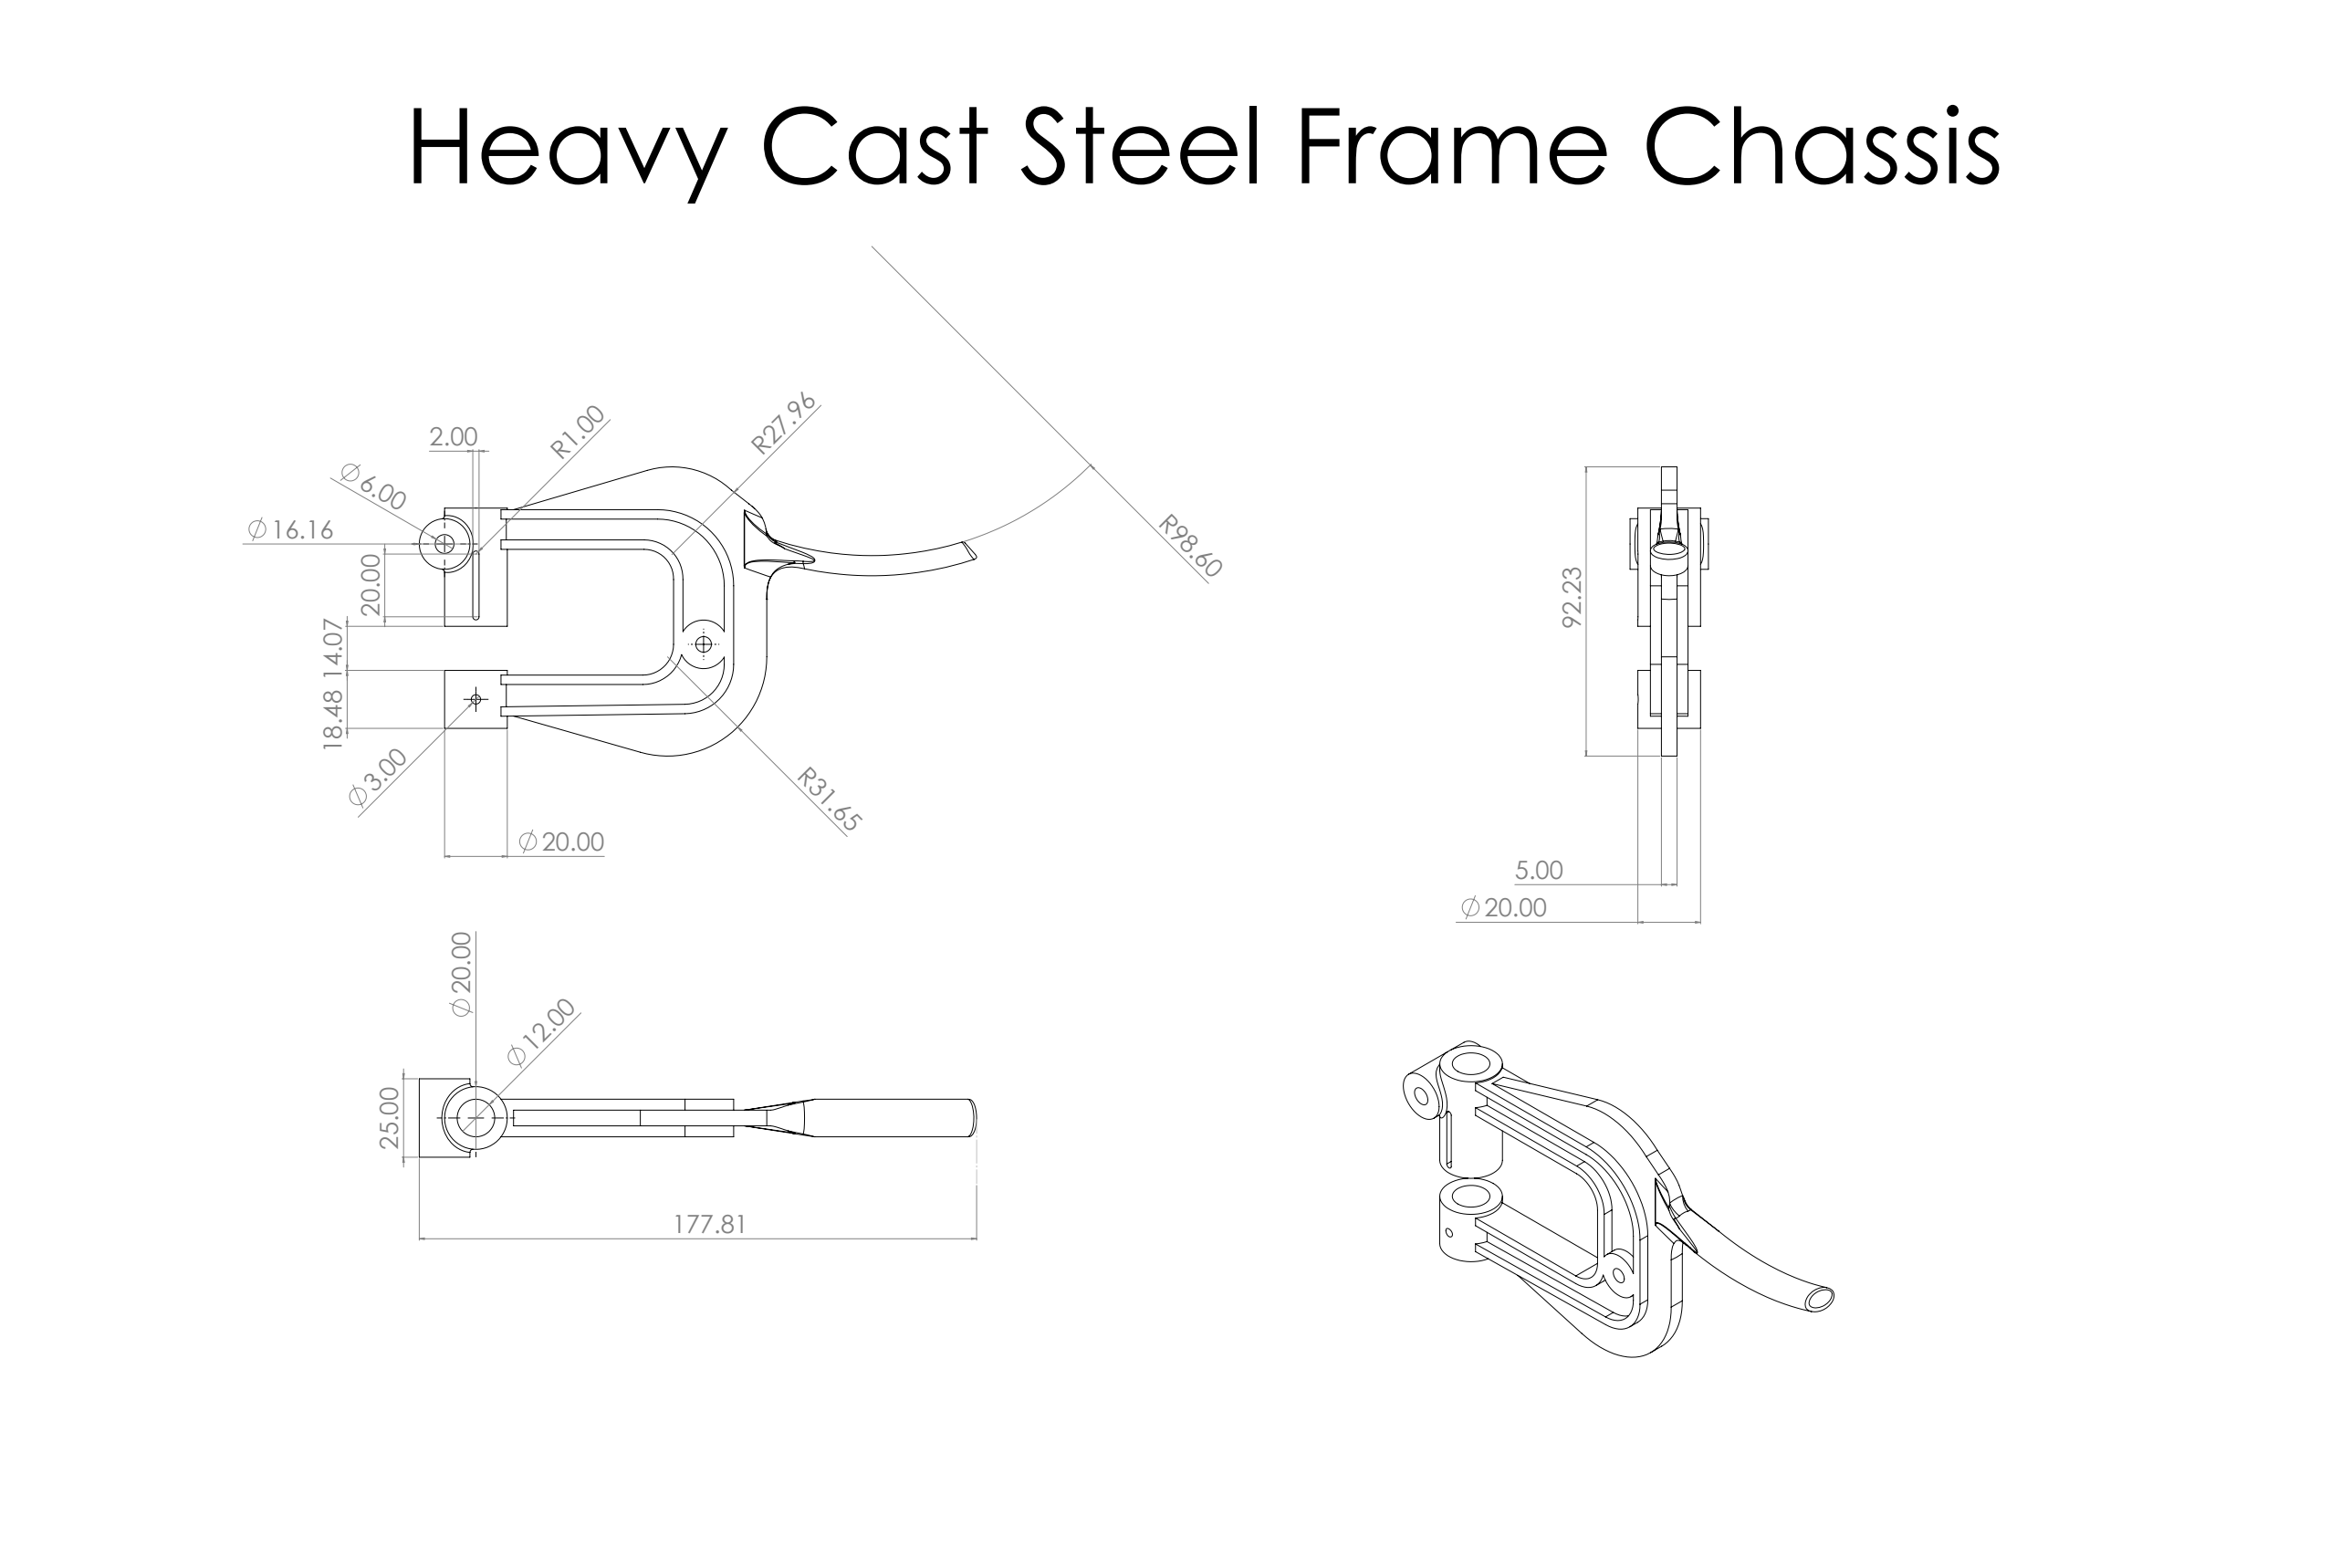
ISO-10303-21;
HEADER;
FILE_DESCRIPTION (('STEP AP214'),
    '1' );
FILE_NAME ('Heavy Cast Steel Frame Chassis.step',
    '2026-10-24T22:54:28',
    ( '' ),
    ( '' ),
    'SwSTEP 2.0',
    'SolidWorks 2025',
    '' );
FILE_SCHEMA (( 'AUTOMOTIVE_DESIGN' ));
ENDSEC;

DATA;
#3=CARTESIAN_POINT ( 'NONE',  ( 35.84136525188217348, -3.161327592290550825, 5.800309892887216989 ) ) ;
#5=CARTESIAN_POINT ( 'NONE',  ( 21.85645829928708039, 3.222455659797274663, 4.920547929353077166 ) ) ;
#7=VERTEX_POINT ( 'NONE', #10173 ) ;
#8=AXIS2_PLACEMENT_3D ( 'NONE', #5733, #22003, #2874 ) ;
#12=CARTESIAN_POINT ( 'NONE',  ( -71.92837670882107659, -20.78299143688747819, 38.00000000000000711 ) ) ;
#18=ORIENTED_EDGE ( 'NONE', *, *, #8070, .F. ) ;
#19=CARTESIAN_POINT ( 'NONE',  ( 21.85695786933250062, 3.618345527896555058, -4.619311229777957273 ) ) ;
#21=CARTESIAN_POINT ( 'NONE',  ( 21.85643539959774273, 10.54442680926682208, -0.8960936389291185300 ) ) ;
#28=CARTESIAN_POINT ( 'NONE',  ( 84.98726364908050357, 2.895996327189970021, 0.3032432708941606436 ) ) ;
#33=CARTESIAN_POINT ( 'NONE',  ( 15.61026443024166888, -3.737113800699907618, 2.632854455050967157 ) ) ;
#35=CARTESIAN_POINT ( 'NONE',  ( 34.13602976376383680, -3.136024335859604495, -5.534151046271431618 ) ) ;
#42=ORIENTED_EDGE ( 'NONE', *, *, #27798, .T. ) ;
#43=CARTESIAN_POINT ( 'NONE',  ( 37.00808470818950013, -3.245065655003315896, 5.947274188226997715 ) ) ;
#46=CARTESIAN_POINT ( 'NONE',  ( 87.70627581785944926, -2.246752060737267964, -2.595469083058261184 ) ) ;
#50=CARTESIAN_POINT ( 'NONE',  ( -70.92837670882107659, -23.80776546975053520, 0.000000000000000000 ) ) ;
#55=CARTESIAN_POINT ( 'NONE',  ( 24.04452188815935898, 3.332949059894338983, 3.268005727657652404 ) ) ;
#62=CARTESIAN_POINT ( 'NONE',  ( -71.02647992656017095, -45.61702805680359774, 6.000000000000006217 ) ) ;
#64=CARTESIAN_POINT ( 'NONE',  ( 17.44489164598297748, 8.923283497490654526, -2.906184072486747816 ) ) ;
#74=CARTESIAN_POINT ( 'NONE',  ( 27.93970670347097851, 2.313158937601060838, 2.612756796560576689 ) ) ;
#75=ADVANCED_FACE ( 'NONE', ( #21079, #21280 ), #17552, .T. ) ;
#78=CARTESIAN_POINT ( 'NONE',  ( 21.32819773538203734, -0.9284710762945487250, 4.803740791084685213 ) ) ;
#81=DIRECTION ( 'NONE',  ( -0.000000000000000000, -0.000000000000000000, -1.000000000000000000 ) ) ;
#86=CARTESIAN_POINT ( 'NONE',  ( 33.43749314767592296, -3.587398716883661631, -5.336340041065867901 ) ) ;
#90=CARTESIAN_POINT ( 'NONE',  ( 87.15505355144220800, 0.4610318193416703680, -5.246243280819175681 ) ) ;
#91=CARTESIAN_POINT ( 'NONE',  ( 23.06594672544511582, -8.086844732617873177, 2.500000000000001332 ) ) ;
#99=CARTESIAN_POINT ( 'NONE',  ( 8.290806648384990041, -33.63722727088462250, 6.000000000000001776 ) ) ;
#105=CARTESIAN_POINT ( 'NONE',  ( 24.41733686895641853, 3.169751135957838084, 3.243633740826553424 ) ) ;
#111=CARTESIAN_POINT ( 'NONE',  ( 23.09356329134889663, 0.3660385851480518205, 5.918987391801470821 ) ) ;
#117=EDGE_CURVE ( 'NONE', #23904, #23738, #12152, .T. ) ;
#120=CARTESIAN_POINT ( 'NONE',  ( 21.85643539959779602, 4.838159542671753854, -10.55000746994157979 ) ) ;
#122=CARTESIAN_POINT ( 'NONE',  ( -73.76321677170048474, 8.370041474172571938, 9.593160009199120708 ) ) ;
#123=CARTESIAN_POINT ( 'NONE',  ( 37.18496992949054913, -2.918767381260244154, 5.998331359843706245 ) ) ;
#127=CARTESIAN_POINT ( 'NONE',  ( -80.34626650618338317, 10.54088118240301775, -3.386839445737261034 ) ) ;
#128=CARTESIAN_POINT ( 'NONE',  ( 28.64320648638592104, -3.206774183960824587, -4.676863129512683237 ) ) ;
#129=CARTESIAN_POINT ( 'NONE',  ( 37.18689723876565978, -2.963747097358016003, -6.000011646107364705 ) ) ;
#130=CARTESIAN_POINT ( 'NONE',  ( -4.890026461918814071, -8.228598103685714525E-16, 6.000000000000000000 ) ) ;
#131=SHAPE_REPRESENTATION ( 'Heavy Cast Steel Frame Chassis', ( #30744 ), #7710 ) ;
#132=CARTESIAN_POINT ( 'NONE',  ( 21.48907598089328630, 5.617352746613489600, 3.514627525551620391 ) ) ;
#134=DIRECTION ( 'NONE',  ( 7.826543628040252284E-17, -1.000000000000000000, 0.000000000000000000 ) ) ;
#135=DIRECTION ( 'NONE',  ( 0.000000000000000000, 0.000000000000000000, -1.000000000000000000 ) ) ;
#137=CARTESIAN_POINT ( 'NONE',  ( 21.75356392267549310, 0.6818289899092313533, -8.045969637709488254 ) ) ;
#139=CARTESIAN_POINT ( 'NONE',  ( 32.63483486068848549, -3.790703822822770075, -4.926795467402606654 ) ) ;
#140=CARTESIAN_POINT ( 'NONE',  ( 25.39710067966193918, 2.282707499838438459, -4.082506721808119465 ) ) ;
#141=VERTEX_POINT ( 'NONE', #15910 ) ;
#144=CARTESIAN_POINT ( 'NONE',  ( 35.79015163951060430, -3.279169341215469213, 5.792316770070685017 ) ) ;
#146=CARTESIAN_POINT ( 'NONE',  ( 87.19696342060086636, -0.1553247823698818142, -5.755373573531420206 ) ) ;
#148=DIRECTION ( 'NONE',  ( 0.000000000000000000, 1.000000000000000000, 0.000000000000000000 ) ) ;
#150=CARTESIAN_POINT ( 'NONE',  ( 24.34527755301806451, 2.925195485058063927, 3.749207160500627634 ) ) ;
#163=CARTESIAN_POINT ( 'NONE',  ( -71.80187163192030653, -21.28714814314140469, 9.961904852117910991 ) ) ;
#165=CARTESIAN_POINT ( 'NONE',  ( 22.18865037645032601, 5.257466153314783064, -3.084642082178049360 ) ) ;
#173=CARTESIAN_POINT ( 'NONE',  ( -80.59724102483603758, -5.646254625739555166, -5.338710406051827562 ) ) ;
#176=CARTESIAN_POINT ( 'NONE',  ( 87.91343731185466481, -2.496140582104141359, -0.8634702502314072214 ) ) ;
#178=ORIENTED_EDGE ( 'NONE', *, *, #20772, .F. ) ;
#184=ORIENTED_EDGE ( 'NONE', *, *, #32019, .F. ) ;
#185=CARTESIAN_POINT ( 'NONE',  ( 35.86808974331964350, -2.088826501973227057, 5.804480896110276511 ) ) ;
#187=CARTESIAN_POINT ( 'NONE',  ( 87.73528170195316989, -0.1907079786014589107, -4.255344914058586170 ) ) ;
#191=DIRECTION ( 'NONE',  ( 1.000000000000000000, 0.000000000000000000, 0.000000000000000000 ) ) ;
#193=ORIENTED_EDGE ( 'NONE', *, *, #36678, .T. ) ;
#195=ORIENTED_EDGE ( 'NONE', *, *, #21675, .F. ) ;
#196=CARTESIAN_POINT ( 'NONE',  ( -72.40112826922974421, 5.951953399866846794, 9.891857903246553008 ) ) ;
#199=CARTESIAN_POINT ( 'NONE',  ( 21.94883752246645514, 5.596572238070317340, 3.078924485188955895 ) ) ;
#200=CARTESIAN_POINT ( 'NONE',  ( 25.44397797946202289, 1.878947632829091274, 4.230557655479292301 ) ) ;
#201=CARTESIAN_POINT ( 'NONE',  ( 27.23730700677205618, 2.045195204592743288, 3.801859922671973369 ) ) ;
#206=CARTESIAN_POINT ( 'NONE',  ( 85.45774792847294066, 2.367526054045318240, -2.907096912194419236 ) ) ;
#211=CARTESIAN_POINT ( 'NONE',  ( 23.22388547762907507, 3.341220446849921366, -3.796200845986580141 ) ) ;
#213=CARTESIAN_POINT ( 'NONE',  ( 21.85643539959774273, -10.14878426894149221, 9.991042268249278990 ) ) ;
#215=EDGE_CURVE ( 'NONE', #29684, #24175, #38700, .T. ) ;
#217=CARTESIAN_POINT ( 'NONE',  ( 88.07575545775937087, -0.5731442609823791390, 3.387043347726935050 ) ) ;
#218=VERTEX_POINT ( 'NONE', #31772 ) ;
#220=CARTESIAN_POINT ( 'NONE',  ( 14.77315594796442966, 13.19392823276588089, 2.499999999999996891 ) ) ;
#222=CARTESIAN_POINT ( 'NONE',  ( 26.28033317518049472, -2.868937434659071695, 4.308079602883402970 ) ) ;
#223=CARTESIAN_POINT ( 'NONE',  ( 33.68713372036676645, -3.101946962961664500, -5.464089962110080911 ) ) ;
#231=CARTESIAN_POINT ( 'NONE',  ( 31.99965334531182393, -3.138902966780172665, 5.200717837716557490 ) ) ;
#234=CARTESIAN_POINT ( 'NONE',  ( 20.91779494910925052, 4.579615739114438533, 2.660980063663031636 ) ) ;
#240=CARTESIAN_POINT ( 'NONE',  ( 87.52056228721085063, 0.05047505923521825727, -4.363535012332786955 ) ) ;
#248=CARTESIAN_POINT ( 'NONE',  ( 23.42285139394776650, 3.710806655037595547, 3.268438641518027765 ) ) ;
#250=EDGE_CURVE ( 'NONE', #11656, #22420, #37713, .T. ) ;
#255=CARTESIAN_POINT ( 'NONE',  ( -72.12756863348978698, -46.19478142241662511, 5.880635833492268816 ) ) ;
#257=CARTESIAN_POINT ( 'NONE',  ( 15.15950051851460145, 11.94258596470134215, -2.548869419651209611 ) ) ;
#262=VECTOR ( 'NONE', #5403, 1000.000000000000000 ) ;
#267=CARTESIAN_POINT ( 'NONE',  ( 17.02720445904918023, 12.19482440094239273, 2.500000000000000444 ) ) ;
#268=CARTESIAN_POINT ( 'NONE',  ( 31.47838864403340509, -3.170179483860372738, -5.357953045474171283 ) ) ;
#269=CARTESIAN_POINT ( 'NONE',  ( 0.000000000000000000, 0.000000000000000000, -2.500000000000000000 ) ) ;
#272=CIRCLE ( 'NONE', #25922, 10.00000000000000888 ) ;
#275=DIRECTION ( 'NONE',  ( -0.000000000000000000, -0.000000000000000000, 1.000000000000000000 ) ) ;
#277=CARTESIAN_POINT ( 'NONE',  ( 36.44537822125108306, -3.301946079842590365, -5.889618514196052423 ) ) ;
#280=CARTESIAN_POINT ( 'NONE',  ( 14.75904227071888108, -4.442295602227281037, -2.509903513768624972 ) ) ;
#286=CARTESIAN_POINT ( 'NONE',  ( 31.57897186779749887, -2.953369379551184171, 5.135060318927252787 ) ) ;
#290=B_SPLINE_CURVE_WITH_KNOTS ( 'NONE', 3,
 ( #31493, #201, #40324, #12739, #21411, #2492, #33986, #15014, #5760, #12117, #37245, #27977, #18300, #40525, #12334, #9037, #21615, #18711, #24908, #12538, #37442, #9240, #21817, #6170, #3114, #15632, #25110, #4461, #3513, #22239, #20275, #20084, #35749, #37849, #13504, #16983, #1375, #1769, #7523, #29956, #25318, #17182, #6583, #39002, #9654, #29158 ),
 .UNSPECIFIED., .F., .F.,
 ( 4, 2, 1, 1, 2, 2, 1, 1, 1, 2, 2, 2, 1, 1, 1, 2, 2, 1, 2, 2, 2, 2, 1, 1, 2, 2, 1, 2, 4 ),
 ( 0.1281237029900336166, 0.4747198910002122796, 0.4963821527508484044, 0.4990899354696787804, 0.4997668811493873875, 0.5004438268290958280, 0.5017977181885129312, 0.5072132836261800115, 0.5180444145015135060, 0.5613689380028479281, 0.6480179850055166613, 0.7346670320081853944, 0.7454981628835195551, 0.7482059456023534283, 0.7495598369617704204, 0.7498983098016249738, 0.7502367826414796381, 0.7509137283211883007, 0.7563292937588557141, 0.7779915555095239243, 0.7996538172601921346, 0.8104849481355265173, 0.8118388394949429543, 0.8121773123347969525, 0.8123465487547236741, 0.8125157851746505067, 0.8131927308543577260, 0.8159005135731869363, 0.8213160790108455789 ),
 .UNSPECIFIED. ) ;
#296=CARTESIAN_POINT ( 'NONE',  ( 23.06570227960076025, 3.126885040524279624, 4.061145912289076954 ) ) ;
#303=CARTESIAN_POINT ( 'NONE',  ( 23.43463349670878415, 3.790763441738238537, 3.110222249176512133 ) ) ;
#305=VECTOR ( 'NONE', #27454, 1000.000000000000000 ) ;
#311=CARTESIAN_POINT ( 'NONE',  ( 21.84880020533123002, 0.3448032378364013772, 8.036168467369821045 ) ) ;
#318=CARTESIAN_POINT ( 'NONE',  ( 22.67874324181232737, -4.030091496876125667, 7.802482278901700319 ) ) ;
#321=CARTESIAN_POINT ( 'NONE',  ( -75.51466614119452458, 10.05014096851642158, 8.892739820773797987 ) ) ;
#322=CARTESIAN_POINT ( 'NONE',  ( 21.96835285544658944, 0.2152711931543893065, -7.743667062754403752 ) ) ;
#323=ORIENTED_EDGE ( 'NONE', *, *, #28033, .F. ) ;
#327=FACE_OUTER_BOUND ( 'NONE', #20175, .T. ) ;
#328=CARTESIAN_POINT ( 'NONE',  ( 36.87196059928034941, -2.085890912122125407, -5.863601101037241747 ) ) ;
#338=CARTESIAN_POINT ( 'NONE',  ( 30.66378199172083896, -3.777849468416345502, -4.533872787636463286 ) ) ;
#343=DIRECTION ( 'NONE',  ( 0.7877517966954343809, -0.6159927814537400348, 0.000000000000000000 ) ) ;
#344=CARTESIAN_POINT ( 'NONE',  ( 88.38642666631945133, -2.374919807968325358, 0.2172961577596721761 ) ) ;
#348=CARTESIAN_POINT ( 'NONE',  ( 24.52494981597524770, 2.752700276650007716, 3.867455811991591386 ) ) ;
#364=ORIENTED_EDGE ( 'NONE', *, *, #24881, .F. ) ;
#370=CARTESIAN_POINT ( 'NONE',  ( 33.89815560913680059, -5.472034195326516581, 0.3552926572089393775 ) ) ;
#371=CARTESIAN_POINT ( 'NONE',  ( 22.19574982338894031, 5.228104102381771590, -3.102888934201143201 ) ) ;
#372=ORIENTED_EDGE ( 'NONE', *, *, #28540, .T. ) ;
#377=CARTESIAN_POINT ( 'NONE',  ( -81.11285676435983305, -5.649961960633484104, -4.124376956758348811 ) ) ;
#379=CARTESIAN_POINT ( 'NONE',  ( 29.20860690094596634, 2.240472738085125037, 1.050758983225395848 ) ) ;
#381=CARTESIAN_POINT ( 'NONE',  ( 87.68638643695580015, -2.222987235672965411, -2.753905389729575326 ) ) ;
#385=CARTESIAN_POINT ( 'NONE',  ( 24.97673583131591712, 3.396458356181121019, -1.647695864654638909 ) ) ;
#394=CARTESIAN_POINT ( 'NONE',  ( 21.25246165869702253, 3.318379160498120761, 3.523358653204108570 ) ) ;
#396=CARTESIAN_POINT ( 'NONE',  ( 86.26657670271889344, 1.459011185482768314, -4.895973709007312991 ) ) ;
#411=CARTESIAN_POINT ( 'NONE',  ( 23.70424450760806323, 1.818959193472196922, 4.681574839466135174 ) ) ;
#413=CIRCLE ( 'NONE', #30646, 12.38600677260393113 ) ;
#417=CARTESIAN_POINT ( 'NONE',  ( 85.87571968583984017, 1.898040338034475472, 4.108051227457266918 ) ) ;
#421=CARTESIAN_POINT ( 'NONE',  ( 22.18398091595247124, 4.302725770086238022, -3.814574538098304046 ) ) ;
#425=CARTESIAN_POINT ( 'NONE',  ( 21.85643539959775339, -6.841675198209371977, -12.88699694080538549 ) ) ;
#427=CARTESIAN_POINT ( 'NONE',  ( 53.63043182916395324, -5.819003020824450978, 6.000000000000000888 ) ) ;
#429=CARTESIAN_POINT ( 'NONE',  ( 85.06055580697953644, 2.762169973306998205, -2.784126402610546780 ) ) ;
#431=CARTESIAN_POINT ( 'NONE',  ( 14.69558838330753581, 12.33286846116140367, 2.499999999999996891 ) ) ;
#432=CARTESIAN_POINT ( 'NONE',  ( 14.98566736410303868, -6.090311521776418324, 2.529564007200721054 ) ) ;
#433=CARTESIAN_POINT ( 'NONE',  ( 33.62870426848748195, -1.228885055514358005, -5.454970633020429283 ) ) ;
#436=CARTESIAN_POINT ( 'NONE',  ( -74.18164544079856171, -2.036837289978346455, 10.73485733915913443 ) ) ;
#440=CARTESIAN_POINT ( 'NONE',  ( 33.46455574127770660, -3.089180930156425475, 5.429351285402141514 ) ) ;
#443=CARTESIAN_POINT ( 'NONE',  ( 36.13178710339454369, -1.532094116269871797, 5.644416983045655201 ) ) ;
#445=VECTOR ( 'NONE', #7320, 1000.000000000000000 ) ;
#448=VECTOR ( 'NONE', #1284, 1000.000000000000000 ) ;
#449=EDGE_CURVE ( 'NONE', #15211, #25138, #33471, .T. ) ;
#451=CARTESIAN_POINT ( 'NONE',  ( -80.82841455951717080, 11.46672392024627385, -1.471659699228122786 ) ) ;
#454=CARTESIAN_POINT ( 'NONE',  ( 8.290806648384990041, -10.90558813203967148, 6.000000000000000000 ) ) ;
#458=CARTESIAN_POINT ( 'NONE',  ( 22.03184786808944651, 5.415838924531075627, 3.191312399929147059 ) ) ;
#467=CARTESIAN_POINT ( 'NONE',  ( 19.96934150597399693, 6.745664378534328876, -3.285863046672279353 ) ) ;
#474=B_SPLINE_CURVE_WITH_KNOTS ( 'NONE', 3,
 ( #7514, #16768, #32255, #7119, #4054, #35545, #13493, #35147, #38993, #16570, #10598, #20074, #26464, #32851, #19480, #29350, #16376, #29150, #32651, #13092, #19682, #7315, #32054, #38600, #4451, #22979, #28950, #10792, #32446, #13285, #25857, #25653, #3860, #1170, #753, #1365 ),
 .UNSPECIFIED., .F., .F.,
 ( 4, 2, 2, 2, 2, 2, 2, 2, 2, 2, 2, 2, 2, 2, 2, 2, 2, 4 ),
 ( 0.07948797976893491601, 0.08078140541914788364, 0.08207483106936083739, 0.08336825671957380501, 0.08466168236978677264, 0.08595510801999974027, 0.08724853367021269401, 0.08854195932042566164, 0.08983538497063862927, 0.09112881062085158301, 0.09242223627106455064, 0.09371566192127751826, 0.09500908757149048589, 0.09630251322170343964, 0.09759593887191640726, 0.09888936452212937489, 0.09953607734723585176, 0.1001827901723423425 ),
 .UNSPECIFIED. ) ;
#478=CARTESIAN_POINT ( 'NONE',  ( 26.73479038929921359, 2.133517298515754668, 4.055905576634827092 ) ) ;
#490=CARTESIAN_POINT ( 'NONE',  ( 30.66842703005120185, 0.2949493320676357944, -4.962900476310909248 ) ) ;
#495=CARTESIAN_POINT ( 'NONE',  ( 22.49821043992852410, -9.358482552309803637, -2.500000000000000000 ) ) ;
#497=CARTESIAN_POINT ( 'NONE',  ( 21.89440445940014257, -12.98914838499760549, 2.499999999999999556 ) ) ;
#506=CARTESIAN_POINT ( 'NONE',  ( 30.31548945822549967, -3.037691172068890388, 4.938150023066174121 ) ) ;
#508=CARTESIAN_POINT ( 'NONE',  ( 21.85677098809243546, 3.668375465701176896, 4.582786065448858359 ) ) ;
#514=CARTESIAN_POINT ( 'NONE',  ( 24.40645114936911853, 3.164002126677583959, 3.269146773302918696 ) ) ;
#518=EDGE_LOOP ( 'NONE', ( #5397, #1910, #16353, #3651, #24693, #26966, #34035 ) ) ;
#520=CARTESIAN_POINT ( 'NONE',  ( 24.12512118317265930, 0.5285243960147255615, 5.092426130416875196 ) ) ;
#527=CARTESIAN_POINT ( 'NONE',  ( 24.99455384622441301, -2.608472216378299180, -6.027016329390949778 ) ) ;
#531=CARTESIAN_POINT ( 'NONE',  ( -72.64281072204887835, 6.529755665022496380, 9.854046603058758791 ) ) ;
#532=CARTESIAN_POINT ( 'NONE',  ( 20.40287464734031531, 10.75613383782063970, 2.500000000000000000 ) ) ;
#533=EDGE_LOOP ( 'NONE', ( #33702, #7118, #20763, #32067, #12346, #35016, #16297 ) ) ;
#537=CARTESIAN_POINT ( 'NONE',  ( 33.45805083109267741, -3.829395647111636602, -5.093820334410049000 ) ) ;
#538=CARTESIAN_POINT ( 'NONE',  ( 27.81621687972488033, 1.844493567162720948, -3.906584444767790654 ) ) ;
#540=CARTESIAN_POINT ( 'NONE',  ( 16.53760894254279634, 10.03315526601902619, 2.737223308667571242 ) ) ;
#541=CARTESIAN_POINT ( 'NONE',  ( 0.7201709579117279159, -51.60714625320436255, 6.000000000000000000 ) ) ;
#546=ADVANCED_FACE ( 'NONE', ( #1471 ), #22891, .T. ) ;
#548=CARTESIAN_POINT ( 'NONE',  ( 35.51269972589511070, -1.199312315519171834, -5.486990563529896114 ) ) ;
#553=CARTESIAN_POINT ( 'NONE',  ( 87.30284416890829391, -1.044652313481390760, -5.185858056390752147 ) ) ;
#556=ORIENTED_EDGE ( 'NONE', *, *, #29793, .F. ) ;
#557=CARTESIAN_POINT ( 'NONE',  ( 24.53045243809206255, 2.749270639064558708, 3.869256640630484689 ) ) ;
#559=DIRECTION ( 'NONE',  ( 0.000000000000000000, 1.000000000000000000, 0.000000000000000000 ) ) ;
#561=VERTEX_POINT ( 'NONE', #26383 ) ;
#564=ORIENTED_EDGE ( 'NONE', *, *, #36948, .F. ) ;
#575=CARTESIAN_POINT ( 'NONE',  ( 33.79783626363753513, -4.901490921675078383, -3.331131011404923736 ) ) ;
#576=CARTESIAN_POINT ( 'NONE',  ( 21.84698693888098120, 5.866571965567933589, -3.176918204583274452 ) ) ;
#582=CARTESIAN_POINT ( 'NONE',  ( -81.25348608327379907, -5.644728239778403989, -3.708980196009161290 ) ) ;
#584=FACE_OUTER_BOUND ( 'NONE', #9272, .T. ) ;
#586=CARTESIAN_POINT ( 'NONE',  ( 87.11462257552980759, -1.147413441766115039, -5.140310012396687611 ) ) ;
#596=CARTESIAN_POINT ( 'NONE',  ( 36.91143285253476591, -2.638629310656217530, 5.967319821651744682 ) ) ;
#599=CARTESIAN_POINT ( 'NONE',  ( 87.87162303905448368, -0.3438530395839958231, 3.959040383187740542 ) ) ;
#600=ORIENTED_EDGE ( 'NONE', *, *, #11873, .T. ) ;
#601=CARTESIAN_POINT ( 'NONE',  ( 14.61802081865034530, -4.584627643820613052, 2.500000000000000000 ) ) ;
#602=CARTESIAN_POINT ( 'NONE',  ( -69.43819311319896315, -46.91958326716831351, 9.888363374916961490 ) ) ;
#606=CARTESIAN_POINT ( 'NONE',  ( -74.34312302644391934, -4.176925768793524618, 9.403213700939037523 ) ) ;
#610=( BOUNDED_SURFACE ( )  B_SPLINE_SURFACE ( 3, 2, ( 
 ( #27283, #33689, #29569 ),
 ( #11415, #17802, #7936 ),
 ( #2192, #24196, #39423 ),
 ( #20486, #1385, #20907 ),
 ( #33070, #11616, #10817 ),
 ( #23392, #32870, #8123 ),
 ( #23982, #14709, #17593 ),
 ( #36357, #35958, #20286 ),
 ( #4659, #14512, #17387 ),
 ( #26688, #11213, #36755 ),
 ( #1994, #8331, #33493 ),
 ( #17195, #39221, #4853 ),
 ( #39849, #30387, #30172 ),
 ( #1782, #29763, #21121 ),
 ( #1577, #11012, #14109 ),
 ( #23593, #33279, #14311 ),
 ( #26880, #23778, #20696 ),
 ( #5059, #27086, #39632 ) ),
 .UNSPECIFIED., .F., .F., .T. ) 
 B_SPLINE_SURFACE_WITH_KNOTS ( ( 4, 2, 2, 2, 2, 2, 2, 2, 4 ),
 ( 3, 3 ),
 ( 0.000000000000000000, 9.251198296377863305E-05, 0.0001850239659275572661, 0.0003700479318551145322, 0.0005550718977826718525, 0.0006475838807464504585, 0.0006938398722283398157, 0.0007169678679692844401, 0.0007400958637102290644 ),
 ( 0.000000000000000000, 1.000000000000000000 ),
 .UNSPECIFIED. ) 
 GEOMETRIC_REPRESENTATION_ITEM ( )  RATIONAL_B_SPLINE_SURFACE ( (
 ( 1.000000000000000000, 0.9970051441236916778, 1.000000000000000000),
 ( 1.000000000000000000, 0.9970374898934499797, 1.000000000000000000),
 ( 1.000000000000000000, 0.9972378587227352931, 1.000000000000000000),
 ( 1.000000000000000000, 0.9976285232392927416, 1.000000000000000000),
 ( 1.000000000000000000, 0.9978377992949450936, 1.000000000000000000),
 ( 1.000000000000000000, 0.9984458866281191725, 1.000000000000000000),
 ( 1.000000000000000000, 0.9988290234017360714, 1.000000000000000000),
 ( 1.000000000000000000, 0.9994403397046758286, 1.000000000000000000),
 ( 1.000000000000000000, 0.9996688303162680755, 1.000000000000000000),
 ( 1.000000000000000000, 0.9998817225008336251, 1.000000000000000000),
 ( 1.000000000000000000, 0.9999314634536117241, 1.000000000000000000),
 ( 1.000000000000000000, 0.9999767510700310336, 1.000000000000000000),
 ( 1.000000000000000000, 0.9999869665867011648, 1.000000000000000000),
 ( 1.000000000000000000, 0.9999959687235325800, 1.000000000000000000),
 ( 1.000000000000000000, 0.9999979380867456413, 1.000000000000000000),
 ( 1.000000000000000000, 0.9999998520708384131, 1.000000000000000000),
 ( 1.000000000000000000, 0.9999995175495077770, 1.000000000000000000),
 ( 1.000000000000000000, 0.9999995739621224677, 1.000000000000000000) ) ) 
 REPRESENTATION_ITEM ( '' )  SURFACE ( )  );
#613=CARTESIAN_POINT ( 'NONE',  ( 25.37055851336592838, 2.296153116583149689, 4.076656671453694258 ) ) ;
#615=VERTEX_POINT ( 'NONE', #39728 ) ;
#622=CARTESIAN_POINT ( 'NONE',  ( 24.35698045111728760, 2.890171444508740084, -3.780454612355467425 ) ) ;
#623=EDGE_LOOP ( 'NONE', ( #17672, #40325, #5137, #17035, #31443 ) ) ;
#624=EDGE_CURVE ( 'NONE', #9599, #28854, #17535, .T. ) ;
#627=CARTESIAN_POINT ( 'NONE',  ( 21.85643539959780313, -7.722266916079949972, 9.821539774841749448 ) ) ;
#628=EDGE_CURVE ( 'NONE', #3707, #4251, #20578, .T. ) ;
#629=CARTESIAN_POINT ( 'NONE',  ( 21.83106932671409339, 5.061056560966107121, -3.908462188292611383 ) ) ;
#633=CARTESIAN_POINT ( 'NONE',  ( 84.79809517660038409, 3.058972130929652256, -0.4747855469284483210 ) ) ;
#638=CARTESIAN_POINT ( 'NONE',  ( 14.78598032573992072, -5.967041118660810106, 2.514107848754160823 ) ) ;
#639=CARTESIAN_POINT ( 'NONE',  ( 37.03752275446304054, -3.000583964048129104, 5.986999200343480432 ) ) ;
#643=CARTESIAN_POINT ( 'NONE',  ( 32.78033889701190873, -0.9298251412089901802, -5.322562699007520770 ) ) ;
#646=CARTESIAN_POINT ( 'NONE',  ( -73.95647868120518353, -1.676906216185754417, 10.78713444449159553 ) ) ;
#649=CARTESIAN_POINT ( 'NONE',  ( 28.64411823881500041, -3.206366735157959003, 4.677005430563262678 ) ) ;
#652=CARTESIAN_POINT ( 'NONE',  ( 29.48743188508317914, 1.218356524489477177, 4.224828210317064681 ) ) ;
#670=CARTESIAN_POINT ( 'NONE',  ( 17.70185162816926194, 8.503195812862719194, -2.969200086112000037 ) ) ;
#675=CARTESIAN_POINT ( 'NONE',  ( 24.20710697820493706, 2.664667655643908617, -3.984502513680244107 ) ) ;
#678=CARTESIAN_POINT ( 'NONE',  ( 15.85384028848737792, 7.981620951995479274, 3.484773800359201701 ) ) ;
#679=CARTESIAN_POINT ( 'NONE',  ( 29.75545004716739683, -3.157578436209982353, 4.923334784591472335 ) ) ;
#684=ADVANCED_FACE ( 'NONE', ( #21823 ), #31095, .T. ) ;
#689=CARTESIAN_POINT ( 'NONE',  ( 35.33682791254538103, -3.445753084594619153, -5.710983022405980769 ) ) ;
#696=CARTESIAN_POINT ( 'NONE',  ( 21.86866938121569603, -13.71747586059087709, 2.499999999999999112 ) ) ;
#698=CARTESIAN_POINT ( 'NONE',  ( 31.82733904959990312, -2.965273931086898962, 5.173824024430509816 ) ) ;
#700=DIRECTION ( 'NONE',  ( 1.000000000000000000, 8.966158204770716457E-16, 0.000000000000000000 ) ) ;
#705=CARTESIAN_POINT ( 'NONE',  ( 23.67813930011643464, 3.094851216756080436, 3.803410633069329361 ) ) ;
#707=LINE ( 'NONE', #9951, #21414 ) ;
#709=ORIENTED_EDGE ( 'NONE', *, *, #911, .F. ) ;
#715=CARTESIAN_POINT ( 'NONE',  ( 22.31539195409567355, 0.2712039597043285344, 7.065721357752317466 ) ) ;
#722=CARTESIAN_POINT ( 'NONE',  ( 25.51676067120702740, -4.685157242005201006, -0.9133679171623337867 ) ) ;
#724=ORIENTED_EDGE ( 'NONE', *, *, #737, .F. ) ;
#725=CARTESIAN_POINT ( 'NONE',  ( -74.08736391206848282, -1.888185831823766314, 10.75649061611074764 ) ) ;
#731=CARTESIAN_POINT ( 'NONE',  ( 32.01241132122780897, -3.694368527175160288, -4.883964182103501805 ) ) ;
#732=CARTESIAN_POINT ( 'NONE',  ( 35.73033373643165334, -1.304506732970901028, -5.538159404137515729 ) ) ;
#734=CARTESIAN_POINT ( 'NONE',  ( 19.77034930170943738, 6.504725764514479813, 3.292039174873226060 ) ) ;
#737=EDGE_CURVE ( 'NONE', #21561, #15320, #31300, .T. ) ;
#741=CARTESIAN_POINT ( 'NONE',  ( 21.92110598244980935, 0.6179470853736169778, -7.522509096894697045 ) ) ;
#742=CARTESIAN_POINT ( 'NONE',  ( 33.54628729347086846, -0.3308921759967717868, -5.040328079186997101 ) ) ;
#749=CARTESIAN_POINT ( 'NONE',  ( 85.85763368383675243, 1.114829962406831410, -5.799110970849834068 ) ) ;
#753=CARTESIAN_POINT ( 'NONE',  ( -72.84815947045235873, 2.644610850572383320, -10.96147798754375202 ) ) ;
#764=LINE ( 'NONE', #38611, #21033 ) ;
#766=EDGE_CURVE ( 'NONE', #17308, #38743, #18493, .T. ) ;
#770=CARTESIAN_POINT ( 'NONE',  ( 21.85643539959776760, -0.9922589305345951294, -16.01828770219436393 ) ) ;
#771=CARTESIAN_POINT ( 'NONE',  ( 24.04398671587223291, 3.332573078807886446, -3.269442169970088408 ) ) ;
#778=CARTESIAN_POINT ( 'NONE',  ( -74.68647436060540201, -2.705062680926989316, -10.58800659810225220 ) ) ;
#780=DIRECTION ( 'NONE',  ( -0.000000000000000000, -0.000000000000000000, -1.000000000000000000 ) ) ;
#783=CARTESIAN_POINT ( 'NONE',  ( 84.50243033367722489, 2.523019330700893903, 3.504063919878146027 ) ) ;
#784=DIRECTION ( 'NONE',  ( 0.000000000000000000, -1.000000000000000000, 0.000000000000000000 ) ) ;
#787=CARTESIAN_POINT ( 'NONE',  ( 32.07395207475902055, -0.6787058776523876569, 5.212313951365143083 ) ) ;
#792=CARTESIAN_POINT ( 'NONE',  ( 25.29738944813237467, 1.738831336413337203, 4.154667461693681396 ) ) ;
#795=CARTESIAN_POINT ( 'NONE',  ( 87.05466826895010968, 0.5737893332097195875, -5.097061431219924721 ) ) ;
#802=CARTESIAN_POINT ( 'NONE',  ( 0.000000000000000000, 10.37661300689600097, 6.000000000000000000 ) ) ;
#804=CARTESIAN_POINT ( 'NONE',  ( -73.13398320254746920, 7.456860240122096251, 9.756630903624417428 ) ) ;
#805=AXIS2_PLACEMENT_3D ( 'NONE', #17898, #40334, #36246 ) ;
#812=CARTESIAN_POINT ( 'NONE',  ( 22.74182454973798073, 2.295841465708973850, 4.886361631232980507 ) ) ;
#824=CARTESIAN_POINT ( 'NONE',  ( 22.00320784554085662, 4.481518016395985349, -3.871533879853490845 ) ) ;
#827=CARTESIAN_POINT ( 'NONE',  ( 21.85643539959772497, -13.01485165473748573, 3.478087416278500932 ) ) ;
#828=CARTESIAN_POINT ( 'NONE',  ( 21.86697325015170890, 4.291357277895272659, 2.119771864001716910 ) ) ;
#829=ORIENTED_EDGE ( 'NONE', *, *, #15859, .F. ) ;
#832=CARTESIAN_POINT ( 'NONE',  ( 87.01296019436635731, 0.4868102506410553754, -5.723292304581113044 ) ) ;
#833=VERTEX_POINT ( 'NONE', #26333 ) ;
#836=CARTESIAN_POINT ( 'NONE',  ( 14.77222812468937363, 12.33286846116137347, 2.511961485181785747 ) ) ;
#837=CARTESIAN_POINT ( 'NONE',  ( 35.94401475533869927, -2.118279520774572600, 5.816330830489228276 ) ) ;
#839=CARTESIAN_POINT ( 'NONE',  ( 36.64572461763481215, -2.462317435528831755, -5.925849625417530575 ) ) ;
#841=CARTESIAN_POINT ( 'NONE',  ( 84.16515158064987645, 2.938904301663770369, -1.440371321264852122 ) ) ;
#847=CARTESIAN_POINT ( 'NONE',  ( 28.41948456483106256, -4.023518219021338993, 4.166478601093604794 ) ) ;
#850=CARTESIAN_POINT ( 'NONE',  ( 21.73904118813925379, 4.235523336977800035, 2.801162882007421029 ) ) ;
#851=( BOUNDED_CURVE ( )  B_SPLINE_CURVE ( 3, ( #21836, #427, #38077, #9879 ),
 .UNSPECIFIED., .F., .F. ) 
 B_SPLINE_CURVE_WITH_KNOTS ( ( 4, 4 ),
 ( 0.3200567789910438443, 0.9848974682458135899 ),
 .UNSPECIFIED. ) 
 CURVE ( )  GEOMETRIC_REPRESENTATION_ITEM ( )  RATIONAL_B_SPLINE_CURVE ( ( 0.9715283101266052324, 0.9610937201533095164, 0.9699355995880819536, 0.9980539484309227660 ) ) 
 REPRESENTATION_ITEM ( '' )  );
#855=CARTESIAN_POINT ( 'NONE',  ( 86.80810971983586910, -1.084991844513179204, 5.287006610588839806 ) ) ;
#858=CARTESIAN_POINT ( 'NONE',  ( -12.99139449055068596, 10.37661300689600097, -6.000000000000000000 ) ) ;
#859=DIRECTION ( 'NONE',  ( 0.000000000000000000, 0.000000000000000000, -1.000000000000000000 ) ) ;
#864=CARTESIAN_POINT ( 'NONE',  ( 21.74862740251015580, 5.983917815004713425, 3.320825558061557103 ) ) ;
#868=ORIENTED_EDGE ( 'NONE', *, *, #20775, .T. ) ;
#878=CARTESIAN_POINT ( 'NONE',  ( 22.90829551299158240, 3.597247491013313425, -3.781791572659710443 ) ) ;
#882=CARTESIAN_POINT ( 'NONE',  ( 28.73718198699435433, 0.3327373454474676917, -5.564570571917969666 ) ) ;
#884=FACE_OUTER_BOUND ( 'NONE', #21957, .T. ) ;
#887=CARTESIAN_POINT ( 'NONE',  ( 37.06596529586517619, -2.656456832825214498, -5.990207561623762444 ) ) ;
#890=CARTESIAN_POINT ( 'NONE',  ( 4.938390203311415748E-15, -42.37473357531882101, 6.000000000000000000 ) ) ;
#891=CARTESIAN_POINT ( 'NONE',  ( 22.05611991773309555, -11.37525250134437016, -2.500000000000000000 ) ) ;
#893=FACE_OUTER_BOUND ( 'NONE', #28439, .T. ) ;
#895=CARTESIAN_POINT ( 'NONE',  ( 33.45000747465049074, -3.250805911200664866, 5.427080676543816651 ) ) ;
#903=CARTESIAN_POINT ( 'NONE',  ( 23.43999384881404069, 3.253530542321768859, 3.760554638137439287 ) ) ;
#909=CARTESIAN_POINT ( 'NONE',  ( 22.18569188669614434, 5.274102994114218568, 3.071853425151234607 ) ) ;
#911=EDGE_CURVE ( 'NONE', #4342, #17714, #30011, .T. ) ;
#917=ORIENTED_EDGE ( 'NONE', *, *, #25735, .T. ) ;
#919=CARTESIAN_POINT ( 'NONE',  ( 27.39979242429538786, 1.046165008357551329, 4.482586396029306641 ) ) ;
#920=CARTESIAN_POINT ( 'NONE',  ( 14.77222415230653318, -4.492512959436772313, -2.511960865195376424 ) ) ;
#928=CARTESIAN_POINT ( 'NONE',  ( 23.99854160108877110, 3.116918725036224025, -4.608611027060286247 ) ) ;
#931=CARTESIAN_POINT ( 'NONE',  ( -79.85848762145901958, -6.650571597313232886, 4.518583439907962074 ) ) ;
#932=FACE_OUTER_BOUND ( 'NONE', #28199, .T. ) ;
#936=CARTESIAN_POINT ( 'NONE',  ( 37.00823095920353722, -3.245628662103481776, -5.947143878220320978 ) ) ;
#937=DIRECTION ( 'NONE',  ( 1.165409145176970240E-16, -1.000000000000000000, 0.000000000000000000 ) ) ;
#938=CARTESIAN_POINT ( 'NONE',  ( -4.890026461918814071, -8.228598103685714525E-16, -6.000000000000000000 ) ) ;
#947=CARTESIAN_POINT ( 'NONE',  ( 24.52892761326155835, 0.9676208338128078346, -4.779935416704812035 ) ) ;
#948=CARTESIAN_POINT ( 'NONE',  ( 36.44367235456785892, -1.740113775189354506, -5.733408591441955693 ) ) ;
#949=LINE ( 'NONE', #28530, #9128 ) ;
#950=ORIENTED_EDGE ( 'NONE', *, *, #18826, .T. ) ;
#954=CARTESIAN_POINT ( 'NONE',  ( 84.14932678670007249, 2.958124188176427083, -1.306863746360770184 ) ) ;
#975=CARTESIAN_POINT ( 'NONE',  ( 21.85643539959777826, -5.920441741711214512, 15.33489310402742234 ) ) ;
#977=CARTESIAN_POINT ( 'NONE',  ( 24.75846013112230537, 3.019289815473042093, -3.350249464038115743 ) ) ;
#984=CARTESIAN_POINT ( 'NONE',  ( -72.89865255728501836, 3.415802629356370801, -10.95661767982553414 ) ) ;
#988=CARTESIAN_POINT ( 'NONE',  ( 86.62140889132389532, -0.8164050916001737157, 5.580443680875508683 ) ) ;
#992=EDGE_CURVE ( 'NONE', #8047, #13934, #24934, .T. ) ;
#994=CARTESIAN_POINT ( 'NONE',  ( 16.66444302124740418, 9.373703860693387568, -2.807287383179874585 ) ) ;
#996=CARTESIAN_POINT ( 'NONE',  ( -70.92837670882107659, -23.80776546975053165, 0.000000000000000000 ) ) ;
#999=CARTESIAN_POINT ( 'NONE',  ( 35.45370152372439065, -1.914224272725399745, 5.739805592425503811 ) ) ;
#1004=CARTESIAN_POINT ( 'NONE',  ( 88.13490256179494509, -0.6395810955261213016, -2.488665338685403849 ) ) ;
#1009=CARTESIAN_POINT ( 'NONE',  ( 88.14657295384911606, -0.6526898337915518766, -2.384354617864239856 ) ) ;
#1014=CARTESIAN_POINT ( 'NONE',  ( -72.53312289749355557, -1.419736944430859849, 9.872087320082300721 ) ) ;
#1016=EDGE_CURVE ( 'NONE', #7067, #19825, #28357, .T. ) ;
#1019=CARTESIAN_POINT ( 'NONE',  ( 22.80245925209617397, 1.698177091178224130, 5.311506672424976649 ) ) ;
#1021=ORIENTED_EDGE ( 'NONE', *, *, #22573, .F. ) ;
#1024=CARTESIAN_POINT ( 'NONE',  ( 86.45541607342296686, 1.246897841450794298, 4.891341099398129444 ) ) ;
#1028=CARTESIAN_POINT ( 'NONE',  ( 22.79970795871216183, 3.574398117813434528, -3.863569992082448668 ) ) ;
#1029=ORIENTED_EDGE ( 'NONE', *, *, #23203, .T. ) ;
#1034=CARTESIAN_POINT ( 'NONE',  ( 21.85643539959776049, -10.96491163060450802, -3.419414754301954851 ) ) ;
#1035=AXIS2_PLACEMENT_3D ( 'NONE', #17718, #30302, #39763 ) ;
#1037=CARTESIAN_POINT ( 'NONE',  ( 20.16883043526225805, 11.76570021213147932, -3.257865388785521787 ) ) ;
#1040=CARTESIAN_POINT ( 'NONE',  ( 88.05979627311084812, -0.5552181473167765446, -3.927858985986737661 ) ) ;
#1042=CARTESIAN_POINT ( 'NONE',  ( 14.67409684075444609, -5.611220017537962512, 2.496645725009577266 ) ) ;
#1043=CARTESIAN_POINT ( 'NONE',  ( 31.19756578357611332, -3.761128863170072112, 4.642324994556521922 ) ) ;
#1044=CARTESIAN_POINT ( 'NONE',  ( 33.95934880225217967, -3.272301304683462142, -5.506575709182617295 ) ) ;
#1045=CARTESIAN_POINT ( 'NONE',  ( 33.46266692859374103, -3.084164941913754898, -5.429056490501709575 ) ) ;
#1047=CARTESIAN_POINT ( 'NONE',  ( 84.10804491527638049, 3.008217574094829594, -0.3805531846457105294 ) ) ;
#1054=CARTESIAN_POINT ( 'NONE',  ( 30.73573697167703855, -3.645023302247464070, 4.721775058918869838 ) ) ;
#1057=CARTESIAN_POINT ( 'NONE',  ( 36.71904603859049843, -3.458174413421041038, 5.860823370863815995 ) ) ;
#1061=CARTESIAN_POINT ( 'NONE',  ( 87.17674554246272578, -1.585054265969757958, 4.548888058249088040 ) ) ;
#1070=CARTESIAN_POINT ( 'NONE',  ( 8.290806648384990041, 0.000000000000000000, 6.000000000000000000 ) ) ;
#1071=EDGE_LOOP ( 'NONE', ( #24906, #31817, #31731, #18549, #40271, #17938, #12859, #23182 ) ) ;
#1089=CARTESIAN_POINT ( 'NONE',  ( 28.53445731760455573, 0.6922391713037714389, -5.301755952056612209 ) ) ;
#1092=CARTESIAN_POINT ( 'NONE',  ( -80.24641704084613991, -5.629453946137603637, -6.035434990652555953 ) ) ;
#1097=CARTESIAN_POINT ( 'NONE',  ( 36.02633504632637340, -1.730128226848125950, -5.776816043798858047 ) ) ;
#1105=CARTESIAN_POINT ( 'NONE',  ( 21.85643539959776760, -15.11427361947482062, -2.500000000000000000 ) ) ;
#1107=CARTESIAN_POINT ( 'NONE',  ( 31.81222844470352840, -2.964472128955970121, 5.171465649085067895 ) ) ;
#1110=CARTESIAN_POINT ( 'NONE',  ( 36.54090531688899546, -2.167697392235706566, 5.903356262276473032 ) ) ;
#1115=CARTESIAN_POINT ( 'NONE',  ( -18.27651686900387418, -64.04014080848075707, 2.500000000000000000 ) ) ;
#1116=CARTESIAN_POINT ( 'NONE',  ( 30.87880611384830587, -3.486100459600208090, 4.898406253664910892 ) ) ;
#1120=ADVANCED_FACE ( 'NONE', ( #27731 ), #11866, .T. ) ;
#1122=CARTESIAN_POINT ( 'NONE',  ( -0.000000000000000000, 10.37661300689600097, -2.500000000000000000 ) ) ;
#1124=CARTESIAN_POINT ( 'NONE',  ( 24.75831320048713735, 3.019228828327055858, 3.350538031934082284 ) ) ;
#1127=CARTESIAN_POINT ( 'NONE',  ( 25.22329213065313169, -5.090999687581535760, -2.500000000044154014 ) ) ;
#1130=CARTESIAN_POINT ( 'NONE',  ( 24.12373500254816605, 0.4971700199039688073, 5.094523214884540074 ) ) ;
#1140=CARTESIAN_POINT ( 'NONE',  ( 22.31759743831440090, 6.226164879696757026, 1.431367841762869686 ) ) ;
#1143=CARTESIAN_POINT ( 'NONE',  ( -76.06876986340937208, -4.053555619469175753, 8.607033718690072277 ) ) ;
#1144=CARTESIAN_POINT ( 'NONE',  ( -12.99139449055068241, 13.37661300689600097, 6.000000000000000000 ) ) ;
#1145=ADVANCED_FACE ( 'NONE', ( #40479 ), #21777, .F. ) ;
#1150=CARTESIAN_POINT ( 'NONE',  ( 37.01014894729547677, -2.248942906826801202, -5.913016239383465766 ) ) ;
#1151=CARTESIAN_POINT ( 'NONE',  ( 30.76700883330015301, -3.320931493643032084, -4.963836536440328295 ) ) ;
#1157=EDGE_CURVE ( 'NONE', #22987, #8010, #30329, .T. ) ;
#1158=VECTOR ( 'NONE', #8175, 1000.000000000000000 ) ;
#1160=CARTESIAN_POINT ( 'NONE',  ( 22.83119761409040294, 1.181603121085857078, -5.687369041816118909 ) ) ;
#1162=ORIENTED_EDGE ( 'NONE', *, *, #19712, .F. ) ;
#1163=VECTOR ( 'NONE', #24219, 1000.000000000000000 ) ;
#1165=VECTOR ( 'NONE', #34063, 1000.000000000000000 ) ;
#1168=CARTESIAN_POINT ( 'NONE',  ( 84.24490603200722205, 3.007448030680667017, 1.128815683486722454 ) ) ;
#1170=CARTESIAN_POINT ( 'NONE',  ( -72.85671063792464963, 2.859724406437386346, -10.96068470457861999 ) ) ;
#1176=ORIENTED_EDGE ( 'NONE', *, *, #3818, .T. ) ;
#1179=CARTESIAN_POINT ( 'NONE',  ( 33.60131552963068913, -4.188911086009777129, 4.688672432858080441 ) ) ;
#1181=CARTESIAN_POINT ( 'NONE',  ( 24.18364339310534916, 2.677224417268836199, 3.980840453756503194 ) ) ;
#1183=CYLINDRICAL_SURFACE ( 'NONE', #24845, 12.80480339192541628 ) ;
#1185=CARTESIAN_POINT ( 'NONE',  ( 21.85643539959778181, 2.657715471900086612, -15.25567151318962367 ) ) ;
#1189=CIRCLE ( 'NONE', #4471, 10.00000000000000533 ) ;
#1193=CARTESIAN_POINT ( 'NONE',  ( -75.00170219041523012, -3.073105394106712129, -9.174977135382700766 ) ) ;
#1210=CARTESIAN_POINT ( 'NONE',  ( 34.33337444863689569, -1.484546483778259818, 5.564951457145235203 ) ) ;
#1212=CARTESIAN_POINT ( 'NONE',  ( 85.85116863490735284, 1.861966474136578231, -4.950709030323501736 ) ) ;
#1227=CARTESIAN_POINT ( 'NONE',  ( 25.36303923114378733, 1.426800422063377427, 4.397790789347460816 ) ) ;
#1228=ORIENTED_EDGE ( 'NONE', *, *, #3853, .F. ) ;
#1230=CIRCLE ( 'NONE', #24210, 10.00000000000000888 ) ;
#1236=CARTESIAN_POINT ( 'NONE',  ( 23.41943767133188814, 3.656341323882381200, -3.349654434191691621 ) ) ;
#1239=CARTESIAN_POINT ( 'NONE',  ( 22.37806265499392566, 3.168015787195890720, 7.828147373443384183 ) ) ;
#1240=CARTESIAN_POINT ( 'NONE',  ( 21.86870537176919527, 3.698784010464675198, 3.388912068464415395 ) ) ;
#1243=CARTESIAN_POINT ( 'NONE',  ( 84.68420644151177612, 2.996072101527111453, 1.894685230139086851 ) ) ;
#1247=CARTESIAN_POINT ( 'NONE',  ( 31.01275874060653592, -3.765090545890084961, 4.604780786014718963 ) ) ;
#1248=CARTESIAN_POINT ( 'NONE',  ( 33.12677655050840997, -3.093949257744326609, -5.376632673462000689 ) ) ;
#1250=CARTESIAN_POINT ( 'NONE',  ( 36.63309929816978894, -3.078772421412805382, -5.923879138970663760 ) ) ;
#1252=CARTESIAN_POINT ( 'NONE',  ( 84.43366413210182486, 2.606424049041346169, 3.204991622768011084 ) ) ;
#1259=ORIENTED_EDGE ( 'NONE', *, *, #27979, .T. ) ;
#1260=CARTESIAN_POINT ( 'NONE',  ( 29.48809767354670086, 1.219317615460245641, 4.222743620664576092 ) ) ;
#1261=CARTESIAN_POINT ( 'NONE',  ( 15.55633224523761982, -3.531369950178294914, 2.634339896823157723 ) ) ;
#1263=CARTESIAN_POINT ( 'NONE',  ( 87.90175190873620181, -2.482191174542180523, 0.8726593636648759533 ) ) ;
#1270=CARTESIAN_POINT ( 'NONE',  ( 22.92431439707159058, 4.119491578302444168, 3.288696840953844625 ) ) ;
#1278=CARTESIAN_POINT ( 'NONE',  ( 22.07118065842499277, 4.795981446113927404, -3.651139553905330182 ) ) ;
#1281=CARTESIAN_POINT ( 'NONE',  ( 22.04371986193802968, 2.335811073793032211, -5.477320531203638154 ) ) ;
#1282=CARTESIAN_POINT ( 'NONE',  ( -70.92837670881976919, 0.2170085631237942680, 10.00000000000113154 ) ) ;
#1284=DIRECTION ( 'NONE',  ( -1.000000000000000000, -1.165409145176970240E-16, 0.000000000000000000 ) ) ;
#1290=CARTESIAN_POINT ( 'NONE',  ( 31.58133870531054654, -3.380569343585269504, 5.164673136779329710 ) ) ;
#1292=CARTESIAN_POINT ( 'NONE',  ( 8.290806648384990041, -25.50263309590217276, 27.90461065042423527 ) ) ;
#1296=EDGE_CURVE ( 'NONE', #8875, #10017, #1826, .T. ) ;
#1297=CARTESIAN_POINT ( 'NONE',  ( 36.21777210603757169, -2.179854984378739591, -5.859057285912292024 ) ) ;
#1305=CARTESIAN_POINT ( 'NONE',  ( 25.49146503112114459, 2.250848193396226993, 4.142220051770394207 ) ) ;
#1310=ORIENTED_EDGE ( 'NONE', *, *, #18970, .T. ) ;
#1314=CARTESIAN_POINT ( 'NONE',  ( 85.65063761622859317, 0.8893949271338112972, -5.850088623745237193 ) ) ;
#1317=VERTEX_POINT ( 'NONE', #30167 ) ;
#1318=CARTESIAN_POINT ( 'NONE',  ( 24.39763012491684080, 3.159636959096371100, 3.289163722610739082 ) ) ;
#1320=CARTESIAN_POINT ( 'NONE',  ( 17.92594389746831851, -3.172814633591019451, 2.962253944291116436 ) ) ;
#1325=CARTESIAN_POINT ( 'NONE',  ( 23.05869099769193653, 0.3511655747170696062, 5.953694451861818671 ) ) ;
#1337=CARTESIAN_POINT ( 'NONE',  ( 30.01304521823198712, -3.946539318896107318, -3.661452490695084272 ) ) ;
#1340=CARTESIAN_POINT ( 'NONE',  ( -80.58488676320212107, -5.645780868419546294, 5.363795197840156348 ) ) ;
#1341=CARTESIAN_POINT ( 'NONE',  ( 24.74496925782481682, 0.5731625295932825104, -4.778242445000019600 ) ) ;
#1347=CARTESIAN_POINT ( 'NONE',  ( 36.13237780866466409, -1.531151423559755198, -5.643717596868586206 ) ) ;
#1354=CARTESIAN_POINT ( 'NONE',  ( -4.266520354791871306, -48.67644278316300444, 6.000000000000000000 ) ) ;
#1361=VECTOR ( 'NONE', #14321, 1000.000000000000000 ) ;
#1363=CARTESIAN_POINT ( 'NONE',  ( 88.01214243333713227, -2.271333487497714465, 2.136702053253976885 ) ) ;
#1365=CARTESIAN_POINT ( 'NONE',  ( -72.84815947045233031, 2.429809908903064919, -10.96147798754375202 ) ) ;
#1372=AXIS2_PLACEMENT_3D ( 'NONE', #36269, #39544, #11531 ) ;
#1375=CARTESIAN_POINT ( 'NONE',  ( 37.14216958134459645, -2.489364195891544007, 5.966867749344678451 ) ) ;
#1379=CARTESIAN_POINT ( 'NONE',  ( 24.20516649451111491, 2.665701447796034795, 3.984199654269047652 ) ) ;
#1380=CARTESIAN_POINT ( 'NONE',  ( 21.05503876034566346, 6.110295703302774051, -3.370870897236230679 ) ) ;
#1382=CARTESIAN_POINT ( 'NONE',  ( 33.80124125800227830, -4.917752503226308747, -3.288427953259154268 ) ) ;
#1385=CARTESIAN_POINT ( 'NONE',  ( 14.68923871262327374, -4.581893804377800805, 2.499999999999876543 ) ) ;
#1387=CARTESIAN_POINT ( 'NONE',  ( -74.54874278403309518, -2.537033486011438299, -9.369704204412682813 ) ) ;
#1401=CARTESIAN_POINT ( 'NONE',  ( 35.33522315395951097, -3.172769310824047118, 5.721314177413483471 ) ) ;
#1404=CARTESIAN_POINT ( 'NONE',  ( 85.19300053701067554, 2.612159253720373275, 3.340723803646971302 ) ) ;
#1409=EDGE_LOOP ( 'NONE', ( #16820, #14083, #26242, #14507 ) ) ;
#1416=CARTESIAN_POINT ( 'NONE',  ( 25.01091293555841233, 3.329590545877085805, 1.936828124349011526 ) ) ;
#1418=CARTESIAN_POINT ( 'NONE',  ( 24.52405562390649152, 0.9766989416590386996, 4.778545449797553246 ) ) ;
#1422=AXIS2_PLACEMENT_3D ( 'NONE', #5373, #27190, #39748 ) ;
#1426=CARTESIAN_POINT ( 'NONE',  ( -8.400069747914319152, -0.9236158798217076749, 2.500000000000000000 ) ) ;
#1429=CARTESIAN_POINT ( 'NONE',  ( 22.67711167293747465, 4.399063442879564079, -3.239999287829872010 ) ) ;
#1431=CARTESIAN_POINT ( 'NONE',  ( -71.19092636660957396, 0.1906808711754918728, 5.995465708869196497 ) ) ;
#1432=CARTESIAN_POINT ( 'NONE',  ( 21.85643539959776049, -3.145688729744653411, 12.47482453294728266 ) ) ;
#1433=CARTESIAN_POINT ( 'NONE',  ( 21.38787910472312959, 9.379444465854763990, -3.308503362029312722 ) ) ;
#1434=CARTESIAN_POINT ( 'NONE',  ( 16.10543310223363989, 10.11511964520479623, 2.500000000000331291 ) ) ;
#1437=CARTESIAN_POINT ( 'NONE',  ( 88.82472656415403378, -2.095778867207653828, 0.2190179053162402134 ) ) ;
#1440=CARTESIAN_POINT ( 'NONE',  ( -77.48844425012140391, -4.890808455674215516, 9.140760539542357677 ) ) ;
#1443=CARTESIAN_POINT ( 'NONE',  ( 18.21410597459779979, -2.881839143183631879, -3.049149765790359012 ) ) ;
#1444=CARTESIAN_POINT ( 'NONE',  ( 20.42278620884589202, 3.662520991485072042, -3.393867733478101112 ) ) ;
#1450=CARTESIAN_POINT ( 'NONE',  ( 31.91123179551076561, -2.970386030880023398, -5.186917516383627635 ) ) ;
#1453=CARTESIAN_POINT ( 'NONE',  ( 36.20098261264391226, -3.650343263429455476, 5.718100817311416506 ) ) ;
#1457=EDGE_LOOP ( 'NONE', ( #39718, #28497, #15279, #32228 ) ) ;
#1463=CYLINDRICAL_SURFACE ( 'NONE', #28929, 6.000000000000002665 ) ;
#1465=CARTESIAN_POINT ( 'NONE',  ( 22.55238216757502556, 4.103974954327002322, 3.630433831594339633 ) ) ;
#1468=EDGE_CURVE ( 'NONE', #11412, #35457, #22361, .T. ) ;
#1471=FACE_OUTER_BOUND ( 'NONE', #6124, .T. ) ;
#1474=CARTESIAN_POINT ( 'NONE',  ( 22.67441447122924103, 2.915876502080354093, -4.452506167857361419 ) ) ;
#1475=DIRECTION ( 'NONE',  ( -0.000000000000000000, -0.000000000000000000, -1.000000000000000000 ) ) ;
#1481=CARTESIAN_POINT ( 'NONE',  ( 85.82060591106392167, 1.959946745720340777, 4.199140470389015611 ) ) ;
#1482=CARTESIAN_POINT ( 'NONE',  ( 33.33276309746427302, -3.557760156652166383, 5.357383698657358195 ) ) ;
#1484=CARTESIAN_POINT ( 'NONE',  ( -71.32207927536605041, -45.65648572842182062, 9.993882909048494412 ) ) ;
#1486=CARTESIAN_POINT ( 'NONE',  ( -74.48011309984730133, -2.455786751632346832, -10.65291168091849805 ) ) ;
#1489=CARTESIAN_POINT ( 'NONE',  ( 36.79817360360340928, -3.072032592432972553, -5.949642976670753036 ) ) ;
#1498=CARTESIAN_POINT ( 'NONE',  ( 35.34387176057341406, -3.571392527219161561, 5.666785202510572717 ) ) ;
#1506=CARTESIAN_POINT ( 'NONE',  ( 85.38064914651351955, 1.325933486174632359, -5.556288812255563592 ) ) ;
#1508=DIRECTION ( 'NONE',  ( 0.01395351027862084224, -0.9999026450364577601, 0.000000000000000000 ) ) ;
#1509=VECTOR ( 'NONE', #23962, 1000.000000000000000 ) ;
#1512=CARTESIAN_POINT ( 'NONE',  ( 23.74299019415878220, 3.560518783519561303, 3.187235075460781442 ) ) ;
#1516=EDGE_CURVE ( 'NONE', #22380, #20746, #23495, .T. ) ;
#1519=CARTESIAN_POINT ( 'NONE',  ( 26.02524177375569181, 0.8359984680724493744, 4.424135539687619634 ) ) ;
#1525=CARTESIAN_POINT ( 'NONE',  ( -70.92837670882107659, -56.35932253828836025, 0.000000000000000000 ) ) ;
#1526=CARTESIAN_POINT ( 'NONE',  ( 28.77170544830297416, -1.679059579700503901, 5.945470488877720783 ) ) ;
#1530=CARTESIAN_POINT ( 'NONE',  ( -78.62674788310239649, -5.321002937650163744, 8.138356128977308757 ) ) ;
#1531=CARTESIAN_POINT ( 'NONE',  ( 24.12311362605193210, 0.4935845079932565382, -5.095120067356918803 ) ) ;
#1534=DIRECTION ( 'NONE',  ( -0.000000000000000000, -0.000000000000000000, -1.000000000000000000 ) ) ;
#1536=CARTESIAN_POINT ( 'NONE',  ( 33.67912868440872387, -3.778924337320058502, -5.203600794767529791 ) ) ;
#1540=CARTESIAN_POINT ( 'NONE',  ( 0.000000000000000000, 0.000000000000000000, 2.500000000000000000 ) ) ;
#1551=EDGE_CURVE ( 'NONE', #5954, #20746, #16300, .T. ) ;
#1553=CARTESIAN_POINT ( 'NONE',  ( 88.05006142693602555, -2.316660831613085225, -1.868938639203592489 ) ) ;
#1560=DIRECTION ( 'NONE',  ( 1.000000000000000000, 0.000000000000000000, 0.000000000000000000 ) ) ;
#1562=EDGE_CURVE ( 'NONE', #16241, #1778, #14544, .T. ) ;
#1566=CARTESIAN_POINT ( 'NONE',  ( 13.80252864702349314, 11.14042148585687109, -2.500000000000005773 ) ) ;
#1570=CARTESIAN_POINT ( 'NONE',  ( 14.97038224746134816, 12.32935407697701358, -2.523898521188913335 ) ) ;
#1571=CARTESIAN_POINT ( 'NONE',  ( 17.34825500165157308, 14.28608438251766444, 2.500000000000000444 ) ) ;
#1572=CARTESIAN_POINT ( 'NONE',  ( 21.85643539959779247, -13.31640034840845388, 0.8419676367911695936 ) ) ;
#1577=CARTESIAN_POINT ( 'NONE',  ( 14.76025685109631169, -5.148805109997777407, 2.500008232146889942 ) ) ;
#1579=CARTESIAN_POINT ( 'NONE',  ( -76.52714247067879683, -4.348968750379587078, -9.772157169844637892 ) ) ;
#1581=CARTESIAN_POINT ( 'NONE',  ( 33.68523101384537455, -3.842693762900835530, -5.135094833158061256 ) ) ;
#1587=ADVANCED_FACE ( 'NONE', ( #32776 ), #35863, .T. ) ;
#1591=CARTESIAN_POINT ( 'NONE',  ( 87.02342806255605012, 0.6088798157811630141, 4.904800718280144523 ) ) ;
#1596=CARTESIAN_POINT ( 'NONE',  ( 36.14178000185388839, -3.145485669043203814, 5.847196880178433531 ) ) ;
#1599=CARTESIAN_POINT ( 'NONE',  ( 87.65094362820954643, -0.09597545124639318692, -4.742286025697146634 ) ) ;
#1613=CARTESIAN_POINT ( 'NONE',  ( 22.45543544006284620, 0.4771679794038178879, 6.706977661937824742 ) ) ;
#1620=LINE ( 'NONE', #14155, #11937 ) ;
#1622=CARTESIAN_POINT ( 'NONE',  ( 21.90044900377229098, 5.537031193749818669, -3.318543414941498515 ) ) ;
#1626=CARTESIAN_POINT ( 'NONE',  ( 22.39040353993711108, 2.683735211801196563, -8.168217153243197970 ) ) ;
#1627=CARTESIAN_POINT ( 'NONE',  ( 16.55058170395099637, 7.675961124049503148, 3.484773800359490359 ) ) ;
#1630=CARTESIAN_POINT ( 'NONE',  ( 87.30391260081773908, -0.2898811470106905652, 5.673122884556256906 ) ) ;
#1631=DIRECTION ( 'NONE',  ( 0.000000000000000000, -0.000000000000000000, -1.000000000000000000 ) ) ;
#1636=CIRCLE ( 'NONE', #21354, 10.00000000000000533 ) ;
#1638=CARTESIAN_POINT ( 'NONE',  ( 31.37357152309853348, -3.143197726502084954, -5.103002627509826361 ) ) ;
#1639=CARTESIAN_POINT ( 'NONE',  ( 35.33510904524467833, -3.167696954624281691, -5.721296367988784048 ) ) ;
#1640=CARTESIAN_POINT ( 'NONE',  ( -17.27251170661583402, 3.729367930467589076, -6.000000000000000000 ) ) ;
#1641=B_SPLINE_CURVE_WITH_KNOTS ( 'NONE', 3,
 ( #33052, #20678, #1766, #10796, #33260, #39207, #39617, #5660, #30373, #17786, #24807, #14914, #2599, #11805, #12015, #13247, #10150, #31796, #35303, #15527, #21920, #18817, #3216, #12639, #16933, #29702, #20425, #23721, #1320, #19836, #29108, #22938, #4202, #27419 ),
 .UNSPECIFIED., .F., .F.,
 ( 4, 2, 2, 1, 1, 1, 1, 1, 1, 2, 2, 2, 2, 1, 1, 1, 1, 1, 1, 2, 2, 2, 4 ),
 ( 0.000000000000000000, 0.2499999999999977796, 0.3749999999999966693, 0.4374999999999957812, 0.4687499999999956701, 0.4843749999999956701, 0.4921874999999956146, 0.4960937499999956146, 0.4980468749999955591, 0.4990234374999951705, 0.4999999999999947820, 0.6249999999999529265, 0.6874999999999320544, 0.7187499999999212852, 0.7343749999999154010, 0.7421874999999126254, 0.7460937499999110711, 0.7480468749999104050, 0.7490234374999100719, 0.7495117187499102940, 0.7499999999999105160, 0.8749999999999553690, 1.000000000000000000 ),
 .UNSPECIFIED. ) ;
#1642=CARTESIAN_POINT ( 'NONE',  ( 21.81791346015125654, 0.2734699911238404058, -8.212990486451831273 ) ) ;
#1644=ORIENTED_EDGE ( 'NONE', *, *, #31991, .T. ) ;
#1645=CARTESIAN_POINT ( 'NONE',  ( 36.42057415831622080, -3.112379919131356143, 5.890709450956581605 ) ) ;
#1653=CARTESIAN_POINT ( 'NONE',  ( 37.10978108531639919, -2.403808732534971515, 5.951661781935858819 ) ) ;
#1656=CARTESIAN_POINT ( 'NONE',  ( 86.49500509992682851, -0.6166496396440827032, 5.723172357827475132 ) ) ;
#1663=DIRECTION ( 'NONE',  ( 0.000000000000000000, -0.000000000000000000, -1.000000000000000000 ) ) ;
#1667=CARTESIAN_POINT ( 'NONE',  ( 22.94147134705455926, 4.030654817714214744, 3.371037374912960960 ) ) ;
#1669=AXIS2_PLACEMENT_3D ( 'NONE', #7800, #8398, #33552 ) ;
#1671=CARTESIAN_POINT ( 'NONE',  ( 1.700390093233090871, -29.56993018339339940, -15.49999999999999822 ) ) ;
#1675=CARTESIAN_POINT ( 'NONE',  ( 18.72828149013939125, -2.774847064971670552, -3.129399290372459674 ) ) ;
#1678=VERTEX_POINT ( 'NONE', #30276 ) ;
#1679=CARTESIAN_POINT ( 'NONE',  ( 23.39550106081508218, 2.664895405987246502, -4.239314792157373724 ) ) ;
#1687=CARTESIAN_POINT ( 'NONE',  ( 86.26657670271889344, 1.459011185482768314, -4.895973709007312991 ) ) ;
#1688=CARTESIAN_POINT ( 'NONE',  ( 33.73883514186113075, -4.630787605642836091, -3.992050560354765576 ) ) ;
#1690=CARTESIAN_POINT ( 'NONE',  ( -74.72715548395238727, -2.765387099023297157, -10.57877961556935098 ) ) ;
#1693=CARTESIAN_POINT ( 'NONE',  ( 37.05749439986598759, -2.899774270594387637, -5.990116258624699874 ) ) ;
#1697=EDGE_CURVE ( 'NONE', #3707, #35445, #36857, .T. ) ;
#1698=AXIS2_PLACEMENT_3D ( 'NONE', #31877, #10433, #38229 ) ;
#1703=CARTESIAN_POINT ( 'NONE',  ( 36.69966961405233263, -3.382783021916500044, 5.888606945404527337 ) ) ;
#1711=CARTESIAN_POINT ( 'NONE',  ( 85.66380979468560497, 0.8667738229574647457, -5.860807272458633754 ) ) ;
#1712=CARTESIAN_POINT ( 'NONE',  ( -78.91378792136296738, 11.43306328107894032, 6.033766101647666247 ) ) ;
#1715=ORIENTED_EDGE ( 'NONE', *, *, #26675, .F. ) ;
#1716=CARTESIAN_POINT ( 'NONE',  ( 24.06494024425525069, 3.347574872190568929, 3.211326713574206515 ) ) ;
#1722=B_SPLINE_CURVE_WITH_KNOTS ( 'NONE', 3,
 ( #37789, #12892, #38000, #9801 ),
 .UNSPECIFIED., .F., .F.,
 ( 4, 4 ),
 ( 0.000000000000000000, 1.000000000000000000 ),
 .UNSPECIFIED. ) ;
#1723=CARTESIAN_POINT ( 'NONE',  ( 26.06744471409270147, 0.7518114339798734891, 4.421646308027469274 ) ) ;
#1724=CARTESIAN_POINT ( 'NONE',  ( 14.76771331554806999, -5.163171487644635960, -2.500000296585186632 ) ) ;
#1729=CARTESIAN_POINT ( 'NONE',  ( 35.64856448684500378, -3.751217397768356054, -5.580918352854083331 ) ) ;
#1733=CARTESIAN_POINT ( 'NONE',  ( 29.34753533916922308, -2.431376398363487734, 5.582488461359439214 ) ) ;
#1737=CARTESIAN_POINT ( 'NONE',  ( 21.78667867209630060, 0.2188310260794802675, -8.380823656482592199 ) ) ;
#1738=VECTOR ( 'NONE', #25826, 1000.000000000000000 ) ;
#1743=CARTESIAN_POINT ( 'NONE',  ( 36.68395750019694646, -1.917487243977046729, -5.804568023447322034 ) ) ;
#1757=CARTESIAN_POINT ( 'NONE',  ( 85.19771215196759329, 1.813128620488922760, 5.066052097874169213 ) ) ;
#1766=CARTESIAN_POINT ( 'NONE',  ( 27.40362055195197755, -3.367332562137738794, 4.313861870170892843 ) ) ;
#1769=CARTESIAN_POINT ( 'NONE',  ( 37.14318591385630697, -2.491847215272260829, 5.967311536227382085 ) ) ;
#1770=ADVANCED_FACE ( 'NONE', ( #15029, #20796 ), #33390, .T. ) ;
#1773=CARTESIAN_POINT ( 'NONE',  ( 23.14887797670855107, 3.363171500915444589, 3.819340284631616900 ) ) ;
#1775=CARTESIAN_POINT ( 'NONE',  ( 16.11725891508299924, 15.27317977276803873, 2.500000000000000000 ) ) ;
#1777=CARTESIAN_POINT ( 'NONE',  ( 21.85643539959774628, 6.760345589247273246, -10.71366635798555578 ) ) ;
#1778=VERTEX_POINT ( 'NONE', #11117 ) ;
#1779=CARTESIAN_POINT ( 'NONE',  ( -80.90823458386326195, 10.55951580149532809, 0.6344085041158121774 ) ) ;
#1782=CARTESIAN_POINT ( 'NONE',  ( 14.75796219645098795, -5.141356742665804447, 2.500016127560962254 ) ) ;
#1784=CARTESIAN_POINT ( 'NONE',  ( -77.44075151393023759, 9.727190932936968792, -9.175713659463616167 ) ) ;
#1786=CARTESIAN_POINT ( 'NONE',  ( 37.01100706631705606, -2.247765066581573823, -5.912597513712233521 ) ) ;
#1792=VECTOR ( 'NONE', #31538, 1000.000000000000000 ) ;
#1796=CARTESIAN_POINT ( 'NONE',  ( 86.98314280420640898, 0.6541301300131903140, 4.930073579784800764 ) ) ;
#1801=CARTESIAN_POINT ( 'NONE',  ( 36.64085946849131403, -3.117955867178630935, 5.925090301229771761 ) ) ;
#1804=CARTESIAN_POINT ( 'NONE',  ( 86.49834695356116754, 1.198675839257056230, 5.248227958817050620 ) ) ;
#1813=VERTEX_POINT ( 'NONE', #34000 ) ;
#1820=VECTOR ( 'NONE', #81, 1000.000000000000000 ) ;
#1822=CARTESIAN_POINT ( 'NONE',  ( 26.76923719187233175, 1.540101848406568052, 4.364735894841153652 ) ) ;
#1826=B_SPLINE_CURVE_WITH_KNOTS ( 'NONE', 3,
 ( #8325, #1380, #10610, #29560, #35754, #13910, #32865, #17188, #33064, #5256, #20480, #4848, #1570, #14704, #20689, #17796 ),
 .UNSPECIFIED., .F., .F.,
 ( 4, 2, 2, 2, 2, 2, 2, 4 ),
 ( 0.000000000000000000, 0.002644435627895791452, 0.005288871255791582904, 0.006611089069739476028, 0.007933306883687369152, 0.009255524697635263143, 0.009916633604609207536, 0.01057774251158315366 ),
 .UNSPECIFIED. ) ;
#1829=CARTESIAN_POINT ( 'NONE',  ( -70.92837670882107659, -23.80776546975053165, -6.000000000000002665 ) ) ;
#1830=DIRECTION ( 'NONE',  ( -0.000000000000000000, -0.000000000000000000, -1.000000000000000000 ) ) ;
#1834=CARTESIAN_POINT ( 'NONE',  ( 22.76078985634742935, 3.901595487204953638, -3.625275301636816216 ) ) ;
#1838=CARTESIAN_POINT ( 'NONE',  ( 21.85643539959774273, 9.212406492340052822, 1.715677401501900956 ) ) ;
#1842=CARTESIAN_POINT ( 'NONE',  ( 84.91553621511910421, 2.364970790127210787, 4.120477167815592701 ) ) ;
#1848=LINE ( 'NONE', #5324, #11132 ) ;
#1849=CARTESIAN_POINT ( 'NONE',  ( 26.27693392017907925, -3.249033630802554473, -4.181544638722900054 ) ) ;
#1850=CARTESIAN_POINT ( 'NONE',  ( 34.92931741750302876, -1.710645300694223492, -5.657962770372154893 ) ) ;
#1851=CARTESIAN_POINT ( 'NONE',  ( 8.290806648384990041, 0.000000000000000000, 6.000000000000000000 ) ) ;
#1852=CARTESIAN_POINT ( 'NONE',  ( 22.33694865187872480, 0.2827817013730578033, -7.021907440927535937 ) ) ;
#1855=CARTESIAN_POINT ( 'NONE',  ( 31.71703756440468069, -0.5641108459604192715, 5.156608810014274624 ) ) ;
#1860=CARTESIAN_POINT ( 'NONE',  ( 37.00876839025129073, -3.246501946636328295, 5.946957662215321072 ) ) ;
#1862=CARTESIAN_POINT ( 'NONE',  ( 16.71262745093176250, -3.379652782812611722, -2.787236875488859678 ) ) ;
#1864=VERTEX_POINT ( 'NONE', #24712 ) ;
#1869=CIRCLE ( 'NONE', #23572, 10.00000000000000888 ) ;
#1876=CARTESIAN_POINT ( 'NONE',  ( 24.35455115775381785, 2.928845783586057738, 3.741716916781699709 ) ) ;
#1878=ADVANCED_FACE ( 'NONE', ( #2915 ), #23044, .T. ) ;
#1885=CARTESIAN_POINT ( 'NONE',  ( 22.71051984177768190, 2.583563127446080188, -4.683974715729272376 ) ) ;
#1888=EDGE_CURVE ( 'NONE', #38890, #24333, #37427, .T. ) ;
#1889=AXIS2_PLACEMENT_3D ( 'NONE', #26254, #13475, #22962 ) ;
#1890=FACE_OUTER_BOUND ( 'NONE', #23994, .T. ) ;
#1897=CARTESIAN_POINT ( 'NONE',  ( 88.10293741339057760, -0.6036763236807990429, 2.641732887311516453 ) ) ;
#1898=CARTESIAN_POINT ( 'NONE',  ( 31.05604276399450114, -2.500009215535430762, 5.784057531382419626 ) ) ;
#1901=CARTESIAN_POINT ( 'NONE',  ( -81.21715035842910879, -5.646436377738331736, -3.817250611473149036 ) ) ;
#1902=CARTESIAN_POINT ( 'NONE',  ( 23.84748567078391446, -3.102047020920744913, 3.830198175285921547 ) ) ;
#1904=CARTESIAN_POINT ( 'NONE',  ( 31.75256816120542425, -0.4599525743511591602, -5.162154218955760321 ) ) ;
#1910=ORIENTED_EDGE ( 'NONE', *, *, #29793, .T. ) ;
#1911=CARTESIAN_POINT ( 'NONE',  ( 35.36141464313556071, -3.735660561169047877, 5.554341061716538519 ) ) ;
#1924=CARTESIAN_POINT ( 'NONE',  ( 24.73621386372994380, 3.010848716420428062, 3.391332750938185203 ) ) ;
#1932=( BOUNDED_SURFACE ( )  B_SPLINE_SURFACE ( 3, 2, ( 
 ( #17523, #7680, #33212 ),
 ( #19839, #20230, #17130 ),
 ( #30118, #1127, #26428 ),
 ( #29905, #38956, #14049 ) ),
 .UNSPECIFIED., .F., .F., .T. ) 
 B_SPLINE_SURFACE_WITH_KNOTS ( ( 4, 4 ),
 ( 3, 3 ),
 ( 0.1160256260365885861, 0.1317056536943987943 ),
 ( 0.000000000000000000, 0.8973000442991090342 ),
 .UNSPECIFIED. ) 
 GEOMETRIC_REPRESENTATION_ITEM ( )  RATIONAL_B_SPLINE_SURFACE ( (
 ( 1.000000000000000000, 0.9342716120537195579, 0.9864993949392519834),
 ( 1.000000000000000000, 0.9342716120537195579, 0.9864993949392519834),
 ( 1.000000000000000000, 0.9342716120537194469, 0.9864993949392519834),
 ( 1.000000000000000000, 0.9342716120537194469, 0.9864993949392519834) ) ) 
 REPRESENTATION_ITEM ( '' )  SURFACE ( )  );
#1933=CARTESIAN_POINT ( 'NONE',  ( 24.11607445809433514, 0.4540071914542280762, 5.103030637244794221 ) ) ;
#1937=ADVANCED_FACE ( 'NONE', ( #20372 ), #1463, .F. ) ;
#1939=CARTESIAN_POINT ( 'NONE',  ( 35.41233797231917890, -3.779600677375021256, -5.524434929723343046 ) ) ;
#1943=CARTESIAN_POINT ( 'NONE',  ( 37.83867290611771494, -6.084034091406928191, -6.000000000000000000 ) ) ;
#1944=CARTESIAN_POINT ( 'NONE',  ( 27.52542935251784328, 0.09321990139520379415, -5.913109915068038624 ) ) ;
#1945=DIRECTION ( 'NONE',  ( 0.000000000000000000, 0.000000000000000000, -1.000000000000000000 ) ) ;
#1948=CARTESIAN_POINT ( 'NONE',  ( -81.80090188080515645, -5.603160304130406111, -0.6545554231109771415 ) ) ;
#1949=CARTESIAN_POINT ( 'NONE',  ( 23.58764223058103227, 0.4154427152156035530, -5.528209969427812176 ) ) ;
#1954=CARTESIAN_POINT ( 'NONE',  ( -71.84266479621042834, -48.31020963306245619, 9.958452096079875915 ) ) ;
#1955=CARTESIAN_POINT ( 'NONE',  ( 30.88234279937811166, 0.6976323447808369105, -4.494874676303273198 ) ) ;
#1958=CYLINDRICAL_SURFACE ( 'NONE', #12107, 3.000000000000002665 ) ;
#1966=CARTESIAN_POINT ( 'NONE',  ( -69.72971309252355354, -48.03957001906470481, 5.880709122941769174 ) ) ;
#1971=CARTESIAN_POINT ( 'NONE',  ( -62.92837670882106238, -23.80776546975053520, -6.000000000000000000 ) ) ;
#1978=CARTESIAN_POINT ( 'NONE',  ( 24.08390956300509700, 3.360009220450308032, 3.160289221677234028 ) ) ;
#1979=CIRCLE ( 'NONE', #22376, 10.00000000000000888 ) ;
#1982=CARTESIAN_POINT ( 'NONE',  ( 16.28258139852007957, 10.03625398311444705, -2.500000000000424993 ) ) ;
#1989=DIRECTION ( 'NONE',  ( -1.000000000000000000, 0.000000000000000000, 0.000000000000000000 ) ) ;
#1990=CARTESIAN_POINT ( 'NONE',  ( 21.85643539959778181, 10.07385928288181987, 4.538892979079195200 ) ) ;
#1992=CARTESIAN_POINT ( 'NONE',  ( -79.67878442765989178, 10.46676075307951592, 4.855440592539105538 ) ) ;
#1994=CARTESIAN_POINT ( 'NONE',  ( 14.73988855999587422, -5.058265782967484192, 2.500274136440799211 ) ) ;
#1995=CARTESIAN_POINT ( 'NONE',  ( -80.59971289683194584, 10.50603676119796503, -5.334131017465025160 ) ) ;
#2001=CARTESIAN_POINT ( 'NONE',  ( -4.890026461918812295, -8.951974136083761024, 2.500000000000000000 ) ) ;
#2002=CARTESIAN_POINT ( 'NONE',  ( -70.92837670881976919, 0.2170085631237942680, 10.00000000000113154 ) ) ;
#2004=CARTESIAN_POINT ( 'NONE',  ( 87.91376162421416041, -0.3911850984532471154, 3.331745215148313122 ) ) ;
#2008=CARTESIAN_POINT ( 'NONE',  ( 36.19519395851039434, -2.229529781144294898, 5.855533419936117312 ) ) ;
#2009=EDGE_CURVE ( 'NONE', #13035, #3867, #19725, .T. ) ;
#2011=CARTESIAN_POINT ( 'NONE',  ( 86.86561140461988373, 0.2703162379016064154, -5.930766725306959586 ) ) ;
#2013=CARTESIAN_POINT ( 'NONE',  ( 31.00707005056823817, -0.8718966892480422004, 5.891928739871540088 ) ) ;
#2014=CARTESIAN_POINT ( 'NONE',  ( 33.70392053634464702, -1.255035446422470891, -5.466709950731788226 ) ) ;
#2019=EDGE_CURVE ( 'NONE', #17221, #8271, #9087, .T. ) ;
#2020=VERTEX_POINT ( 'NONE', #22027 ) ;
#2025=CARTESIAN_POINT ( 'NONE',  ( 22.22833818514967419, 0.9551375975900053827, 6.581072739463595944 ) ) ;
#2031=EDGE_CURVE ( 'NONE', #7067, #4684, #22895, .T. ) ;
#2032=CARTESIAN_POINT ( 'NONE',  ( 91.69672933337632514, -4.640393979863029372, -6.000000000000000888 ) ) ;
#2033=CARTESIAN_POINT ( 'NONE',  ( 11.29080664838498826, -10.90558813203967148, 6.000000000000000000 ) ) ;
#2037=CARTESIAN_POINT ( 'NONE',  ( 21.91451482393930306, 5.430938580357159040, -3.368358593842193383 ) ) ;
#2038=ORIENTED_EDGE ( 'NONE', *, *, #215, .T. ) ;
#2040=CARTESIAN_POINT ( 'NONE',  ( 22.82080504511013430, -6.970192185297126031, -1.116939615399285657 ) ) ;
#2045=CARTESIAN_POINT ( 'NONE',  ( 85.85763368383675243, 1.114829962406831410, -5.799110970849834068 ) ) ;
#2049=EDGE_CURVE ( 'NONE', #15393, #2537, #290, .T. ) ;
#2052=CARTESIAN_POINT ( 'NONE',  ( 14.81973502151181243, -5.946294937045099260, -2.518644691825020931 ) ) ;
#2053=CARTESIAN_POINT ( 'NONE',  ( 35.45276959245764203, -1.916775701034503898, -5.739660142012472654 ) ) ;
#2055=CARTESIAN_POINT ( 'NONE',  ( 23.10155575571232234, 0.3729460866388023543, -5.910048752073230105 ) ) ;
#2058=CARTESIAN_POINT ( 'NONE',  ( 21.25143394907042449, 3.315796038557054182, 3.523198254261666218 ) ) ;
#2060=CARTESIAN_POINT ( 'NONE',  ( 31.84521792906302906, -2.966245498930080160, -5.176614455973063578 ) ) ;
#2063=CARTESIAN_POINT ( 'NONE',  ( 37.01052352883407082, -2.248283349646221563, 5.912786814818789871 ) ) ;
#2071=EDGE_CURVE ( 'NONE', #18532, #22978, #40503, .T. ) ;
#2072=DIRECTION ( 'NONE',  ( 1.000000000000000000, 0.000000000000000000, 0.000000000000000000 ) ) ;
#2082=CARTESIAN_POINT ( 'NONE',  ( 22.49878221582566340, 4.485478565812190510, 3.364408562939156244 ) ) ;
#2087=CARTESIAN_POINT ( 'NONE',  ( 18.17282410049547536, -2.848335441370983379, -3.042706730930791803 ) ) ;
#2088=CARTESIAN_POINT ( 'NONE',  ( -80.92837670882107659, 2.429809908903242555, 12.50000000000000000 ) ) ;
#2090=CARTESIAN_POINT ( 'NONE',  ( 24.46993583969108244, 2.591970903540452120, -3.976734763430334496 ) ) ;
#2095=CARTESIAN_POINT ( 'NONE',  ( 86.64693249831780975, 1.031777503091004800, -5.158387491453222395 ) ) ;
#2096=CARTESIAN_POINT ( 'NONE',  ( 31.72291873093343284, -3.714249907566092634, 4.801291842747894556 ) ) ;
#2099=CARTESIAN_POINT ( 'NONE',  ( 14.91371995633972247, -5.924865805607109515, 2.519702374887847096 ) ) ;
#2102=CARTESIAN_POINT ( 'NONE',  ( 35.50436178781468755, -1.785355687363928689, -5.747712351859902924 ) ) ;
#2106=ADVANCED_FACE ( 'NONE', ( #17375 ), #15506, .F. ) ;
#2107=DIRECTION ( 'NONE',  ( 0.000000000000000000, 0.000000000000000000, -1.000000000000000000 ) ) ;
#2108=CARTESIAN_POINT ( 'NONE',  ( -70.17520183749425655, -45.81613455447481442, 5.953107086803218095 ) ) ;
#2111=CARTESIAN_POINT ( 'NONE',  ( 37.06794226148818439, -2.451797619550506901, 5.964046084392197855 ) ) ;
#2120=CARTESIAN_POINT ( 'NONE',  ( -75.29003035974771763, 9.883927643020312459, 9.004751556950759905 ) ) ;
#2122=EDGE_CURVE ( 'NONE', #2020, #23233, #18410, .T. ) ;
#2125=CARTESIAN_POINT ( 'NONE',  ( 23.74487617493794644, 3.563056966343403076, 3.179706526333272887 ) ) ;
#2131=CARTESIAN_POINT ( 'NONE',  ( 27.43005921570062355, 0.9938728547065163177, 4.487513223811070873 ) ) ;
#2132=CARTESIAN_POINT ( 'NONE',  ( 14.72813615105396323, -4.875043543781444555, -2.502213707555314581 ) ) ;
#2142=CARTESIAN_POINT ( 'NONE',  ( 27.17726507492083599, 0.7866376163037266389, 5.581651230154481169 ) ) ;
#2147=CARTESIAN_POINT ( 'NONE',  ( 21.78050909960382953, 0.2073865793812009195, -8.415697349445284914 ) ) ;
#2152=CARTESIAN_POINT ( 'NONE',  ( -72.38841993492154359, -47.51249456017484363, 9.893128921701961787 ) ) ;
#2153=CARTESIAN_POINT ( 'NONE',  ( 37.21138578923722662, -2.744110368974991498, -6.000908943309275045 ) ) ;
#2161=CARTESIAN_POINT ( 'NONE',  ( 21.79832107181720957, 1.471655218185874858, -6.775317797187613067 ) ) ;
#2181=CARTESIAN_POINT ( 'NONE',  ( 18.26922853518255252, 11.64739320590812888, -2.500000000000005773 ) ) ;
#2188=CARTESIAN_POINT ( 'NONE',  ( 21.85643539959774273, 11.87467848218428834, -0.9583437110454642305 ) ) ;
#2192=CARTESIAN_POINT ( 'NONE',  ( 14.76646934850686321, -4.520893997360137639, 2.511033383266843888 ) ) ;
#2193=CARTESIAN_POINT ( 'NONE',  ( -74.87089915843765198, 7.795108144428510855, -9.236877437684523073 ) ) ;
#2197=CARTESIAN_POINT ( 'NONE',  ( 14.72032977250883334, 13.14393988312540529, 2.499678740116445752 ) ) ;
#2207=CARTESIAN_POINT ( 'NONE',  ( 34.13188676842981550, -3.213403896779438718, 5.533504431668644585 ) ) ;
#2210=CARTESIAN_POINT ( 'NONE',  ( 88.65680102019307185, -1.418189719613276223, -2.767552868364703045 ) ) ;
#2212=CARTESIAN_POINT ( 'NONE',  ( 31.80158048871438581, -1.669318041804891850, 6.009059823207920203 ) ) ;
#2224=CARTESIAN_POINT ( 'NONE',  ( 26.67559340739115115, 0.9924815708228320599, 4.380057119474870753 ) ) ;
#2238=CARTESIAN_POINT ( 'NONE',  ( 22.22276440514101381, 5.121701983031256233, -3.164228572747696422 ) ) ;
#2241=CARTESIAN_POINT ( 'NONE',  ( 26.56634348862415251, 2.991955253353971500, -0.5426703667890996341 ) ) ;
#2245=CARTESIAN_POINT ( 'NONE',  ( 84.85978623402763787, 2.253055191119315737, -4.296636491436513161 ) ) ;
#2251=CARTESIAN_POINT ( 'NONE',  ( 21.51474421073843502, -2.978796432270695682, -3.508324343008054846 ) ) ;
#2253=PLANE ( 'NONE',  #7556 ) ;
#2255=EDGE_LOOP ( 'NONE', ( #30060, #4003, #25056, #9557, #12158, #12053, #15972, #4464 ) ) ;
#2257=CARTESIAN_POINT ( 'NONE',  ( 86.06238440510853138, 1.688369665709827272, 4.446988894268222303 ) ) ;
#2262=CARTESIAN_POINT ( 'NONE',  ( 33.68538319921849933, -3.842697165577637186, 5.135126983811714396 ) ) ;
#2264=CARTESIAN_POINT ( 'NONE',  ( 16.87423662129170765, -3.093369055974038329, 2.840030748344179568 ) ) ;
#2265=CARTESIAN_POINT ( 'NONE',  ( 16.92519036607385985, -3.330348903852535791, -2.818005368153482237 ) ) ;
#2269=ORIENTED_EDGE ( 'NONE', *, *, #8966, .T. ) ;
#2271=CARTESIAN_POINT ( 'NONE',  ( -5.316495087772349137, -32.84709638682603838, -2.500000000000000444 ) ) ;
#2278=ORIENTED_EDGE ( 'NONE', *, *, #8027, .F. ) ;
#2283=DIRECTION ( 'NONE',  ( 0.000000000000000000, 0.000000000000000000, 1.000000000000000000 ) ) ;
#2284=CARTESIAN_POINT ( 'NONE',  ( 26.06061125667445921, -2.757087722844052902, -4.273786683505784723 ) ) ;
#2287=CARTESIAN_POINT ( 'NONE',  ( 22.65677964865432870, 3.082858489129792545, -4.336902647173903169 ) ) ;
#2293=FACE_OUTER_BOUND ( 'NONE', #31505, .T. ) ;
#2295=CARTESIAN_POINT ( 'NONE',  ( 85.17388679999480416, 2.686372346413934409, 1.032998165733738816 ) ) ;
#2299=ADVANCED_FACE ( 'NONE', ( #20234 ), #19648, .F. ) ;
#2303=CARTESIAN_POINT ( 'NONE',  ( 21.53627039407701460, -3.050411829391824536, 3.479264532985287595 ) ) ;
#2305=CARTESIAN_POINT ( 'NONE',  ( 36.14161076797949335, -3.144492548583445846, -5.847170467139393146 ) ) ;
#2313=CARTESIAN_POINT ( 'NONE',  ( 20.85071236293282482, 4.522924277292770689, 2.940040760293478161 ) ) ;
#2322=CARTESIAN_POINT ( 'NONE',  ( -75.61141378505557498, -5.258309523962441112, -8.843508591838688204 ) ) ;
#2330=CARTESIAN_POINT ( 'NONE',  ( 23.72810756034646218, 3.537902271613312610, 3.249573880183133312 ) ) ;
#2337=CARTESIAN_POINT ( 'NONE',  ( 22.61186175525197939, 0.2941385288943472176, 6.499543881263520895 ) ) ;
#2338=CARTESIAN_POINT ( 'NONE',  ( 14.62968864654182433, -4.708885747848794878, -2.500000000000228706 ) ) ;
#2344=CARTESIAN_POINT ( 'NONE',  ( 35.77311163637067182, -3.731966479379717594, -5.611466549886873878 ) ) ;
#2349=FACE_BOUND ( 'NONE', #29906, .T. ) ;
#2350=CARTESIAN_POINT ( 'NONE',  ( 30.13988473044573624, 0.1694294105150049301, -5.382122866902316893 ) ) ;
#2351=B_SPLINE_CURVE_WITH_KNOTS ( 'NONE', 3,
 ( #6009, #15058, #37082, #24740, #21045, #27411, #28024, #8873, #39974, #2739, #5599, #5804, #5393, #30307 ),
 .UNSPECIFIED., .F., .F.,
 ( 4, 2, 2, 2, 2, 2, 4 ),
 ( 0.000000000000000000, 0.002649657113267142768, 0.005299314226534285535, 0.007948971339801423966, 0.009273799896434993181, 0.009936214174751781258, 0.01059862845306856587 ),
 .UNSPECIFIED. ) ;
#2354=CARTESIAN_POINT ( 'NONE',  ( -81.72496613755205885, -5.611374088600661558, 1.578727716436091333 ) ) ;
#2355=CARTESIAN_POINT ( 'NONE',  ( 25.38754743222835231, 0.7148885839003105147, -4.601077336691401953 ) ) ;
#2360=VECTOR ( 'NONE', #7370, 1000.000000000000000 ) ;
#2362=CARTESIAN_POINT ( 'NONE',  ( -71.41219010185693605, -48.54025046412724009, 9.988702396128939398 ) ) ;
#2363=CARTESIAN_POINT ( 'NONE',  ( 23.38378197942683201, 3.557987824482284456, -3.100743960359395146 ) ) ;
#2366=DIRECTION ( 'NONE',  ( 1.000000000000000000, 0.000000000000000000, 0.000000000000000000 ) ) ;
#2369=CARTESIAN_POINT ( 'NONE',  ( -73.32694038987526142, 5.199692155526626891, 10.90380950792603443 ) ) ;
#2372=CARTESIAN_POINT ( 'NONE',  ( 14.72861853083255035, -4.938210908769336882, -2.501287736049143895 ) ) ;
#2373=CARTESIAN_POINT ( 'NONE',  ( 22.25801210972482380, 1.411373041331142941, -6.101462656651117200 ) ) ;
#2379=CARTESIAN_POINT ( 'NONE',  ( 86.14505873727070195, -0.01797735283943463491, 5.995667628870159582 ) ) ;
#2381=CARTESIAN_POINT ( 'NONE',  ( 21.58862418887968460, 7.202556094215188054, 2.923978954502209682 ) ) ;
#2387=CARTESIAN_POINT ( 'NONE',  ( 21.70916979853645756, 6.353179628818696578, 3.184481357965229797 ) ) ;
#2393=CARTESIAN_POINT ( 'NONE',  ( 16.14085281723246013, 12.58767971060109758, -2.499999999999998668 ) ) ;
#2402=CARTESIAN_POINT ( 'NONE',  ( 21.85643539959774273, 10.50077279934518160, -1.805501455388072385 ) ) ;
#2404=CARTESIAN_POINT ( 'NONE',  ( -77.68413004431236857, 11.14508354151945113, 7.383713242483813666 ) ) ;
#2405=CARTESIAN_POINT ( 'NONE',  ( -17.69482985384422236, -39.37473357531881391, 6.000000000000000000 ) ) ;
#2409=CARTESIAN_POINT ( 'NONE',  ( -78.64083763406480898, 10.18485694350484927, -8.124114778902974621 ) ) ;
#2413=CARTESIAN_POINT ( 'NONE',  ( 14.73716873398060478, 12.66775802014586105, 2.506489619347135545 ) ) ;
#2418=CARTESIAN_POINT ( 'NONE',  ( -70.92837670882107659, 13.87661300689599386, 6.000000000000002665 ) ) ;
#2419=CARTESIAN_POINT ( 'NONE',  ( 24.61164019132730374, 2.699834716109671184, -3.894731277034012340 ) ) ;
#2423=STYLED_ITEM('',(#40738),#39057);
#2425=CARTESIAN_POINT ( 'NONE',  ( 37.05753485607799291, -2.899691229771081069, 5.990122572795006484 ) ) ;
#2428=CARTESIAN_POINT ( 'NONE',  ( 88.82472656415403378, -2.095778867207653828, 0.2190179053162402134 ) ) ;
#2433=CARTESIAN_POINT ( 'NONE',  ( 85.57577930415899914, 1.015208198401525541, 5.782835925834406865 ) ) ;
#2443=CARTESIAN_POINT ( 'NONE',  ( 22.37141982511144889, 0.3128190655527079977, 6.946763763332127972 ) ) ;
#2449=CARTESIAN_POINT ( 'NONE',  ( 25.88590780377253964, -5.105876911915265381, 3.183034662934932868 ) ) ;
#2453=CARTESIAN_POINT ( 'NONE',  ( 23.42389927133387317, 3.726266061901138738, -3.241371881706822222 ) ) ;
#2454=EDGE_LOOP ( 'NONE', ( #3913, #20566, #18074, #14726 ) ) ;
#2458=CARTESIAN_POINT ( 'NONE',  ( 24.33259761278756272, 0.1721304915443387373, 6.926443425830641765 ) ) ;
#2463=CARTESIAN_POINT ( 'NONE',  ( 87.68748590470411841, -1.878626560869070872, 3.708385665356400906 ) ) ;
#2464=CARTESIAN_POINT ( 'NONE',  ( -70.92837670882107659, -37.87473357531881391, 0.000000000000000000 ) ) ;
#2467=PLANE ( 'NONE',  #8 ) ;
#2468=CARTESIAN_POINT ( 'NONE',  ( 14.79422032056577052, -5.583071962950631573, -2.503592320680073424 ) ) ;
#2469=CARTESIAN_POINT ( 'NONE',  ( 29.09904249065658277, 0.3518783346174893523, -4.748007362305766144 ) ) ;
#2472=ORIENTED_EDGE ( 'NONE', *, *, #17443, .T. ) ;
#2474=CARTESIAN_POINT ( 'NONE',  ( 86.56125476490799997, 1.128014799767447229, 4.962829853851403961 ) ) ;
#2476=ORIENTED_EDGE ( 'NONE', *, *, #32019, .T. ) ;
#2478=CARTESIAN_POINT ( 'NONE',  ( 36.20144388887960218, -3.653144936024889322, 5.716525466092109653 ) ) ;
#2479=CARTESIAN_POINT ( 'NONE',  ( 22.73643742276861346, -2.655319355651748925, 3.754968961276796247 ) ) ;
#2484=EDGE_LOOP ( 'NONE', ( #3436, #28923, #6825, #34739 ) ) ;
#2486=ORIENTED_EDGE ( 'NONE', *, *, #18879, .T. ) ;
#2491=CARTESIAN_POINT ( 'NONE',  ( 22.96819900907483358, 2.437540201623891623, 4.628877954886912782 ) ) ;
#2492=CARTESIAN_POINT ( 'NONE',  ( 31.33775714179567373, 0.5243197422169587618, 4.587784402887622903 ) ) ;
#2498=CARTESIAN_POINT ( 'NONE',  ( 22.18386873814171878, -2.652701146302887558, -3.668727254116632253 ) ) ;
#2501=CARTESIAN_POINT ( 'NONE',  ( 23.03775345957872389, 3.287047143578627484, -3.951504299623971317 ) ) ;
#2504=CARTESIAN_POINT ( 'NONE',  ( 21.85643539959777115, 4.792808800112425160, -12.41435969090265523 ) ) ;
#2510=CARTESIAN_POINT ( 'NONE',  ( 86.42578330747443260, 1.280182770620154953, -5.202446006352976937 ) ) ;
#2514=CARTESIAN_POINT ( 'NONE',  ( 14.84236729553075129, -4.537698572362919514, 2.514786686759733048 ) ) ;
#2515=CARTESIAN_POINT ( 'NONE',  ( 21.54943548333990577, 7.328808947467964963, 1.955308278464419347 ) ) ;
#2516=CARTESIAN_POINT ( 'NONE',  ( 34.33397697960574391, -1.483043513302994443, -5.565045496675192993 ) ) ;
#2523=CARTESIAN_POINT ( 'NONE',  ( 36.99646211313889665, -3.220648697242111780, 5.952655130425513974 ) ) ;
#2531=ORIENTED_EDGE ( 'NONE', *, *, #15578, .T. ) ;
#2533=CARTESIAN_POINT ( 'NONE',  ( -77.20907466686004739, -6.116245841690640894, -7.791481786428602341 ) ) ;
#2537=VERTEX_POINT ( 'NONE', #34449 ) ;
#2538=CARTESIAN_POINT ( 'NONE',  ( 22.63321249055432816, 4.548868538501633196, 3.119291088745934637 ) ) ;
#2545=CARTESIAN_POINT ( 'NONE',  ( 27.44076331759783116, 0.9565809941908112179, 4.489197854688308453 ) ) ;
#2546=CARTESIAN_POINT ( 'NONE',  ( 14.75858788393853160, -5.151706771557507558, -2.499999999916640014 ) ) ;
#2556=CARTESIAN_POINT ( 'NONE',  ( -80.92837670882107659, 2.429809908903242555, -12.50000000000000000 ) ) ;
#2558=CARTESIAN_POINT ( 'NONE',  ( 27.86875652909539980, 2.635651561731235493, 0.006556038081918813022 ) ) ;
#2559=CARTESIAN_POINT ( 'NONE',  ( 14.73423124852490318, -5.107548947968362008, -2.500000000000001776 ) ) ;
#2561=CARTESIAN_POINT ( 'NONE',  ( -81.58016648964061801, -5.624404198090563689, 2.451861983733245598 ) ) ;
#2562=CARTESIAN_POINT ( 'NONE',  ( 21.99020519201814849, 0.2365064862963604797, -7.678606242944151283 ) ) ;
#2568=CARTESIAN_POINT ( 'NONE',  ( 33.44571278339331144, -3.711821305012397598, -5.220872097300803816 ) ) ;
#2569=CARTESIAN_POINT ( 'NONE',  ( -61.24591834330252027, -49.47158280949359010, 2.500000000000000000 ) ) ;
#2578=CARTESIAN_POINT ( 'NONE',  ( 20.95047569564395573, 9.633251686941981973, 2.522532965598568211 ) ) ;
#2579=CARTESIAN_POINT ( 'NONE',  ( 22.53785975336948155, 1.420150480624714273, -5.804402300735387321 ) ) ;
#2585=CARTESIAN_POINT ( 'NONE',  ( 86.53727031679849802, -0.6854317443871157378, -5.678301933988063155 ) ) ;
#2597=CARTESIAN_POINT ( 'NONE',  ( 24.42167434069570930, 3.172085603352147842, 3.233354437090341094 ) ) ;
#2599=CARTESIAN_POINT ( 'NONE',  ( 22.15639445573606992, -3.079419702076586329, 3.567612438417096410 ) ) ;
#2603=DIRECTION ( 'NONE',  ( -0.000000000000000000, -0.000000000000000000, -1.000000000000000000 ) ) ;
#2606=ORIENTED_EDGE ( 'NONE', *, *, #8684, .T. ) ;
#2608=DIRECTION ( 'NONE',  ( -0.000000000000000000, -1.000000000000000000, -0.000000000000000000 ) ) ;
#2609=CARTESIAN_POINT ( 'NONE',  ( 21.85643539959776760, 6.468309080218945795, -8.875946301973074881 ) ) ;
#2614=CARTESIAN_POINT ( 'NONE',  ( -72.63917791570506211, 6.521876929970503056, -9.854674157099612586 ) ) ;
#2615=CARTESIAN_POINT ( 'NONE',  ( 29.48920755849628605, -3.189424998377129228, -4.808902057303421351 ) ) ;
#2616=CARTESIAN_POINT ( 'NONE',  ( 36.13397042527238057, -1.528216537091738214, -5.641571063127631014 ) ) ;
#2618=CARTESIAN_POINT ( 'NONE',  ( 15.49758433003794877, 11.04722695288106671, 2.625170863832550605 ) ) ;
#2623=CARTESIAN_POINT ( 'NONE',  ( 19.92985266052819782, 11.61392316146510240, -2.499999999999999556 ) ) ;
#2624=CARTESIAN_POINT ( 'NONE',  ( 37.18189302406424446, -2.607975392620101474, -5.985526701086073764 ) ) ;
#2625=CARTESIAN_POINT ( 'NONE',  ( 24.88192582561759636, 2.551848270425359555, -3.964384284743410092 ) ) ;
#2628=CARTESIAN_POINT ( 'NONE',  ( 36.68763091036087332, -2.387583900041891027, 5.932390115904950356 ) ) ;
#2631=AXIS2_PLACEMENT_3D ( 'NONE', #35079, #25792, #32188 ) ;
#2633=CARTESIAN_POINT ( 'NONE',  ( 86.85482141032015591, 0.6757441427909987031, 5.750446197363288547 ) ) ;
#2636=CARTESIAN_POINT ( 'NONE',  ( 37.01725082149712875, -2.757042412250769292, -5.983835274925594305 ) ) ;
#2657=CARTESIAN_POINT ( 'NONE',  ( 22.01200767717710605, 5.505276828284054069, -3.148064352147821765 ) ) ;
#2661=CARTESIAN_POINT ( 'NONE',  ( 26.66483005201559564, 2.460286195115170216, -3.284910328407702806 ) ) ;
#2665=CARTESIAN_POINT ( 'NONE',  ( 87.02687067233559048, -1.029203037998749570, 5.291918051785640564 ) ) ;
#2673=CARTESIAN_POINT ( 'NONE',  ( 14.89421247541311999, -5.922026149921197913, -2.519984706040779621 ) ) ;
#2674=CARTESIAN_POINT ( 'NONE',  ( 36.64490972802850166, -2.463767798561049549, -5.925722442186287076 ) ) ;
#2675=DIRECTION ( 'NONE',  ( 0.000000000000000000, 0.000000000000000000, -1.000000000000000000 ) ) ;
#2678=CARTESIAN_POINT ( 'NONE',  ( 36.91034452848013814, -2.639964513169326565, 5.967149962361803617 ) ) ;
#2679=CARTESIAN_POINT ( 'NONE',  ( 86.83829259450851623, 0.8168327605515373069, 4.998615091244022146 ) ) ;
#2683=CARTESIAN_POINT ( 'NONE',  ( 37.11018018669391694, -2.403351589215351414, 5.951538865951512491 ) ) ;
#2685=CARTESIAN_POINT ( 'NONE',  ( 18.09051835526576824, -2.859643911663029225, 3.029860928815728549 ) ) ;
#2686=CARTESIAN_POINT ( 'NONE',  ( 14.62858089720442401, 12.62725169013372550, -2.499999999999999556 ) ) ;
#2699=CARTESIAN_POINT ( 'NONE',  ( 24.63365376234076010, 2.464256406091844376, 4.030237559253687429 ) ) ;
#2700=CARTESIAN_POINT ( 'NONE',  ( 21.46987128311033999, 7.825037809131126565, -2.777605031916560829 ) ) ;
#2704=CARTESIAN_POINT ( 'NONE',  ( -70.92837670882012446, 0.2170085631207802901, 6.000000000001379341 ) ) ;
#2709=CARTESIAN_POINT ( 'NONE',  ( 23.24073689758073513, 3.246734186628089880, -3.866034852107397057 ) ) ;
#2711=CARTESIAN_POINT ( 'NONE',  ( 21.85643539959777115, 5.662525507098640887, -13.61651877770312957 ) ) ;
#2712=CARTESIAN_POINT ( 'NONE',  ( 16.09990961988970426, 15.28674628019742343, -3.774899269766144538 ) ) ;
#2716=CARTESIAN_POINT ( 'NONE',  ( 88.68641656676298624, -1.259067802340008146, 0.2042187262504959744 ) ) ;
#2717=DIRECTION ( 'NONE',  ( -0.000000000000000000, -0.000000000000000000, -1.000000000000000000 ) ) ;
#2720=CARTESIAN_POINT ( 'NONE',  ( 31.36708859361117518, -3.142839770289761692, 5.101990809574796337 ) ) ;
#2722=CARTESIAN_POINT ( 'NONE',  ( 34.33342975363300553, -1.484566801286986371, -5.564960088827437978 ) ) ;
#2728=AXIS2_PLACEMENT_3D ( 'NONE', #22101, #24775, #37711 ) ;
#2730=CARTESIAN_POINT ( 'NONE',  ( 36.84734063698446249, -2.123997533844214747, 5.880499845153348559 ) ) ;
#2736=CARTESIAN_POINT ( 'NONE',  ( 88.34928245270404545, -0.8803827640786102693, 0.5788234153557996198 ) ) ;
#2737=CARTESIAN_POINT ( 'NONE',  ( -73.85267074163550660, -3.621953098407464378, -9.567270356371031070 ) ) ;
#2739=CARTESIAN_POINT ( 'NONE',  ( 15.23433789938383320, 11.32867894725656477, 2.584084891689991448 ) ) ;
#2744=CARTESIAN_POINT ( 'NONE',  ( 22.88829950429575533, 4.274613241398780517, 3.138138624598397541 ) ) ;
#2748=EDGE_LOOP ( 'NONE', ( #28656, #3105, #29221, #32948, #5854 ) ) ;
#2761=CARTESIAN_POINT ( 'NONE',  ( 30.56085893896448269, -1.894852608703655017, -5.974852047816421319 ) ) ;
#2766=CARTESIAN_POINT ( 'NONE',  ( 27.32964825819615839, 1.127509148772342762, -4.470608802228491108 ) ) ;
#2771=CARTESIAN_POINT ( 'NONE',  ( -71.59355962058776868, -48.46505220862084684, 9.978265513184469526 ) ) ;
#2772=CARTESIAN_POINT ( 'NONE',  ( 33.67397214766437941, -3.719464542966671949, -5.264060338108396131 ) ) ;
#2778=CARTESIAN_POINT ( 'NONE',  ( -74.72254313616608101, 7.619260614993313752, 10.58017416545770928 ) ) ;
#2779=CARTESIAN_POINT ( 'NONE',  ( 87.04213330793400871, 0.5878691963681514920, -4.891134986362597914 ) ) ;
#2782=CARTESIAN_POINT ( 'NONE',  ( 22.80421717993787567, 1.676252718750713688, -5.327314847823195088 ) ) ;
#2788=CARTESIAN_POINT ( 'NONE',  ( 87.65251942239244443, -2.181810347267220340, 2.926837865475490297 ) ) ;
#2789=CIRCLE ( 'NONE', #25780, 8.080217238368755162 ) ;
#2797=CARTESIAN_POINT ( 'NONE',  ( 23.14564712628083853, 4.056498438990249866, 3.055703889222537661 ) ) ;
#2809=CARTESIAN_POINT ( 'NONE',  ( 21.85643539959777826, -4.710037025930063237, 11.93878138912534226 ) ) ;
#2811=CARTESIAN_POINT ( 'NONE',  ( -71.75745688627573315, 2.666801288543074300, 9.965618436493368648 ) ) ;
#2812=CARTESIAN_POINT ( 'NONE',  ( 36.00450899137167227, -3.689287878764249573, 5.669280554162174468 ) ) ;
#2814=CARTESIAN_POINT ( 'NONE',  ( -80.58960834254915540, 10.55424001629280717, -2.612171128296283396 ) ) ;
#2815=CARTESIAN_POINT ( 'NONE',  ( 29.48024936498151405, -3.085360730154540043, -4.807503914550576241 ) ) ;
#2816=CARTESIAN_POINT ( 'NONE',  ( 37.21202728235306978, -2.743901910341996153, -6.000907511358490432 ) ) ;
#2818=CARTESIAN_POINT ( 'NONE',  ( 14.95701748268968778, 12.36391905844671513, 2.521938411237070632 ) ) ;
#2820=CARTESIAN_POINT ( 'NONE',  ( 28.82542678208081455, -3.983772535877290633, 4.161834042892701646 ) ) ;
#2822=ADVANCED_FACE ( 'NONE', ( #31419 ), #7105, .T. ) ;
#2827=CARTESIAN_POINT ( 'NONE',  ( 23.61982383042622402, 0.4723780055816908519, -5.491273804847549123 ) ) ;
#2828=CARTESIAN_POINT ( 'NONE',  ( 36.84340344443402415, -2.068064908961660731, -5.856630628969484498 ) ) ;
#2829=CARTESIAN_POINT ( 'NONE',  ( 24.52266067897431157, 2.754179337185791887, -3.866659408860876557 ) ) ;
#2832=CARTESIAN_POINT ( 'NONE',  ( 27.48828073121227433, 1.193421157888713946, 4.496609033324144633 ) ) ;
#2835=CARTESIAN_POINT ( 'NONE',  ( 88.77375424906220758, -2.037038645060464503, 1.247452244799444276 ) ) ;
#2837=CARTESIAN_POINT ( 'NONE',  ( 33.33276309746427302, -3.557760156652166383, 5.357383698657358195 ) ) ;
#2838=CARTESIAN_POINT ( 'NONE',  ( 36.65097534261938250, -3.107212338371014848, -5.926669128040790824 ) ) ;
#2840=EDGE_LOOP ( 'NONE', ( #20264, #20844, #34094, #10773 ) ) ;
#2841=CARTESIAN_POINT ( 'NONE',  ( 24.37720413515472018, 2.941578208236205416, 3.719711831669278546 ) ) ;
#2846=ORIENTED_EDGE ( 'NONE', *, *, #34522, .F. ) ;
#2859=CARTESIAN_POINT ( 'NONE',  ( 22.63048122002746965, 4.558493641243840599, -3.110483684673575056 ) ) ;
#2861=FACE_OUTER_BOUND ( 'NONE', #19747, .T. ) ;
#2863=CARTESIAN_POINT ( 'NONE',  ( 25.40259394636483137, -3.746514978370850457, -4.387842602613081233 ) ) ;
#2865=CARTESIAN_POINT ( 'NONE',  ( -81.72866360994999013, -5.611003566215041261, -1.550695278273204414 ) ) ;
#2868=CARTESIAN_POINT ( 'NONE',  ( 87.21044761576042958, -0.9232309944945271685, 5.337239039084527015 ) ) ;
#2872=CARTESIAN_POINT ( 'NONE',  ( -72.27608653515989090, -46.45118525884571881, 9.908840844397285963 ) ) ;
#2874=DIRECTION ( 'NONE',  ( 1.000000000000000000, 0.000000000000000000, 0.000000000000000000 ) ) ;
#2875=CARTESIAN_POINT ( 'NONE',  ( 14.99834168678628821, -6.074323333651953760, -2.528087544903816042 ) ) ;
#2879=CARTESIAN_POINT ( 'NONE',  ( 33.62692633095992534, -1.233801386824908697, 5.454693142869670552 ) ) ;
#2881=CARTESIAN_POINT ( 'NONE',  ( 86.23508606437836477, 1.494382965102754923, 4.690504771849753674 ) ) ;
#2884=CARTESIAN_POINT ( 'NONE',  ( 14.61802081865033820, -4.461849342347350422, 2.500000000000000000 ) ) ;
#2887=CARTESIAN_POINT ( 'NONE',  ( 22.12814134479806327, -2.652490312909201009, 3.660029646613253362 ) ) ;
#2891=CARTESIAN_POINT ( 'NONE',  ( 27.39224238248323928, -4.425241401586402112, -3.685821984149812547 ) ) ;
#2897=VERTEX_POINT ( 'NONE', #31621 ) ;
#2898=CARTESIAN_POINT ( 'NONE',  ( 22.94192414811271874, 2.589169918962352934, 4.530654349547726945 ) ) ;
#2905=CARTESIAN_POINT ( 'NONE',  ( -70.66670089265474530, 0.1910294010741415138, 5.995519781525873171 ) ) ;
#2906=CARTESIAN_POINT ( 'NONE',  ( 86.41267556467273891, 1.294906009465945695, -4.859934084155808520 ) ) ;
#2909=VERTEX_POINT ( 'NONE', #28525 ) ;
#2910=CARTESIAN_POINT ( 'NONE',  ( 22.87293662167099484, 3.020083017603196751, -4.246090233063728903 ) ) ;
#2913=CARTESIAN_POINT ( 'NONE',  ( 21.85643539959776760, 8.744094842958308078, -10.51782716378651550 ) ) ;
#2915=FACE_OUTER_BOUND ( 'NONE', #13802, .T. ) ;
#2919=CARTESIAN_POINT ( 'NONE',  ( 88.25065740119208613, -0.7696024251930051463, 2.713887439742028285 ) ) ;
#2923=CARTESIAN_POINT ( 'NONE',  ( 14.70875212460786585, -5.604200338437857809, 2.501448141494666544 ) ) ;
#2928=CARTESIAN_POINT ( 'NONE',  ( 36.14168653043503809, -3.145492948648968667, -5.847182291702903711 ) ) ;
#2932=CARTESIAN_POINT ( 'NONE',  ( 21.95193868331012155, 4.960489846753153742, -3.632506201283221881 ) ) ;
#2938=CARTESIAN_POINT ( 'NONE',  ( 36.71867153785819937, -3.456726483225898594, 5.861373841279237773 ) ) ;
#2942=CARTESIAN_POINT ( 'NONE',  ( 87.43068102542478925, -1.906665703887821417, -3.819564193719649392 ) ) ;
#2946=CARTESIAN_POINT ( 'NONE',  ( -79.61006498529616238, -6.642554117411252790, -4.980146162474928140 ) ) ;
#2952=CARTESIAN_POINT ( 'NONE',  ( 22.20283045833796365, 5.199714587881895334, 3.119843736163353309 ) ) ;
#2957=ORIENTED_EDGE ( 'NONE', *, *, #17175, .T. ) ;
#2961=CARTESIAN_POINT ( 'NONE',  ( 17.19129603292001818, 9.338074606371669972, -2.827989852679653637 ) ) ;
#2971=CARTESIAN_POINT ( 'NONE',  ( 32.04447592720433136, -5.114560573210904515, 0.4782324236124577688 ) ) ;
#2975=CARTESIAN_POINT ( 'NONE',  ( 27.29033202111899570, 1.163606810116843082, -4.463626990047735887 ) ) ;
#2984=CARTESIAN_POINT ( 'NONE',  ( 33.88299691088344190, -0.6033410658551250361, -5.261223570660462201 ) ) ;
#2992=VECTOR ( 'NONE', #23154, 1000.000000000000000 ) ;
#2993=CARTESIAN_POINT ( 'NONE',  ( 14.76635595020048086, -4.521629488604276048, -2.511015163609813250 ) ) ;
#2997=EDGE_LOOP ( 'NONE', ( #12758, #22042, #7381, #30565 ) ) ;
#2998=FACE_OUTER_BOUND ( 'NONE', #35857, .T. ) ;
#3007=ORIENTED_EDGE ( 'NONE', *, *, #4349, .F. ) ;
#3008=CARTESIAN_POINT ( 'NONE',  ( 22.61636450491116079, 4.630129225324790987, 3.032335577038935526 ) ) ;
#3011=VERTEX_POINT ( 'NONE', #1354 ) ;
#3021=CARTESIAN_POINT ( 'NONE',  ( 21.85643539959777826, -3.517407513333692837, -12.34883488727242806 ) ) ;
#3024=CARTESIAN_POINT ( 'NONE',  ( -73.53826198524987490, 5.721180179705736002, 10.86979427268231646 ) ) ;
#3025=DIRECTION ( 'NONE',  ( -0.000000000000000000, -1.000000000000000000, 0.000000000000000000 ) ) ;
#3031=CARTESIAN_POINT ( 'NONE',  ( 31.99223528116318960, -3.505258990368231409, -5.093870457845899757 ) ) ;
#3032=CARTESIAN_POINT ( 'NONE',  ( 35.83255119622532447, -3.731021559448283842, -5.622473652077308870 ) ) ;
#3034=CARTESIAN_POINT ( 'NONE',  ( 14.62015730672339231, 13.26385897396263402, 2.488227156191563427 ) ) ;
#3036=CARTESIAN_POINT ( 'NONE',  ( 29.91572391670933939, -3.747096582641243234, 4.516102143398081026 ) ) ;
#3039=CARTESIAN_POINT ( 'NONE',  ( 22.71381320255807168, 0.3598457172671483684, -6.352659116514114856 ) ) ;
#3040=CARTESIAN_POINT ( 'NONE',  ( 30.95657945650521370, -3.766297307885082546, -4.594095185586652974 ) ) ;
#3041=CARTESIAN_POINT ( 'NONE',  ( 25.18369925879074600, 2.393806484869988704, -4.034630338149852058 ) ) ;
#3044=CARTESIAN_POINT ( 'NONE',  ( 25.38651582566222231, 1.982134986759825246, 4.168577788436554243 ) ) ;
#3049=CARTESIAN_POINT ( 'NONE',  ( 85.39132736373097998, 1.761725527925377399, -5.190388716534374502 ) ) ;
#3051=CARTESIAN_POINT ( 'NONE',  ( 36.94799853101055476, -2.665675819573480432, -5.973026780122190793 ) ) ;
#3053=CARTESIAN_POINT ( 'NONE',  ( 24.38485034621638192, 2.855400732331458080, 3.806845948903719634 ) ) ;
#3056=AXIS2_PLACEMENT_3D ( 'NONE', #11972, #24550, #34052 ) ;
#3060=ORIENTED_EDGE ( 'NONE', *, *, #38073, .T. ) ;
#3072=CARTESIAN_POINT ( 'NONE',  ( 23.36039791900657292, -7.521532571658541499, 2.500000000000001332 ) ) ;
#3074=CARTESIAN_POINT ( 'NONE',  ( 33.88948527724345183, -5.411818363456161407, -1.181565996586838363 ) ) ;
#3075=CARTESIAN_POINT ( 'NONE',  ( 23.42457730801429250, 3.736864044906049287, -3.223246337197901212 ) ) ;
#3077=CARTESIAN_POINT ( 'NONE',  ( -76.86283903552966024, -4.590577806607137212, -8.068255941560765976 ) ) ;
#3081=CARTESIAN_POINT ( 'NONE',  ( 84.20866968570335587, 3.050835305001676101, 0.3231758755354003920 ) ) ;
#3087=AXIS2_PLACEMENT_3D ( 'NONE', #26295, #10224, #16595 ) ;
#3094=CARTESIAN_POINT ( 'NONE',  ( 22.91933054147514781, 2.648295867847167084, 3.783513855737346443 ) ) ;
#3096=CARTESIAN_POINT ( 'NONE',  ( -4.266520354791871306, -48.67644278316300444, 2.500000000000000000 ) ) ;
#3105=ORIENTED_EDGE ( 'NONE', *, *, #12178, .T. ) ;
#3109=CARTESIAN_POINT ( 'NONE',  ( 34.16819525005292491, -3.144580783072454810, 5.539171248332353414 ) ) ;
#3110=EDGE_CURVE ( 'NONE', #2909, #32120, #34138, .T. ) ;
#3113=CARTESIAN_POINT ( 'NONE',  ( 22.25424755511076214, 2.880317739159906854, 4.805666700857594620 ) ) ;
#3114=CARTESIAN_POINT ( 'NONE',  ( 36.09558223311753267, -1.516586179111547361, 5.636573198050853328 ) ) ;
#3120=AXIS2_PLACEMENT_3D ( 'NONE', #24190, #36749, #29962 ) ;
#3122=CARTESIAN_POINT ( 'NONE',  ( 8.290806648384990041, 0.000000000000000000, -2.500000000000000000 ) ) ;
#3128=CARTESIAN_POINT ( 'NONE',  ( 23.92392269211408617, 2.966294017613217981, -3.818242420704017537 ) ) ;
#3129=CARTESIAN_POINT ( 'NONE',  ( 21.85643539959775339, 7.579478879252558698, 11.98046644763472024 ) ) ;
#3135=CARTESIAN_POINT ( 'NONE',  ( 86.01579553793663990, 1.740700492558412193, -4.743980989581940477 ) ) ;
#3138=CARTESIAN_POINT ( 'NONE',  ( 23.84092335974494148, -2.965170422622688040, 3.897202789918388977 ) ) ;
#3140=CARTESIAN_POINT ( 'NONE',  ( 33.46241809521923471, -3.087400495052112781, -5.429017654035560803 ) ) ;
#3143=AXIS2_PLACEMENT_3D ( 'NONE', #25763, #7221, #859 ) ;
#3153=CARTESIAN_POINT ( 'NONE',  ( 87.67937458983125509, -2.214055474509613930, -2.742479142822641602 ) ) ;
#3156=CARTESIAN_POINT ( 'NONE',  ( -74.78824586187189993, 9.457194952391420273, -9.226500222781202964 ) ) ;
#3161=ORIENTED_EDGE ( 'NONE', *, *, #7055, .F. ) ;
#3162=CARTESIAN_POINT ( 'NONE',  ( 21.83976307972709918, 5.907766738269700113, 3.159785223916961705 ) ) ;
#3173=CARTESIAN_POINT ( 'NONE',  ( 17.10588945481550383, 9.262888318566355750, -2.855260069168449988 ) ) ;
#3184=CARTESIAN_POINT ( 'NONE',  ( 32.03962978398497796, -5.076534887360421244, -0.9488177176524058565 ) ) ;
#3185=CARTESIAN_POINT ( 'NONE',  ( -12.99139449055068596, 10.37661300689600097, 6.000000000000000000 ) ) ;
#3186=CARTESIAN_POINT ( 'NONE',  ( 24.20305058822417266, -8.556106420403189361, 2.499999999999995115 ) ) ;
#3192=CARTESIAN_POINT ( 'NONE',  ( 23.31574928852108286, 3.489132783961883533, -3.362529947468282820 ) ) ;
#3201=CARTESIAN_POINT ( 'NONE',  ( 22.03054732944672267, -11.55401157302784121, 2.500000000000000000 ) ) ;
#3203=DIRECTION ( 'NONE',  ( 1.000000000000000000, 0.000000000000000000, 0.000000000000000000 ) ) ;
#3206=ORIENTED_EDGE ( 'NONE', *, *, #18499, .F. ) ;
#3213=CARTESIAN_POINT ( 'NONE',  ( 23.75242797775258197, 3.571880847392433722, 3.151661273409955832 ) ) ;
#3214=EDGE_CURVE ( 'NONE', #21048, #17583, #11200, .T. ) ;
#3216=CARTESIAN_POINT ( 'NONE',  ( 18.04466435519415768, -3.159710396077179517, 2.979303362740127081 ) ) ;
#3217=ORIENTED_EDGE ( 'NONE', *, *, #18879, .F. ) ;
#3218=EDGE_CURVE ( 'NONE', #39042, #34269, #36079, .T. ) ;
#3223=CARTESIAN_POINT ( 'NONE',  ( 22.00621292889270819, 0.2476518612282572751, 7.633907389783355590 ) ) ;
#3229=CARTESIAN_POINT ( 'NONE',  ( 21.85643539959779957, 2.883972393613821072, 11.80804406839454046 ) ) ;
#3232=CARTESIAN_POINT ( 'NONE',  ( -74.60456144785419497, 9.286899217492273095, 9.301175053638090162 ) ) ;
#3233=CARTESIAN_POINT ( 'NONE',  ( 37.06055832016893703, -3.177318995967190585, 5.963242555153861701 ) ) ;
#3238=CARTESIAN_POINT ( 'NONE',  ( -81.11237078102703890, 10.50958725180905873, -4.125641042171466211 ) ) ;
#3240=CARTESIAN_POINT ( 'NONE',  ( 20.92112071914918303, 4.582339863481973197, -2.646876999278094278 ) ) ;
#3242=CARTESIAN_POINT ( 'NONE',  ( 20.81473064669264161, 6.282592952945772247, 3.335602345720931172 ) ) ;
#3247=CARTESIAN_POINT ( 'NONE',  ( 23.18753022366955108, 0.6683388799240479461, -5.710891331619152744 ) ) ;
#3248=CARTESIAN_POINT ( 'NONE',  ( 28.66920249112477848, -4.024975064351027143, -4.110187144531254333 ) ) ;
#3250=CARTESIAN_POINT ( 'NONE',  ( 26.62467638871712339, 1.621415574385618008, -4.335577499637811805 ) ) ;
#3253=CARTESIAN_POINT ( 'NONE',  ( 37.06592056232945254, -2.656377846863923864, 5.990200015405097389 ) ) ;
#3255=CARTESIAN_POINT ( 'NONE',  ( 86.42495861400665547, -0.1300389677119091758, -5.942483626122943896 ) ) ;
#3256=CARTESIAN_POINT ( 'NONE',  ( 21.58863229896841673, 7.203270328900314823, 2.924123313244538558 ) ) ;
#3258=CARTESIAN_POINT ( 'NONE',  ( 25.63475025744274305, 2.159471803233731446, 4.132560422135860279 ) ) ;
#3262=ORIENTED_EDGE ( 'NONE', *, *, #30791, .T. ) ;
#3269=CARTESIAN_POINT ( 'NONE',  ( 14.68065631944699412, 12.91438177319650649, 2.499999999999999556 ) ) ;
#3270=ORIENTED_EDGE ( 'NONE', *, *, #36036, .F. ) ;
#3271=ORIENTED_EDGE ( 'NONE', *, *, #40629, .T. ) ;
#3277=DIRECTION ( 'NONE',  ( 0.000000000000000000, -0.000000000000000000, -1.000000000000000000 ) ) ;
#3278=CARTESIAN_POINT ( 'NONE',  ( 14.66962918947507788, -4.461849342347338876, 2.500000000000000000 ) ) ;
#3279=CARTESIAN_POINT ( 'NONE',  ( 22.87815214592131952, 4.326272378261545981, -3.076133176055316554 ) ) ;
#3284=FACE_OUTER_BOUND ( 'NONE', #20019, .T. ) ;
#3287=CARTESIAN_POINT ( 'NONE',  ( 87.93534175303985023, -2.522256948347837202, 0.2133659395812929627 ) ) ;
#3288=DIRECTION ( 'NONE',  ( -0.000000000000000000, -1.000000000000000000, -0.000000000000000000 ) ) ;
#3291=CARTESIAN_POINT ( 'NONE',  ( 14.61802081865033287, 12.33286846116284252, -3.500000000000000000 ) ) ;
#3292=ADVANCED_FACE ( 'NONE', ( #30917 ), #17501, .T. ) ;
#3298=B_SPLINE_SURFACE_WITH_KNOTS ( 'NONE', 5, 3, ( 
 ( #24220, #33711, #19163, #22270, #10290, #3951, #12984 ),
 ( #3543, #13378, #28635, #35637, #35437, #38089, #847 ),
 ( #16656, #35037, #10091, #1054, #19369, #16269, #32151 ),
 ( #32347, #13586, #28841, #18958, #38289, #22469, #38690 ),
 ( #25956, #19576, #22674, #31727, #19772, #10488, #6613 ),
 ( #38487, #22868, #231, #16470, #23069, #34838, #4142 ),
 ( #25344, #35238, #3744, #16069, #29042, #649, #13185 ),
 ( #440, #37882, #31524, #9692, #28424, #7208, #9892 ) ),
 .UNSPECIFIED., .F., .F., .F.,
 ( 6, 2, 6 ),
 ( 4, 1, 1, 1, 4 ),
 ( 0.000000000000000000, 0.5000000000000000000, 1.000000000000000000 ),
 ( 0.000000000000000000, 0.001661007895493813585, 0.002768346492489689309, 0.004010280040507323805, 0.005386808539546716207 ),
 .UNSPECIFIED. ) ;
#3299=CARTESIAN_POINT ( 'NONE',  ( 33.46282145848507383, -3.084177183246969545, 5.429080608628573223 ) ) ;
#3301=CARTESIAN_POINT ( 'NONE',  ( 88.50738123939095203, -1.057966825106399389, -0.8062500484416172952 ) ) ;
#3307=EDGE_LOOP ( 'NONE', ( #7824, #7820, #36129, #32335, #26174, #34431, #38908, #39568 ) ) ;
#3310=CARTESIAN_POINT ( 'NONE',  ( -71.75880299933005801, 2.675120194517714989, 9.965498832022653630 ) ) ;
#3315=CARTESIAN_POINT ( 'NONE',  ( 35.98118923361300858, -3.154045095838573953, 5.822132806892088119 ) ) ;
#3316=CARTESIAN_POINT ( 'NONE',  ( 22.48367044534919401, 2.651248834843010549, 4.808582237203087750 ) ) ;
#3317=CARTESIAN_POINT ( 'NONE',  ( 20.40287464304303100, 10.75613383955523616, -2.500000000000000000 ) ) ;
#3318=ORIENTED_EDGE ( 'NONE', *, *, #13134, .T. ) ;
#3319=ORIENTED_EDGE ( 'NONE', *, *, #22977, .T. ) ;
#3322=CARTESIAN_POINT ( 'NONE',  ( -16.27783086239806210, 25.90100547710869705, -2.500000000000000000 ) ) ;
#3323=CARTESIAN_POINT ( 'NONE',  ( 85.62084935951537545, 2.184322785437529557, -3.437511279438954404 ) ) ;
#3328=CARTESIAN_POINT ( 'NONE',  ( 23.20847637278877684, 3.432400490018996386, -3.727618341475917862 ) ) ;
#3331=CARTESIAN_POINT ( 'NONE',  ( 21.85643539959777826, -5.920441741711214512, 15.33489310402742234 ) ) ;
#3336=CARTESIAN_POINT ( 'NONE',  ( 88.48259847388298738, -1.030129646626848361, 1.133857545573457415 ) ) ;
#3339=CARTESIAN_POINT ( 'NONE',  ( 33.10913737875220875, -3.231866217708247113, 5.373879654101829217 ) ) ;
#3340=CARTESIAN_POINT ( 'NONE',  ( 36.99286102142031751, -2.718909609684730722, -5.980028656754092786 ) ) ;
#3343=ADVANCED_FACE ( 'NONE', ( #11328, #15246 ), #40158, .T. ) ;
#3351=ORIENTED_EDGE ( 'NONE', *, *, #12414, .F. ) ;
#3352=CARTESIAN_POINT ( 'NONE',  ( 23.38445204029254398, 3.558657874120639164, 3.098095084708739400 ) ) ;
#3353=DIRECTION ( 'NONE',  ( 1.000000000000000000, 7.232507224765808510E-18, 0.000000000000000000 ) ) ;
#3361=CYLINDRICAL_SURFACE ( 'NONE', #3143, 10.00000000000000888 ) ;
#3363=ORIENTED_EDGE ( 'NONE', *, *, #8317, .T. ) ;
#3374=CARTESIAN_POINT ( 'NONE',  ( 14.95724209851752917, 12.36297077192868166, -2.521965761379588056 ) ) ;
#3377=VERTEX_POINT ( 'NONE', #17918 ) ;
#3382=DIRECTION ( 'NONE',  ( -0.000000000000000000, 0.000000000000000000, 1.000000000000000000 ) ) ;
#3383=CARTESIAN_POINT ( 'NONE',  ( 17.53685866850469566, 11.96893695421128001, 2.499999999999993339 ) ) ;
#3384=CARTESIAN_POINT ( 'NONE',  ( 30.81316972100007590, -2.191302700533721115, -5.899179390191041428 ) ) ;
#3385=FACE_OUTER_BOUND ( 'NONE', #12096, .T. ) ;
#3395=CARTESIAN_POINT ( 'NONE',  ( 37.07815259682215014, -3.092164982993939049, -5.980626158107812174 ) ) ;
#3405=CARTESIAN_POINT ( 'NONE',  ( 0.7201709579117279159, -51.60714625320436255, -2.500000000000000000 ) ) ;
#3407=LINE ( 'NONE', #12829, #3475 ) ;
#3409=CIRCLE ( 'NONE', #26389, 24.28220113893567245 ) ;
#3411=CARTESIAN_POINT ( 'NONE',  ( 27.43879754216082389, 0.9604377377020558715, 4.488885984917203587 ) ) ;
#3412=CARTESIAN_POINT ( 'NONE',  ( 21.85643539959777115, -15.24623503193425123, 0.9260495571226281530 ) ) ;
#3413=CARTESIAN_POINT ( 'NONE',  ( 22.03446123967401959, 3.769041528266752206, 4.324542679607210616 ) ) ;
#3417=CARTESIAN_POINT ( 'NONE',  ( 24.06586850339645878, 3.348230022213010137, 3.208720231193612715 ) ) ;
#3421=EDGE_LOOP ( 'NONE', ( #32964, #17783, #23479, #38870 ) ) ;
#3423=CARTESIAN_POINT ( 'NONE',  ( 27.24538128678662829, 1.201849171105237479, 4.455454704251525122 ) ) ;
#3431=CARTESIAN_POINT ( 'NONE',  ( 23.92272977471906614, 4.146422156947720872, -1.204255912843045229 ) ) ;
#3434=CARTESIAN_POINT ( 'NONE',  ( -73.70785857967193522, 6.078230591424796714, 10.83945126441197182 ) ) ;
#3435=CARTESIAN_POINT ( 'NONE',  ( 22.59972090504111719, 0.2729357358632942265, -6.520420251158410174 ) ) ;
#3436=ORIENTED_EDGE ( 'NONE', *, *, #18496, .F. ) ;
#3439=CARTESIAN_POINT ( 'NONE',  ( 33.44004484032286229, -3.434887717533713580, -5.408154456503273977 ) ) ;
#3440=CARTESIAN_POINT ( 'NONE',  ( 34.79230701455888664, -3.834676760299985165, -5.377510354588529218 ) ) ;
#3450=CARTESIAN_POINT ( 'NONE',  ( 26.04966261679769346, 1.457184003380286530, -4.328181559151514257 ) ) ;
#3451=CARTESIAN_POINT ( 'NONE',  ( 37.19960550959731194, -2.818616413669091880, -5.999884395390916225 ) ) ;
#3454=ORIENTED_EDGE ( 'NONE', *, *, #18673, .T. ) ;
#3457=CARTESIAN_POINT ( 'NONE',  ( 87.44477293306643162, -1.228341977218806447, 4.926563918429203603 ) ) ;
#3458=CARTESIAN_POINT ( 'NONE',  ( 36.75914032014244270, -2.518819990878720994, -5.943550888763135198 ) ) ;
#3460=CARTESIAN_POINT ( 'NONE',  ( 24.39461023293930708, 2.846075433827604861, 3.813165204976378231 ) ) ;
#3462=ORIENTED_EDGE ( 'NONE', *, *, #26675, .T. ) ;
#3472=CARTESIAN_POINT ( 'NONE',  ( 22.88456325795406698, 4.291280149456187409, -3.119280959484842075 ) ) ;
#3475=VECTOR ( 'NONE', #38338, 1000.000000000000000 ) ;
#3479=CARTESIAN_POINT ( 'NONE',  ( -80.68571131495720294, -5.697267497185621643, -2.227797487936516774 ) ) ;
#3482=DIRECTION ( 'NONE',  ( 0.6159927814537400348, 0.7877517966954343809, -0.000000000000000000 ) ) ;
#3484=CARTESIAN_POINT ( 'NONE',  ( 87.12371845299759343, -1.516527252418922833, -4.675789953527256237 ) ) ;
#3485=CARTESIAN_POINT ( 'NONE',  ( 21.67219544786406260, 6.675102098148268936, -3.070833163645317221 ) ) ;
#3496=CARTESIAN_POINT ( 'NONE',  ( 30.51435440191163195, -0.1427370434214647044, 4.968901015505058361 ) ) ;
#3497=CARTESIAN_POINT ( 'NONE',  ( 86.96272348114096928, 0.6770660828398197273, -5.145113290124521122 ) ) ;
#3502=CARTESIAN_POINT ( 'NONE',  ( 21.63674184841064019, 6.916893520949614071, -2.999760302877421125 ) ) ;
#3506=CARTESIAN_POINT ( 'NONE',  ( -72.89233069014277078, -2.171328805845720300, 9.806946677974712756 ) ) ;
#3512=CARTESIAN_POINT ( 'NONE',  ( 22.03874921663882347, 2.012712906550705227, 5.777197709026360428 ) ) ;
#3513=CARTESIAN_POINT ( 'NONE',  ( 36.44317183454039366, -1.735355048105241549, 5.732832347747111257 ) ) ;
#3519=CARTESIAN_POINT ( 'NONE',  ( 85.76835188082283423, 2.018640952613007578, 3.843583708408826904 ) ) ;
#3523=CARTESIAN_POINT ( 'NONE',  ( 22.98570178199580738, 3.657932872642362998, -3.680547506993712581 ) ) ;
#3525=CARTESIAN_POINT ( 'NONE',  ( 21.85643539959773207, -2.370478073490382531, -12.58538558043069600 ) ) ;
#3527=CARTESIAN_POINT ( 'NONE',  ( 16.09990961988968294, 15.28674628019743942, 3.774899269766986531 ) ) ;
#3530=CARTESIAN_POINT ( 'NONE',  ( 85.43834401013396018, 2.333645700298356829, -4.102255839672300120 ) ) ;
#3532=CARTESIAN_POINT ( 'NONE',  ( -81.82396199936634673, -5.600653810444165437, 0.2120607140719947270 ) ) ;
#3533=CARTESIAN_POINT ( 'NONE',  ( 33.95295690078342687, -3.700853304509699182, 5.336167209958794899 ) ) ;
#3535=CARTESIAN_POINT ( 'NONE',  ( 27.40776759654589156, 0.9655315125819244892, -4.484043011441926296 ) ) ;
#3538=CARTESIAN_POINT ( 'NONE',  ( -75.86661230596840255, -3.880840061887903758, 10.12747849425165647 ) ) ;
#3543=CARTESIAN_POINT ( 'NONE',  ( 33.45304404609620263, -3.772033185430891500, 5.158132413726952414 ) ) ;
#3544=ORIENTED_EDGE ( 'NONE', *, *, #35578, .F. ) ;
#3546=CARTESIAN_POINT ( 'NONE',  ( 36.68438008943704887, -1.916626965623605683, 5.804116225272221818 ) ) ;
#3547=LINE ( 'NONE', #25755, #31053 ) ;
#3553=DIRECTION ( 'NONE',  ( 1.000000000000000000, 0.000000000000000000, 0.000000000000000000 ) ) ;
#3555=CARTESIAN_POINT ( 'NONE',  ( -70.92837670882107659, -23.80776546975053165, 10.00000000000001066 ) ) ;
#3557=CARTESIAN_POINT ( 'NONE',  ( 23.70115564627849736, 3.489872147238937128, 3.358116645522415844 ) ) ;
#3563=CARTESIAN_POINT ( 'NONE',  ( -71.41272068158380648, -45.69399732294015593, 5.981110394793661023 ) ) ;
#3565=CARTESIAN_POINT ( 'NONE',  ( 17.35526930789154676, 8.837536743741704726, -2.915107532907570853 ) ) ;
#3578=CARTESIAN_POINT ( 'NONE',  ( 17.42606411499827601, 12.01804255755900463, 2.499999999999993339 ) ) ;
#3579=CARTESIAN_POINT ( 'NONE',  ( 29.64656804624054942, -2.931097914703496787, 5.165983120431130615 ) ) ;
#3582=CIRCLE ( 'NONE', #34496, 9.386006772603931125 ) ;
#3589=CARTESIAN_POINT ( 'NONE',  ( 33.75541762379567245, -0.8753173094601959248, -5.454573668235052963 ) ) ;
#3595=DIRECTION ( 'NONE',  ( -0.9594800004753906153, -0.2817767355331954326, 0.000000000000000000 ) ) ;
#3596=CARTESIAN_POINT ( 'NONE',  ( 22.02701111391718314, -11.57978826329849475, 2.500000000000000444 ) ) ;
#3597=CARTESIAN_POINT ( 'NONE',  ( 8.290806648384990041, -35.94265729135299381, -6.000000000000000000 ) ) ;
#3602=CIRCLE ( 'NONE', #30524, 27.95745752244933158 ) ;
#3605=CARTESIAN_POINT ( 'NONE',  ( 30.79191905210313251, -3.554283433601253428, 4.832056180595072803 ) ) ;
#3606=CARTESIAN_POINT ( 'NONE',  ( 22.23240669476004783, 3.462061741365346279, 4.374547872445481822 ) ) ;
#3617=CARTESIAN_POINT ( 'NONE',  ( 21.81113558402230268, 0.2595215699418438327, 8.250542685949572075 ) ) ;
#3628=CARTESIAN_POINT ( 'NONE',  ( 24.87384391889476021, -2.282154821806516409, -6.307558310060713325 ) ) ;
#3630=CARTESIAN_POINT ( 'NONE',  ( -77.28818573224673116, 9.645729766875481559, 9.280166210047219977 ) ) ;
#3631=CARTESIAN_POINT ( 'NONE',  ( 23.05078809043722643, 0.3400200871709115336, -5.963306588542081066 ) ) ;
#3636=CARTESIAN_POINT ( 'NONE',  ( 29.60526006017712319, -3.794915248219668857, -4.412248584793623252 ) ) ;
#3637=CARTESIAN_POINT ( 'NONE',  ( 29.48812867847481556, 1.219306054872145273, -4.222749534284976569 ) ) ;
#3639=CARTESIAN_POINT ( 'NONE',  ( 15.98747256189193777, 10.21191258246141587, 2.701629770405024722 ) ) ;
#3643=CARTESIAN_POINT ( 'NONE',  ( 21.58862418887968460, 7.202556094215188054, 2.923978954502209682 ) ) ;
#3644=CARTESIAN_POINT ( 'NONE',  ( 24.05048767930056641, 0.8437649274697022195, -5.043273178371332932 ) ) ;
#3645=CARTESIAN_POINT ( 'NONE',  ( 36.43378600387098487, -1.733243984275257166, -5.730557465163646391 ) ) ;
#3647=ORIENTED_EDGE ( 'NONE', *, *, #7287, .F. ) ;
#3650=CARTESIAN_POINT ( 'NONE',  ( 87.89980060869044109, -1.794189136469996004, 3.743635721206352684 ) ) ;
#3651=ORIENTED_EDGE ( 'NONE', *, *, #40468, .T. ) ;
#3652=CARTESIAN_POINT ( 'NONE',  ( 24.37736685700319939, 2.941625658114979558, 3.719599273349688762 ) ) ;
#3670=AXIS2_PLACEMENT_3D ( 'NONE', #28952, #13288, #38399 ) ;
#3675=CARTESIAN_POINT ( 'NONE',  ( 33.88049027533028124, -5.353668869269942121, -1.604319996572373785 ) ) ;
#3676=CARTESIAN_POINT ( 'NONE',  ( 24.38812970663561330, 3.155185924440667478, -3.309899503823893419 ) ) ;
#3680=CARTESIAN_POINT ( 'NONE',  ( -81.80090188080515645, -5.603160304130403446, -0.6545554231109701471 ) ) ;
#3682=CARTESIAN_POINT ( 'NONE',  ( -61.24591834330252027, -49.47158280949359010, -2.500000000000000000 ) ) ;
#3685=CARTESIAN_POINT ( 'NONE',  ( 22.22910988738226834, 4.118587929658937163, -2.394959132921147038 ) ) ;
#3687=CARTESIAN_POINT ( 'NONE',  ( 21.56937222159085010, 7.264334593773944526, -2.455214307437531662 ) ) ;
#3688=CARTESIAN_POINT ( 'NONE',  ( 35.48433445138798703, -1.920574954861675065, 5.744586601647555746 ) ) ;
#3697=CARTESIAN_POINT ( 'NONE',  ( 36.89747129275986026, -3.002612578834559898, 5.965140782587297075 ) ) ;
#3700=CARTESIAN_POINT ( 'NONE',  ( 85.17359253740836778, 2.686702876117401662, 1.784494502703901864 ) ) ;
#3703=CARTESIAN_POINT ( 'NONE',  ( 25.73532669649552318, 2.638944299754048206, 3.514017186027001305 ) ) ;
#3704=CARTESIAN_POINT ( 'NONE',  ( -69.58021497804521971, -46.45211564195850684, 9.908779002578803841 ) ) ;
#3707=VERTEX_POINT ( 'NONE', #16652 ) ;
#3708=CARTESIAN_POINT ( 'NONE',  ( -75.70508440899935465, -5.314284899882218305, 8.787320279435890669 ) ) ;
#3714=CARTESIAN_POINT ( 'NONE',  ( 23.51831161216184185, 2.310449087985749106, 4.435690330918023783 ) ) ;
#3717=AXIS2_PLACEMENT_3D ( 'NONE', #39855, #20703, #7943 ) ;
#3721=CARTESIAN_POINT ( 'NONE',  ( 86.35258271375249706, 1.362405151798338654, 4.807923594896911013 ) ) ;
#3724=CARTESIAN_POINT ( 'NONE',  ( 22.99674145141367987, 3.564721660139269055, -3.751998251592491229 ) ) ;
#3727=ORIENTED_EDGE ( 'NONE', *, *, #12696, .F. ) ;
#3728=CARTESIAN_POINT ( 'NONE',  ( 21.85643539959781023, -9.626920734992143736, 7.250399157909895642 ) ) ;
#3729=CARTESIAN_POINT ( 'NONE',  ( 18.05491602129117013, 13.75800355182912682, 1.937621434239656715 ) ) ;
#3732=CARTESIAN_POINT ( 'NONE',  ( 88.92600529607371129, -1.724176122391732680, 0.2146816905789898644 ) ) ;
#3733=ORIENTED_EDGE ( 'NONE', *, *, #992, .T. ) ;
#3734=FACE_OUTER_BOUND ( 'NONE', #27206, .T. ) ;
#3735=CARTESIAN_POINT ( 'NONE',  ( 33.95122966076780102, -3.129518407428083737, 5.505308520791801996 ) ) ;
#3736=CARTESIAN_POINT ( 'NONE',  ( 37.03092461603053209, -2.782178920321524807, 5.985969401264504164 ) ) ;
#3737=CARTESIAN_POINT ( 'NONE',  ( 29.53482198975021333, -3.874005733230891035, 4.296914696760256724 ) ) ;
#3738=CARTESIAN_POINT ( 'NONE',  ( 31.71901687615503462, -0.5584438621182004070, -5.156917729482751511 ) ) ;
#3744=CARTESIAN_POINT ( 'NONE',  ( 32.00563084067037067, -3.049499025779075723, 5.201650770433705162 ) ) ;
#3747=CARTESIAN_POINT ( 'NONE',  ( 36.87053919822349002, -2.087953330798700602, 5.864521777571895633 ) ) ;
#3752=CARTESIAN_POINT ( 'NONE',  ( 86.88071486596068382, -1.182640904908754731, -5.180176386390026089 ) ) ;
#3755=SHAPE_REPRESENTATION_RELATIONSHIP ( 'NONE' , 'NONE' ,  #131, #15661 ) ;
#3758=DIRECTION ( 'NONE',  ( 0.000000000000000000, -1.000000000000000000, 0.000000000000000000 ) ) ;
#3759=EDGE_LOOP ( 'NONE', ( #4328, #25731, #16849, #10299, #17163, #15560, #868 ) ) ;
#3767=CARTESIAN_POINT ( 'NONE',  ( 15.64686839187730349, 11.13536136061385307, -2.614792074122313181 ) ) ;
#3774=AXIS2_PLACEMENT_3D ( 'NONE', #6293, #21327, #18218 ) ;
#3779=CARTESIAN_POINT ( 'NONE',  ( 16.68329392019911595, 9.858079660169737579, 2.499999999999976463 ) ) ;
#3780=CARTESIAN_POINT ( 'NONE',  ( 27.77988552260176291, -0.3358138158918914651, -6.029166980063449088 ) ) ;
#3788=CARTESIAN_POINT ( 'NONE',  ( 33.43833233143621442, -3.434996429908883098, -5.407889144347614696 ) ) ;
#3793=ADVANCED_FACE ( 'NONE', ( #26947 ), #16442, .T. ) ;
#3796=CARTESIAN_POINT ( 'NONE',  ( 30.44988808354906595, -2.941501225529987718, 4.958839487400774182 ) ) ;
#3802=B_SPLINE_CURVE_WITH_KNOTS ( 'NONE', 3,
 ( #16565, #29345, #22575, #23168 ),
 .UNSPECIFIED., .F., .F.,
 ( 4, 4 ),
 ( 0.8210829304512126114, 0.9474561098508307300 ),
 .UNSPECIFIED. ) ;
#3805=CARTESIAN_POINT ( 'NONE',  ( 23.66522075457919172, 3.155031241165582312, 3.754767217157412684 ) ) ;
#3812=CARTESIAN_POINT ( 'NONE',  ( 22.87842292266282129, 4.333480938141546446, 3.064138866945673723 ) ) ;
#3818=EDGE_CURVE ( 'NONE', #12484, #5958, #32288, .T. ) ;
#3821=CARTESIAN_POINT ( 'NONE',  ( 21.73434502951461056, 0.2315104026643188539, 9.064982765253589037 ) ) ;
#3829=CARTESIAN_POINT ( 'NONE',  ( 24.03893326528611141, 2.664202206450044130, -5.290213626918107259 ) ) ;
#3831=CARTESIAN_POINT ( 'NONE',  ( -74.86601972701976138, -2.929674985788335739, 9.238933323493853322 ) ) ;
#3832=CARTESIAN_POINT ( 'NONE',  ( 24.74313279468194793, 0.5480144272095329727, -4.780879834594610855 ) ) ;
#3839=CARTESIAN_POINT ( 'NONE',  ( 29.54642850493534567, -3.606211835941682153, -4.678983485493422023 ) ) ;
#3840=CARTESIAN_POINT ( 'NONE',  ( 36.49326386636163733, -3.559160538920521866, -5.796799980422059129 ) ) ;
#3842=CARTESIAN_POINT ( 'NONE',  ( 16.61276722214797275, 9.469120112283594182, 2.799222124946485035 ) ) ;
#3849=CARTESIAN_POINT ( 'NONE',  ( 24.78824275346884676, 1.421632137423702424, -4.544576515312537701 ) ) ;
#3850=CARTESIAN_POINT ( 'NONE',  ( 33.59320765816826082, -0.3498627648884612418, -5.050355079047641915 ) ) ;
#3853=EDGE_CURVE ( 'NONE', #13150, #26564, #32591, .T. ) ;
#3857=CARTESIAN_POINT ( 'NONE',  ( 87.67674921920735187, -0.7466428619051976856, -5.210926517169286676 ) ) ;
#3860=CARTESIAN_POINT ( 'NONE',  ( -72.89123299691203783, 3.290588968460324448, -10.95732599500614945 ) ) ;
#3867=VERTEX_POINT ( 'NONE', #38047 ) ;
#3873=EDGE_LOOP ( 'NONE', ( #30242, #17507, #25147, #10970, #33925, #12535, #40320 ) ) ;
#3878=CARTESIAN_POINT ( 'NONE',  ( 21.85643539959774628, 7.825395393543534972, -11.66269361450695108 ) ) ;
#3879=CARTESIAN_POINT ( 'NONE',  ( 24.36623814963473222, 3.146137341929644560, -3.353173740419891580 ) ) ;
#3882=EDGE_CURVE ( 'NONE', #12496, #7875, #17142, .T. ) ;
#3885=CARTESIAN_POINT ( 'NONE',  ( -75.07486328459704339, -3.143736151799179979, -10.45530216219834330 ) ) ;
#3890=CARTESIAN_POINT ( 'NONE',  ( 85.38915795161820199, 1.318023545160245558, -5.584599991349963766 ) ) ;
#3893=CARTESIAN_POINT ( 'NONE',  ( 21.53507218971822468, 7.396261084522392615, 0.9507677088441091051 ) ) ;
#3894=CARTESIAN_POINT ( 'NONE',  ( 33.55284483517386462, -1.200833309292756779, 5.443130933784450676 ) ) ;
#3903=CARTESIAN_POINT ( 'NONE',  ( 36.44751297234375187, -2.353303903281885656, 5.894913904403375149 ) ) ;
#3906=VECTOR ( 'NONE', #10189, 1000.000000000000000 ) ;
#3908=CARTESIAN_POINT ( 'NONE',  ( 88.52897200822518187, -1.082218601420786186, 0.1993289098281435523 ) ) ;
#3913=ORIENTED_EDGE ( 'NONE', *, *, #7068, .F. ) ;
#3914=FACE_OUTER_BOUND ( 'NONE', #16342, .T. ) ;
#3921=CARTESIAN_POINT ( 'NONE',  ( 24.50089963235556567, 1.790356837895823006, 4.437133755813296609 ) ) ;
#3926=CARTESIAN_POINT ( 'NONE',  ( 85.23804977158383167, 2.614301451366713991, 1.665401937347900763 ) ) ;
#3927=DIRECTION ( 'NONE',  ( -0.000000000000000000, 1.000000000000000000, -0.000000000000000000 ) ) ;
#3929=CARTESIAN_POINT ( 'NONE',  ( 23.64958599753803981, 3.252002366305553060, -3.672120356605920399 ) ) ;
#3933=CARTESIAN_POINT ( 'NONE',  ( 21.85643539959775694, 2.022457263371903569, 13.81434276849105558 ) ) ;
#3934=CARTESIAN_POINT ( 'NONE',  ( 21.77466435200733841, 5.668278662190309625, 2.100676170755116701 ) ) ;
#3938=CARTESIAN_POINT ( 'NONE',  ( 86.79297523138272652, 0.7501027249346864378, -5.742269118526623473 ) ) ;
#3939=ORIENTED_EDGE ( 'NONE', *, *, #766, .F. ) ;
#3940=CARTESIAN_POINT ( 'NONE',  ( 14.64292194440910500, -5.617547757890807958, 2.491780128467261601 ) ) ;
#3942=CARTESIAN_POINT ( 'NONE',  ( 37.04602089111122609, -2.800936193217299586, -5.988325540095575938 ) ) ;
#3951=CARTESIAN_POINT ( 'NONE',  ( 28.84716823796745189, -3.982103006514774002, 4.149921582050339453 ) ) ;
#3953=ORIENTED_EDGE ( 'NONE', *, *, #14972, .T. ) ;
#3954=CARTESIAN_POINT ( 'NONE',  ( 37.10426046727946670, -3.126190214317604799, 5.976248370712866631 ) ) ;
#3956=CARTESIAN_POINT ( 'NONE',  ( 87.50351120902806201, -1.998158110427775247, 3.528025977964829085 ) ) ;
#3965=CARTESIAN_POINT ( 'NONE',  ( 22.22653128512649090, 5.106210340169274886, 3.172958745359750310 ) ) ;
#3975=CARTESIAN_POINT ( 'NONE',  ( 4.588767459758324848E-15, -39.37473357531881391, 6.000000000000000000 ) ) ;
#3976=DIRECTION ( 'NONE',  ( -0.000000000000000000, -0.000000000000000000, -1.000000000000000000 ) ) ;
#3978=CARTESIAN_POINT ( 'NONE',  ( 86.31823139319517679, 1.400990185460310844, -4.784756222713710372 ) ) ;
#3979=CARTESIAN_POINT ( 'NONE',  ( 27.52542935251784328, 0.09321990139520379415, -5.913109915068038624 ) ) ;
#3981=CARTESIAN_POINT ( 'NONE',  ( -69.92837670882109080, -20.91525569503158977, 9.949874371066208312 ) ) ;
#3982=AXIS2_PLACEMENT_3D ( 'NONE', #28937, #9787, #6910 ) ;
#3987=CARTESIAN_POINT ( 'NONE',  ( 25.58354041903514187, 2.439056306859946233, -4.005116038328519146 ) ) ;
#3994=DIRECTION ( 'NONE',  ( -0.2817767355331954882, 0.9594800004753907263, 0.000000000000000000 ) ) ;
#3998=CARTESIAN_POINT ( 'NONE',  ( 33.46455515056310759, -3.089188617792877789, 5.429351193206847448 ) ) ;
#4003=ORIENTED_EDGE ( 'NONE', *, *, #28033, .T. ) ;
#4005=CARTESIAN_POINT ( 'NONE',  ( 30.48050265367797707, -3.144661348558943192, 4.957493858021535971 ) ) ;
#4006=CARTESIAN_POINT ( 'NONE',  ( 22.01915847652775327, 4.164052895855497205, 4.067381656372952570 ) ) ;
#4016=ORIENTED_EDGE ( 'NONE', *, *, #9483, .T. ) ;
#4018=CARTESIAN_POINT ( 'NONE',  ( 22.62923931292150570, 0.3004384395878155201, 6.475933053414085983 ) ) ;
#4026=CARTESIAN_POINT ( 'NONE',  ( 22.31758782591801094, 6.227955964823622459, -0.6941013191108784675 ) ) ;
#4029=CARTESIAN_POINT ( 'NONE',  ( -78.33073954512362036, -5.228239016004201822, 8.428737381316327770 ) ) ;
#4030=CARTESIAN_POINT ( 'NONE',  ( 26.06851587782132285, 0.7123551559736346350, -4.422872410777025642 ) ) ;
#4033=ORIENTED_EDGE ( 'NONE', *, *, #36814, .F. ) ;
#4034=CARTESIAN_POINT ( 'NONE',  ( 22.18112716655140204, 5.504259556802007403, 2.539316679596942183 ) ) ;
#4036=CARTESIAN_POINT ( 'NONE',  ( 21.73971061288548157, 4.236109109462486977, -2.798397955401881632 ) ) ;
#4039=CARTESIAN_POINT ( 'NONE',  ( 18.30092389467140634, 7.735072622103469797, 3.062699801917176945 ) ) ;
#4045=CARTESIAN_POINT ( 'NONE',  ( 35.47974504919754679, -1.182722008973795091, -5.478873071446319187 ) ) ;
#4051=CARTESIAN_POINT ( 'NONE',  ( 88.13894822871212398, -2.422255244508634053, -0.8714879239747004291 ) ) ;
#4054=CARTESIAN_POINT ( 'NONE',  ( -81.73845805635816930, 10.46959273479546049, -1.466899665262664021 ) ) ;
#4066=DIRECTION ( 'NONE',  ( 1.000000000000000000, 7.826543628040252284E-17, -0.000000000000000000 ) ) ;
#4071=CARTESIAN_POINT ( 'NONE',  ( 21.85643539959774273, -9.053501261307662418, 13.64238141129353110 ) ) ;
#4072=CARTESIAN_POINT ( 'NONE',  ( 23.73916140895965299, 3.555150681598093776, -3.202806708119017021 ) ) ;
#4073=ORIENTED_EDGE ( 'NONE', *, *, #4447, .F. ) ;
#4079=CARTESIAN_POINT ( 'NONE',  ( -73.04755721403003577, -2.452746795641160382, -9.775035012883797947 ) ) ;
#4083=CARTESIAN_POINT ( 'NONE',  ( 86.89103086197154369, -0.8412156502217053022, -5.497997349500185926 ) ) ;
#4093=CARTESIAN_POINT ( 'NONE',  ( 36.79828219115022137, -2.555128534534287787, 5.949659924383641219 ) ) ;
#4095=CARTESIAN_POINT ( 'NONE',  ( 85.45255010372768822, 2.373364497502822967, 3.195069691434311743 ) ) ;
#4099=DIRECTION ( 'NONE',  ( 0.000000000000000000, -0.000000000000000000, -1.000000000000000000 ) ) ;
#4103=ORIENTED_EDGE ( 'NONE', *, *, #34680, .T. ) ;
#4104=CARTESIAN_POINT ( 'NONE',  ( -72.92401200329621247, 7.089954214640987296, 9.800610954731245883 ) ) ;
#4105=VERTEX_POINT ( 'NONE', #33708 ) ;
#4108=CARTESIAN_POINT ( 'NONE',  ( 22.53938003481075825, 1.184789744452465321, 6.008811300886961249 ) ) ;
#4112=EDGE_CURVE ( 'NONE', #1778, #29684, #30098, .T. ) ;
#4114=ADVANCED_FACE ( 'NONE', ( #12678 ), #23820, .F. ) ;
#4117=CARTESIAN_POINT ( 'NONE',  ( 85.76128207622278410, 2.026582092692974069, 3.826057417255781967 ) ) ;
#4120=ORIENTED_EDGE ( 'NONE', *, *, #7991, .T. ) ;
#4121=CARTESIAN_POINT ( 'NONE',  ( 23.23159003004921885, 3.295630425265384300, -3.830492098241911503 ) ) ;
#4123=EDGE_CURVE ( 'NONE', #15644, #39711, #6523, .T. ) ;
#4125=CARTESIAN_POINT ( 'NONE',  ( 21.85643539959778536, -7.083161344002194326, -10.43125315386002860 ) ) ;
#4126=CARTESIAN_POINT ( 'NONE',  ( 20.16883043528743968, 11.76570021211175643, 3.257865388789312089 ) ) ;
#4131=CARTESIAN_POINT ( 'NONE',  ( 19.69441324270408700, -2.725662423435629922, 3.280187516344912346 ) ) ;
#4133=CARTESIAN_POINT ( 'NONE',  ( 16.00969967615263556, -3.370281526357195467, -2.705098849150198603 ) ) ;
#4134=CARTESIAN_POINT ( 'NONE',  ( 32.78094590778558626, -0.9280580154095039447, -5.322657437719364282 ) ) ;
#4136=CARTESIAN_POINT ( 'NONE',  ( -62.92837670882107659, -49.49506129533733656, -6.000000000000000000 ) ) ;
#4142=CARTESIAN_POINT ( 'NONE',  ( 28.23003454072220819, -3.405378548512706161, 4.612377654681626638 ) ) ;
#4145=CARTESIAN_POINT ( 'NONE',  ( 36.20113637138914697, -3.651277154294600091, 5.717575700238314518 ) ) ;
#4147=CARTESIAN_POINT ( 'NONE',  ( 87.45676830308305227, -1.940095815629343967, 3.699365911462623391 ) ) ;
#4153=CARTESIAN_POINT ( 'NONE',  ( -4.444218661349752963, -35.94265729135299381, 6.000000000000000000 ) ) ;
#4154=ORIENTED_EDGE ( 'NONE', *, *, #39587, .F. ) ;
#4174=CARTESIAN_POINT ( 'NONE',  ( 26.56638717734885802, 2.990222579127657099, 1.122734419917069237 ) ) ;
#4181=CARTESIAN_POINT ( 'NONE',  ( 36.68200451011485086, -3.313387469113171946, -5.912010938468631238 ) ) ;
#4183=LINE ( 'NONE', #7050, #18704 ) ;
#4186=CARTESIAN_POINT ( 'NONE',  ( -4.890026461918812295, -8.951974136083761024, 6.000000000000000000 ) ) ;
#4189=CARTESIAN_POINT ( 'NONE',  ( 32.91478736177253239, -0.5485403146597650492, 5.320368748126441005 ) ) ;
#4193=ORIENTED_EDGE ( 'NONE', *, *, #35353, .T. ) ;
#4196=CARTESIAN_POINT ( 'NONE',  ( 23.89044766034434275, 3.056531940009395765, 3.748979796177386081 ) ) ;
#4202=CARTESIAN_POINT ( 'NONE',  ( 14.75430999618867745, -4.622527584820372404, 2.500000000000000888 ) ) ;
#4206=EDGE_LOOP ( 'NONE', ( #22146, #8567, #25360, #23422, #15252 ) ) ;
#4208=CARTESIAN_POINT ( 'NONE',  ( 26.70483259202675086, 0.9606887959971135427, 4.381135443176162880 ) ) ;
#4218=CARTESIAN_POINT ( 'NONE',  ( 24.55145103709714505, -1.086933616027371263, 6.883468691731016165 ) ) ;
#4221=CARTESIAN_POINT ( 'NONE',  ( -76.32424250352048034, -4.240740262105982872, 8.445734442623528793 ) ) ;
#4222=LINE ( 'NONE', #1144, #18011 ) ;
#4225=CARTESIAN_POINT ( 'NONE',  ( 20.91978843656600517, 4.581251045227689112, -2.652517874115063012 ) ) ;
#4238=CIRCLE ( 'NONE', #26562, 12.73502530973474300 ) ;
#4240=CARTESIAN_POINT ( 'NONE',  ( 84.10013685850573495, 3.017793503712738357, 0.3246723698904760980 ) ) ;
#4244=CARTESIAN_POINT ( 'NONE',  ( 26.60765709881297880, 1.631430624340022506, 4.332177513178613104 ) ) ;
#4250=ADVANCED_FACE ( 'NONE', ( #5837 ), #36314, .T. ) ;
#4251=VERTEX_POINT ( 'NONE', #20651 ) ;
#4261=CARTESIAN_POINT ( 'NONE',  ( 33.54884098819741212, -4.040961204078771019, -4.876534918468718338 ) ) ;
#4263=CARTESIAN_POINT ( 'NONE',  ( 21.98979295893775543, 5.607672701399281756, -3.095502674479804206 ) ) ;
#4269=CARTESIAN_POINT ( 'NONE',  ( -75.59970171100725622, -3.666675714033016842, -8.878492054693071012 ) ) ;
#4277=CARTESIAN_POINT ( 'NONE',  ( 33.93654037581948302, -1.338830054478469478, 5.503015902613915600 ) ) ;
#4279=CARTESIAN_POINT ( 'NONE',  ( 15.84347261764352766, 10.40642223222415907, -2.679155096453247786 ) ) ;
#4284=CARTESIAN_POINT ( 'NONE',  ( 29.10196052430525171, 0.3604245502769343190, 4.748462792029568114 ) ) ;
#4288=CARTESIAN_POINT ( 'NONE',  ( 86.29974207331044056, 1.340767688666749446, -5.501321414410665689 ) ) ;
#4297=FACE_OUTER_BOUND ( 'NONE', #36494, .T. ) ;
#4307=CARTESIAN_POINT ( 'NONE',  ( 25.21589077596340189, 0.9012383917972676128, 4.613794564236588513 ) ) ;
#4316=CARTESIAN_POINT ( 'NONE',  ( 22.11632824126515828, 4.958352940722863700, -3.426487884367986236 ) ) ;
#4317=EDGE_LOOP ( 'NONE', ( #4193, #15572, #8359, #39908, #36854 ) ) ;
#4318=CYLINDRICAL_SURFACE ( 'NONE', #39498, 7.744449365083023729 ) ;
#4321=CARTESIAN_POINT ( 'NONE',  ( 21.85643539959778892, -9.157157878381195104, -8.039778668638760450 ) ) ;
#4323=CARTESIAN_POINT ( 'NONE',  ( 21.86904452675153365, 4.504091705278521651, 2.554698571754111767E-12 ) ) ;
#4326=CARTESIAN_POINT ( 'NONE',  ( 86.85482141032015591, 0.6757441427909987031, 5.750446197363288547 ) ) ;
#4327=CARTESIAN_POINT ( 'NONE',  ( -17.27251170661583402, 3.729367930467589076, -2.500000000000000444 ) ) ;
#4328=ORIENTED_EDGE ( 'NONE', *, *, #26787, .F. ) ;
#4330=CARTESIAN_POINT ( 'NONE',  ( -78.72866883428119422, -5.350567248293963019, 8.033035618889639906 ) ) ;
#4332=CARTESIAN_POINT ( 'NONE',  ( 14.76950060579820345, -5.972576308483009910, 2.511535789893701409 ) ) ;
#4334=CARTESIAN_POINT ( 'NONE',  ( 33.12369938294775551, -3.163197387429788510, -5.376152407042375181 ) ) ;
#4335=CARTESIAN_POINT ( 'NONE',  ( 30.51439263097747556, -0.1427504069471233206, -4.968906982075368184 ) ) ;
#4337=CARTESIAN_POINT ( 'NONE',  ( 84.10579224183346980, 3.010952253929020550, -0.2616020758091565646 ) ) ;
#4341=VERTEX_POINT ( 'NONE', #25585 ) ;
#4342=VERTEX_POINT ( 'NONE', #22312 ) ;
#4343=CARTESIAN_POINT ( 'NONE',  ( 35.83251579909378393, -3.729987874846103058, 5.623171243541962738 ) ) ;
#4344=CARTESIAN_POINT ( 'NONE',  ( 14.77222811005485603, -4.461988841550141416, 2.511961482897715481 ) ) ;
#4348=CARTESIAN_POINT ( 'NONE',  ( 87.92068663493991210, -2.504771375202706540, 0.3618066692888307623 ) ) ;
#4349=EDGE_CURVE ( 'NONE', #9974, #30067, #24388, .T. ) ;
#4357=CARTESIAN_POINT ( 'NONE',  ( 22.08043625007045563, 5.168148467668603807, 3.316046242248380960 ) ) ;
#4368=CARTESIAN_POINT ( 'NONE',  ( 23.59090747053171100, 2.763374893270500010, -4.088477763750560712 ) ) ;
#4371=CARTESIAN_POINT ( 'NONE',  ( -2.697268050091675118E-17, 3.729367930467589076, 2.500000000000000000 ) ) ;
#4375=CARTESIAN_POINT ( 'NONE',  ( 27.87477497239535396, 2.606304449749688779, 1.085873857364543671 ) ) ;
#4377=CARTESIAN_POINT ( 'NONE',  ( 21.85643539959777115, -15.24623503193425123, 0.9260495571226281530 ) ) ;
#4378=CARTESIAN_POINT ( 'NONE',  ( -78.24659595803589696, -5.198025430032019223, -8.506940804273437351 ) ) ;
#4383=CARTESIAN_POINT ( 'NONE',  ( 37.12953470293586378, -2.935607199016813329, -5.998835710568205748 ) ) ;
#4389=EDGE_CURVE ( 'NONE', #11923, #23464, #34943, .T. ) ;
#4394=CARTESIAN_POINT ( 'NONE',  ( 23.23260104507673418, 3.379988935392680638, 3.619754408035347204 ) ) ;
#4402=CARTESIAN_POINT ( 'NONE',  ( 85.56005740296494366, 1.042223677629517287, -5.769124288340541362 ) ) ;
#4407=CARTESIAN_POINT ( 'NONE',  ( 23.14042469615008812, 4.038978393511998277, 3.095302447830163839 ) ) ;
#4413=CARTESIAN_POINT ( 'NONE',  ( 25.39883144959904726, 0.6937492590089258115, 4.599813248329277293 ) ) ;
#4422=FACE_OUTER_BOUND ( 'NONE', #1071, .T. ) ;
#4423=CARTESIAN_POINT ( 'NONE',  ( 26.56634348862415251, 2.991955253353971500, -0.5426703667890996341 ) ) ;
#4426=CARTESIAN_POINT ( 'NONE',  ( -73.66256240681488521, -1.125518199222426130, 9.676865719492857565 ) ) ;
#4427=CARTESIAN_POINT ( 'NONE',  ( 25.40152483165711672, 0.6871398706826929992, -4.599596795371007296 ) ) ;
#4428=DIRECTION ( 'NONE',  ( -0.000000000000000000, -0.000000000000000000, -1.000000000000000000 ) ) ;
#4429=CARTESIAN_POINT ( 'NONE',  ( 21.58862418887968460, 7.202556094215188054, 2.923978954502209682 ) ) ;
#4431=CARTESIAN_POINT ( 'NONE',  ( 33.68489815951246413, -3.839215430596429002, -5.138831521973123984 ) ) ;
#4432=CARTESIAN_POINT ( 'NONE',  ( 30.63322649116577523, -3.239464216780934436, -4.965866477755658259 ) ) ;
#4438=CIRCLE ( 'NONE', #3774, 12.73502530973474300 ) ;
#4440=CARTESIAN_POINT ( 'NONE',  ( 22.53894523562045293, 1.168954165206360862, -6.023172632562342699 ) ) ;
#4447=EDGE_CURVE ( 'NONE', #6564, #40623, #30994, .T. ) ;
#4448=EDGE_CURVE ( 'NONE', #18960, #24982, #40606, .T. ) ;
#4449=CARTESIAN_POINT ( 'NONE',  ( 85.74309555164268204, 1.026708856660649705, -5.825338620068188256 ) ) ;
#4451=CARTESIAN_POINT ( 'NONE',  ( -74.69100398025469190, 7.583772050443990942, -10.58965610702078841 ) ) ;
#4461=CARTESIAN_POINT ( 'NONE',  ( 36.21386368451217663, -1.588474078234619169, 5.668731034284322234 ) ) ;
#4463=CYLINDRICAL_SURFACE ( 'NONE', #36166, 12.38600677260393113 ) ;
#4464=ORIENTED_EDGE ( 'NONE', *, *, #21922, .F. ) ;
#4465=CARTESIAN_POINT ( 'NONE',  ( 27.43879754216082389, 0.9604377377020558715, 4.488885984917203587 ) ) ;
#4469=CARTESIAN_POINT ( 'NONE',  ( 33.79079129742034127, -4.868640718861981576, -3.414904310288808365 ) ) ;
#4471=AXIS2_PLACEMENT_3D ( 'NONE', #14092, #26274, #10602 ) ;
#4472=LINE ( 'NONE', #25479, #11600 ) ;
#4473=CARTESIAN_POINT ( 'NONE',  ( -72.95661835997130140, 1.053701266592789398, -9.852289288704627168 ) ) ;
#4475=LINE ( 'NONE', #19508, #26068 ) ;
#4488=CARTESIAN_POINT ( 'NONE',  ( 36.19474364399976452, -2.230523885484240854, 5.855463137465835466 ) ) ;
#4491=CARTESIAN_POINT ( 'NONE',  ( 88.39837738899358044, -0.9355285267052176890, 2.786041992172542336 ) ) ;
#4498=CARTESIAN_POINT ( 'NONE',  ( -78.35024558020644747, 11.32744874732892804, -6.714849854229168358 ) ) ;
#4499=CARTESIAN_POINT ( 'NONE',  ( 21.73879351235361668, 6.093659825503084271, 3.276088519256564524 ) ) ;
#4506=CARTESIAN_POINT ( 'NONE',  ( 24.90057636419620124, 1.281227854881117789, 4.570978506677809250 ) ) ;
#4511=CARTESIAN_POINT ( 'NONE',  ( 18.51265066377991531, 11.53724448280501313, 2.500000000000000000 ) ) ;
#4512=CARTESIAN_POINT ( 'NONE',  ( -70.92837670882107659, -23.80776546975053165, -10.00000000000000888 ) ) ;
#4515=CARTESIAN_POINT ( 'NONE',  ( 23.97627728469320019, 3.287926408277590085, -3.421875469786679336 ) ) ;
#4518=CARTESIAN_POINT ( 'NONE',  ( 22.46150523612397976, 0.3089437977474873143, 9.145744397224946809 ) ) ;
#4519=CARTESIAN_POINT ( 'NONE',  ( 17.12093179650374708, 14.48834468576525758, -3.790908043361014279 ) ) ;
#4524=CARTESIAN_POINT ( 'NONE',  ( 86.43196921298398649, 0.8512835087624049946, 5.909244108978848331 ) ) ;
#4526=ORIENTED_EDGE ( 'NONE', *, *, #12031, .F. ) ;
#4529=CARTESIAN_POINT ( 'NONE',  ( 22.43255271695741371, 5.122918363847896117, -2.447134636434162847 ) ) ;
#4530=CARTESIAN_POINT ( 'NONE',  ( 14.75024544199591503, -5.969387982752670574, -2.508530555894281200 ) ) ;
#4531=CARTESIAN_POINT ( 'NONE',  ( 36.99218678239946456, -2.719487527304628394, -5.979923425448357754 ) ) ;
#4534=CARTESIAN_POINT ( 'NONE',  ( 29.68218759030339271, -3.793136067405761924, -4.440320134392340634 ) ) ;
#4540=VERTEX_POINT ( 'NONE', #29675 ) ;
#4542=CARTESIAN_POINT ( 'NONE',  ( 35.22074791301828611, -1.047776788863644226, 5.411314349319545691 ) ) ;
#4550=CARTESIAN_POINT ( 'NONE',  ( 21.90912465241696694, 3.662607847362923774, -2.128491611114075699 ) ) ;
#4552=CARTESIAN_POINT ( 'NONE',  ( 23.96426883893546389, 3.278871655312407984, 3.444941816143999969 ) ) ;
#4561=ORIENTED_EDGE ( 'NONE', *, *, #39880, .T. ) ;
#4562=CARTESIAN_POINT ( 'NONE',  ( 23.43636678123177219, 2.538610166689087677, -4.312835133894656003 ) ) ;
#4564=CARTESIAN_POINT ( 'NONE',  ( 16.14043970921329674, 15.25505324876322888, -0.6630684997063907016 ) ) ;
#4565=DIRECTION ( 'NONE',  ( -0.000000000000000000, -0.000000000000000000, -1.000000000000000000 ) ) ;
#4569=CARTESIAN_POINT ( 'NONE',  ( 85.17359253740836778, 2.686702876117401662, 1.784494502703901864 ) ) ;
#4570=CARTESIAN_POINT ( 'NONE',  ( 33.61282307965942806, -4.196488527906213406, -4.700131347630155609 ) ) ;
#4574=CARTESIAN_POINT ( 'NONE',  ( -72.42837670882107659, -47.11702805680359063, 9.886859966642603581 ) ) ;
#4579=CARTESIAN_POINT ( 'NONE',  ( 35.33513638873442630, -3.237442486773212558, -5.721300635602096563 ) ) ;
#4586=CARTESIAN_POINT ( 'NONE',  ( 36.29298905792148133, -2.016294748008292892, 5.862889200204672413 ) ) ;
#4593=CARTESIAN_POINT ( 'NONE',  ( 85.65758405518126040, 0.8774719100965696628, -5.855775047906961461 ) ) ;
#4595=PLANE ( 'NONE',  #39140 ) ;
#4598=CARTESIAN_POINT ( 'NONE',  ( 24.40258831255338734, 3.162078629162225152, 3.277950946408194621 ) ) ;
#4599=CARTESIAN_POINT ( 'NONE',  ( 0.6783104270758654186, -48.60743831809499227, -2.500000000000000000 ) ) ;
#4600=EDGE_CURVE ( 'NONE', #19379, #38217, #10595, .T. ) ;
#4605=CARTESIAN_POINT ( 'NONE',  ( 21.73501309383516045, 0.2561466533226999243, 9.001404038369074101 ) ) ;
#4606=CARTESIAN_POINT ( 'NONE',  ( 14.69558838330761930, -4.461995682952461628, -2.500000000000009770 ) ) ;
#4614=CARTESIAN_POINT ( 'NONE',  ( 59.69572451838116933, -0.8894979772356270686, 5.999999999999999112 ) ) ;
#4615=CARTESIAN_POINT ( 'NONE',  ( 30.13572739226143327, -4.670734905539763560, 0.4584422186006349986 ) ) ;
#4618=CARTESIAN_POINT ( 'NONE',  ( -74.01468305983279095, -3.815910838439570352, 9.516541306992865046 ) ) ;
#4619=CARTESIAN_POINT ( 'NONE',  ( 21.98018615774344653, 0.2297809094950876430, -7.706785321375619446 ) ) ;
#4621=LINE ( 'NONE', #17344, #27432 ) ;
#4626=CARTESIAN_POINT ( 'NONE',  ( 21.73769930489046232, 4.234352968378803261, -2.806692186376322340 ) ) ;
#4627=LINE ( 'NONE', #39183, #2992 ) ;
#4630=CARTESIAN_POINT ( 'NONE',  ( -72.12732577070732987, -48.03925814481806356, 5.880655408758564739 ) ) ;
#4638=CARTESIAN_POINT ( 'NONE',  ( 87.11462257552980759, -1.147413441766115039, -5.140310012396687611 ) ) ;
#4645=ADVANCED_FACE ( 'NONE', ( #8234 ), #38801, .T. ) ;
#4649=CARTESIAN_POINT ( 'NONE',  ( 12.97258467943525062, 9.268118853444669014, -3.480631448259292604 ) ) ;
#4655=CARTESIAN_POINT ( 'NONE',  ( 21.85643539959776049, -12.91308397612913161, -3.835380774090566103 ) ) ;
#4659=CARTESIAN_POINT ( 'NONE',  ( 14.72840846699002526, -4.935183498936103419, 2.501324498462070167 ) ) ;
#4661=CARTESIAN_POINT ( 'NONE',  ( -74.32433723247588375, -2.242446129776642927, -10.69717072308378469 ) ) ;
#4676=CARTESIAN_POINT ( 'NONE',  ( 33.62922731160094969, -1.227221384262835890, 5.455052266548129580 ) ) ;
#4679=CARTESIAN_POINT ( 'NONE',  ( 86.01579553793663990, 1.740700492558412193, -4.743980989581940477 ) ) ;
#4684=VERTEX_POINT ( 'NONE', #836 ) ;
#4695=CARTESIAN_POINT ( 'NONE',  ( 26.03758185223221489, 1.465628984450591643, 4.326634389998879726 ) ) ;
#4703=CARTESIAN_POINT ( 'NONE',  ( 22.95716255745577428, 3.903089801653534696, -3.484934174897956094 ) ) ;
#4704=ORIENTED_EDGE ( 'NONE', *, *, #20307, .T. ) ;
#4708=CARTESIAN_POINT ( 'NONE',  ( 23.92272977471906614, 4.146422156947720872, -1.204255912843045229 ) ) ;
#4713=CARTESIAN_POINT ( 'NONE',  ( 85.61248512101352048, 1.464218027013357570, -5.526712519226341769 ) ) ;
#4718=CARTESIAN_POINT ( 'NONE',  ( 33.12062221538703000, -3.232445517116538714, -5.375672140621767348 ) ) ;
#4719=CARTESIAN_POINT ( 'NONE',  ( 29.09977985558236924, 0.3540121042850735145, -4.748122445935673674 ) ) ;
#4720=DIRECTION ( 'NONE',  ( 0.9880385148181951571, 0.000000000000000000, -0.1542073060391599970 ) ) ;
#4721=CARTESIAN_POINT ( 'NONE',  ( 84.57639812724936235, 2.428913470196615521, -3.745062422066182339 ) ) ;
#4722=CARTESIAN_POINT ( 'NONE',  ( 30.45118816949839768, -3.644433509500874635, -4.694111347297837078 ) ) ;
#4730=CARTESIAN_POINT ( 'NONE',  ( 33.68516129456243391, -3.840378280999563465, 5.137618048204199539 ) ) ;
#4732=EDGE_CURVE ( 'NONE', #39711, #34290, #29151, .T. ) ;
#4734=CARTESIAN_POINT ( 'NONE',  ( 87.82094399217496061, -2.385319725885814535, 1.832678672200965364 ) ) ;
#4735=ORIENTED_EDGE ( 'NONE', *, *, #20307, .F. ) ;
#4736=EDGE_LOOP ( 'NONE', ( #13583, #10954, #32616, #28436 ) ) ;
#4742=CARTESIAN_POINT ( 'NONE',  ( 22.27435398669647881, 4.892900451708169562, 3.295348648465727948 ) ) ;
#4751=CARTESIAN_POINT ( 'NONE',  ( 22.47393122894036210, 2.796275671460458412, -4.701534300632203234 ) ) ;
#4759=CARTESIAN_POINT ( 'NONE',  ( 87.55151927672237377, 0.01570269930849589254, 4.249584817138070569 ) ) ;
#4760=CARTESIAN_POINT ( 'NONE',  ( 29.34248944929254677, 1.775380825033272991, -3.063368523016994249 ) ) ;
#4765=CARTESIAN_POINT ( 'NONE',  ( 23.84965713394175424, -3.142048526390663010, 3.808973460114609466 ) ) ;
#4767=CARTESIAN_POINT ( 'NONE',  ( 33.67567688289796024, -3.265297112828876802, -5.462301845497175457 ) ) ;
#4770=DIRECTION ( 'NONE',  ( 0.000000000000000000, 0.000000000000000000, 1.000000000000000000 ) ) ;
#4773=EDGE_LOOP ( 'NONE', ( #10996, #15436, #30781, #20986 ) ) ;
#4774=CARTESIAN_POINT ( 'NONE',  ( 33.82075086788260876, -0.7236657158041540638, 5.383591898491746797 ) ) ;
#4792=CARTESIAN_POINT ( 'NONE',  ( 23.14123425308138593, 4.046733741470082357, 3.080193756421565787 ) ) ;
#4799=CARTESIAN_POINT ( 'NONE',  ( 21.77915618962539313, 0.2033484107530734719, 8.424735242863125251 ) ) ;
#4800=CARTESIAN_POINT ( 'NONE',  ( 14.75683830447593614, -5.152850317976760408, -2.499999999999999556 ) ) ;
#4803=ORIENTED_EDGE ( 'NONE', *, *, #36733, .F. ) ;
#4810=CARTESIAN_POINT ( 'NONE',  ( 28.22557690513166762, 1.384627073958520249, -4.541740331631825001 ) ) ;
#4814=CARTESIAN_POINT ( 'NONE',  ( -81.82461451913749784, -5.600584684740513630, -0.2075332267605694003 ) ) ;
#4815=CARTESIAN_POINT ( 'NONE',  ( 23.06578088975079410, 0.3556780097724844825, -5.946217273123633795 ) ) ;
#4818=CARTESIAN_POINT ( 'NONE',  ( 37.10903179270489716, -2.404814453197160695, -5.951927498713348363 ) ) ;
#4826=EDGE_CURVE ( 'NONE', #32259, #30233, #5513, .T. ) ;
#4833=CARTESIAN_POINT ( 'NONE',  ( 87.02687067233559048, -1.029203037998749570, 5.291918051785640564 ) ) ;
#4840=CARTESIAN_POINT ( 'NONE',  ( 24.78141585081923992, 3.030236314331866687, 3.301436159119843339 ) ) ;
#4844=CARTESIAN_POINT ( 'NONE',  ( 33.87044765521353185, -5.290189018693288503, 1.967003440103135548 ) ) ;
#4848=CARTESIAN_POINT ( 'NONE',  ( 15.06093162081344694, 12.12817333299150135, -2.535899686230826067 ) ) ;
#4849=DIRECTION ( 'NONE',  ( 1.000000000000000000, 0.000000000000000000, 0.000000000000000000 ) ) ;
#4850=CARTESIAN_POINT ( 'NONE',  ( 21.85643539959776760, 8.340603020592608274, -8.602649199348869402 ) ) ;
#4852=CARTESIAN_POINT ( 'NONE',  ( -77.10977740483862419, 9.586436412528746231, 7.873194102962211005 ) ) ;
#4853=CARTESIAN_POINT ( 'NONE',  ( 14.73544869152550696, -5.109937501475094734, 2.500000000000000444 ) ) ;
#4856=CARTESIAN_POINT ( 'NONE',  ( -75.61667019430753101, 8.531147133863177245, -10.24029099541588650 ) ) ;
#4857=CARTESIAN_POINT ( 'NONE',  ( 37.21266877546892005, -2.743693451709001252, -6.000906079407704929 ) ) ;
#4866=VECTOR ( 'NONE', #2283, 1000.000000000000000 ) ;
#4868=CARTESIAN_POINT ( 'NONE',  ( 36.79866761904986561, -2.554542194025152035, 5.949720079728989752 ) ) ;
#4871=CARTESIAN_POINT ( 'NONE',  ( 85.42332570945818304, 2.406190724219733568, -3.391956346677281076 ) ) ;
#4874=CARTESIAN_POINT ( 'NONE',  ( 29.58360395842353796, 0.1927886596133820130, -4.823634898514195690 ) ) ;
#4878=CARTESIAN_POINT ( 'NONE',  ( -69.92837670882107659, -20.78299143688747819, 5.916079783099617906 ) ) ;
#4880=ORIENTED_EDGE ( 'NONE', *, *, #35633, .F. ) ;
#4884=ORIENTED_EDGE ( 'NONE', *, *, #25933, .F. ) ;
#4888=CARTESIAN_POINT ( 'NONE',  ( 24.43811349724861515, 1.135655287698857929, 4.744166224008156796 ) ) ;
#4897=CARTESIAN_POINT ( 'NONE',  ( 22.71523255480387604, 4.231905031421672625, -3.372270972680762036 ) ) ;
#4901=CARTESIAN_POINT ( 'NONE',  ( 22.53076953550388950, -1.409035359855524749, -9.122014670555362414 ) ) ;
#4905=CARTESIAN_POINT ( 'NONE',  ( 84.58609069645564205, 2.764543530557054041, -2.886136738505205912 ) ) ;
#4909=CARTESIAN_POINT ( 'NONE',  ( -79.55031281509177177, -5.535808051698485777, 7.055139847234975115 ) ) ;
#4912=CARTESIAN_POINT ( 'NONE',  ( 25.01091298175105848, 3.329590532566609529, -1.936828115965013142 ) ) ;
#4913=CARTESIAN_POINT ( 'NONE',  ( 23.83302048315688992, -3.061032822375338025, -3.850069817691858187 ) ) ;
#4914=CARTESIAN_POINT ( 'NONE',  ( 35.45326567125915318, -1.915512047056902256, -5.739737567107160210 ) ) ;
#4917=CARTESIAN_POINT ( 'NONE',  ( 21.73976651585488895, 0.3939909484403775197, -8.664878499868692074 ) ) ;
#4919=ORIENTED_EDGE ( 'NONE', *, *, #30978, .T. ) ;
#4920=CARTESIAN_POINT ( 'NONE',  ( 37.04303371899823816, -2.892454996259951727, 5.987859319642387490 ) ) ;
#4922=CARTESIAN_POINT ( 'NONE',  ( 31.83096507438640188, -2.965444956201115811, -5.174389953294182831 ) ) ;
#4925=CARTESIAN_POINT ( 'NONE',  ( 20.91979337306159081, 4.581248967235889147, 2.652518752413522307 ) ) ;
#4927=LINE ( 'NONE', #10693, #37919 ) ;
#4929=ADVANCED_FACE ( 'NONE', ( #37029 ), #28050, .F. ) ;
#4943=ORIENTED_EDGE ( 'NONE', *, *, #18735, .F. ) ;
#4944=CARTESIAN_POINT ( 'NONE',  ( 21.98915976803599293, 4.682270550536856923, 3.756922458215664395 ) ) ;
#4946=VECTOR ( 'NONE', #29631, 1000.000000000000000 ) ;
#4947=CIRCLE ( 'NONE', #10868, 8.080217238368755162 ) ;
#4954=EDGE_LOOP ( 'NONE', ( #17719, #25856, #28013, #19643, #9029 ) ) ;
#4955=CARTESIAN_POINT ( 'NONE',  ( 22.04665046261544248, 2.511317956134706986, -5.313134278748806061 ) ) ;
#4963=CARTESIAN_POINT ( 'NONE',  ( 85.36681891225420316, 2.469661840813765608, 2.484336716295309166 ) ) ;
#4964=CARTESIAN_POINT ( 'NONE',  ( 27.93970670347097851, 2.313158937601060838, 2.612756796560576689 ) ) ;
#4969=CARTESIAN_POINT ( 'NONE',  ( 17.15960986616130057, -3.267607912849484375, 2.851956029205625409 ) ) ;
#4971=CARTESIAN_POINT ( 'NONE',  ( 36.14547465321244601, -3.195512951925109757, -5.847773519878426640 ) ) ;
#4979=ORIENTED_EDGE ( 'NONE', *, *, #30612, .T. ) ;
#4980=CARTESIAN_POINT ( 'NONE',  ( 36.02627438905632573, -1.730095084077468481, 5.776804761617037265 ) ) ;
#4983=AXIS2_PLACEMENT_3D ( 'NONE', #269, #6035, #31360 ) ;
#4985=ORIENTED_EDGE ( 'NONE', *, *, #40046, .F. ) ;
#4990=CARTESIAN_POINT ( 'NONE',  ( -78.09790289012752851, 11.26711229117069735, 6.983148571841773844 ) ) ;
#4994=CARTESIAN_POINT ( 'NONE',  ( 21.99104032157442390, 5.601135775457250610, 3.099302606858675535 ) ) ;
#4998=ORIENTED_EDGE ( 'NONE', *, *, #2009, .F. ) ;
#5000=B_SPLINE_CURVE_WITH_KNOTS ( 'NONE', 3,
 ( #18688, #25090, #24461, #6563, #37619, #5737, #31272, #37830, #9014, #19109, #9634, #40717, #22217, #9418, #24885 ),
 .UNSPECIFIED., .F., .F.,
 ( 4, 2, 2, 1, 1, 1, 1, 1, 2, 4 ),
 ( 0.4819642147472752991, 0.4909821073736378994, 0.4954910536868194493, 0.4977455268434102242, 0.4988727634217053897, 0.4994363817108530279, 0.4997181908554266805, 0.4998590954277135068, 0.4999295477138567256, 0.5000000000000000000 ),
 .UNSPECIFIED. ) ;
#5001=CARTESIAN_POINT ( 'NONE',  ( 26.06852323663950344, 0.7122034496989984032, 4.422876470770067847 ) ) ;
#5002=CARTESIAN_POINT ( 'NONE',  ( 14.74846712742400001, -5.105618172135831578, -2.500089296388391613 ) ) ;
#5009=CARTESIAN_POINT ( 'NONE',  ( 36.10284116201629701, 0.9159659085930716982, -6.000000000000000000 ) ) ;
#5010=CARTESIAN_POINT ( 'NONE',  ( 29.52748857962093965, -2.713093490715668743, -5.368793458836177201 ) ) ;
#5013=ORIENTED_EDGE ( 'NONE', *, *, #9148, .F. ) ;
#5015=CARTESIAN_POINT ( 'NONE',  ( 22.29087474900200050, 0.2567279992677524159, -7.116332770368763327 ) ) ;
#5021=CARTESIAN_POINT ( 'NONE',  ( 37.00929082827390459, -2.250120747072028138, -5.913434965054697123 ) ) ;
#5032=ORIENTED_EDGE ( 'NONE', *, *, #16086, .T. ) ;
#5036=CARTESIAN_POINT ( 'NONE',  ( 87.26468549332315661, -1.699173523771937644, 4.325011594718342067 ) ) ;
#5049=CARTESIAN_POINT ( 'NONE',  ( 16.68329415696692664, 9.858079400870805031, -2.499999999999912959 ) ) ;
#5056=CARTESIAN_POINT ( 'NONE',  ( 21.85643539959774273, -7.955861821551272861, 12.12136874776577322 ) ) ;
#5058=CARTESIAN_POINT ( 'NONE',  ( -80.77358443228958151, 10.51022734914309531, 4.964753886184787746 ) ) ;
#5059=CARTESIAN_POINT ( 'NONE',  ( 14.78321307761975234, -5.165297048227083465, 2.500001704151146420 ) ) ;
#5061=CARTESIAN_POINT ( 'NONE',  ( -77.38302135847544605, 11.04206681912608978, -7.647767078175882638 ) ) ;
#5070=EDGE_CURVE ( 'NONE', #18492, #141, #6684, .T. ) ;
#5072=AXIS2_PLACEMENT_3D ( 'NONE', #7054, #35681, #29089 ) ;
#5075=CARTESIAN_POINT ( 'NONE',  ( 87.90580911867260738, -0.3822524667802704168, 3.357330413655388757 ) ) ;
#5079=CARTESIAN_POINT ( 'NONE',  ( 36.21770968404204183, -2.179824564146979338, 5.859047543450206952 ) ) ;
#5081=CARTESIAN_POINT ( 'NONE',  ( 88.21591849536395102, -0.7305820373589052563, 3.481732356799086769 ) ) ;
#5082=CARTESIAN_POINT ( 'NONE',  ( 31.38399832331403161, -1.255798082282080008, 5.972680360385385079 ) ) ;
#5083=CARTESIAN_POINT ( 'NONE',  ( 31.23875116262452778, -0.3865744936300196111, -5.081960649616163117 ) ) ;
#5084=LINE ( 'NONE', #39446, #34046 ) ;
#5093=AXIS2_PLACEMENT_3D ( 'NONE', #27238, #4428, #16953 ) ;
#5095=CARTESIAN_POINT ( 'NONE',  ( 24.04774667349223094, 0.8530566696381411962, 5.040905544005979344 ) ) ;
#5099=EDGE_CURVE ( 'NONE', #8271, #20794, #7484, .T. ) ;
#5102=CARTESIAN_POINT ( 'NONE',  ( 14.69558838330753936, -3.003688195628454238, -6.000000000000000888 ) ) ;
#5106=CARTESIAN_POINT ( 'NONE',  ( 23.95987346625971171, 3.275624734069571442, -3.453389381892394638 ) ) ;
#5110=CARTESIAN_POINT ( 'NONE',  ( 21.85643539959775339, 5.487231995601864476, 10.01193108169250578 ) ) ;
#5114=CARTESIAN_POINT ( 'NONE',  ( 87.67674921920735187, -0.7466428619051976856, -5.210926517169286676 ) ) ;
#5122=CARTESIAN_POINT ( 'NONE',  ( 33.12654886128940035, -3.652994402058499013, -5.215079931666823043 ) ) ;
#5123=CARTESIAN_POINT ( 'NONE',  ( 22.91837443496737237, 2.645784632913941170, -3.783364632193285004 ) ) ;
#5124=FACE_OUTER_BOUND ( 'NONE', #26549, .T. ) ;
#5125=CARTESIAN_POINT ( 'NONE',  ( 26.78359742506201968, 1.531162930580288073, -4.367563350258214960 ) ) ;
#5128=CARTESIAN_POINT ( 'NONE',  ( 34.33118553565899589, -1.490639677210669145, 5.564609824335974508 ) ) ;
#5133=CARTESIAN_POINT ( 'NONE',  ( 35.22190015492834902, -1.045615856747100780, 5.409212822378231422 ) ) ;
#5135=CARTESIAN_POINT ( 'NONE',  ( 14.66504043345076447, 12.84305297963188863, -2.500000000000000000 ) ) ;
#5137=ORIENTED_EDGE ( 'NONE', *, *, #13992, .F. ) ;
#5143=AXIS2_PLACEMENT_3D ( 'NONE', #2556, #21270, #37108 ) ;
#5144=CARTESIAN_POINT ( 'NONE',  ( 14.72857438083221027, -4.937295716523431466, 2.501304222021813128 ) ) ;
#5146=DIRECTION ( 'NONE',  ( 1.000000000000000000, 0.000000000000000000, 0.000000000000000000 ) ) ;
#5148=CARTESIAN_POINT ( 'NONE',  ( 23.17090746384732824, 3.812297950970844784, 3.383282008515589911 ) ) ;
#5152=B_SPLINE_CURVE_WITH_KNOTS ( 'NONE', 3,
 ( #37722, #35090, #28888, #696, #31374, #22522, #13428, #12623, #35288, #6864, #15717, #497, #34890, #22114, #9939, #31781, #3596, #3201, #7056, #34479, #16121, #28269, #91 ),
 .UNSPECIFIED., .F., .F.,
 ( 4, 1, 1, 1, 1, 1, 1, 2, 2, 1, 1, 1, 1, 1, 2, 2, 4 ),
 ( 0.000000000000000000, 0.1249999999999883982, 0.1874999999999822364, 0.2187499999999795997, 0.2343749999999782674, 0.2421874999999781286, 0.2460937499999785449, 0.2480468749999787670, 0.2499999999999789613, 0.3749999999999901745, 0.4374999999999960032, 0.4687499999999989453, 0.4843750000000004996, 0.4921875000000016653, 0.4960937500000021649, 0.5000000000000026645, 1.000000000000000000 ),
 .UNSPECIFIED. ) ;
#5154=CARTESIAN_POINT ( 'NONE',  ( 30.19238557334687911, -2.952639005720375742, -4.918649992961978690 ) ) ;
#5158=CARTESIAN_POINT ( 'NONE',  ( 23.15855103537317206, 2.689427168583138350, -4.343935680606369587 ) ) ;
#5166=CARTESIAN_POINT ( 'NONE',  ( 87.09859342968812257, 0.5244505078549105415, -5.068689133590885909 ) ) ;
#5167=CARTESIAN_POINT ( 'NONE',  ( 30.13988473044573624, 0.1694294105150049301, -5.382122866902316893 ) ) ;
#5169=ADVANCED_FACE ( 'NONE', ( #31894 ), #26335, .T. ) ;
#5171=CARTESIAN_POINT ( 'NONE',  ( -78.80630328534653017, -5.372281114570830240, -7.948834340388816422 ) ) ;
#5173=CARTESIAN_POINT ( 'NONE',  ( 28.89721236653044301, -3.425550027173258627, 4.559861221518604957 ) ) ;
#5176=CARTESIAN_POINT ( 'NONE',  ( 34.36133827824247078, -1.406879114103402273, -5.569315889062961489 ) ) ;
#5183=CARTESIAN_POINT ( 'NONE',  ( 36.96501263788630354, -2.310926168294844985, 5.934243022296812775 ) ) ;
#5186=VECTOR ( 'NONE', #37937, 1000.000000000000114 ) ;
#5189=CARTESIAN_POINT ( 'NONE',  ( 0.000000000000000000, 0.000000000000000000, 2.500000000000000000 ) ) ;
#5192=CARTESIAN_POINT ( 'NONE',  ( -75.60183227957097074, 10.11098911773139442, 8.848339649221273362 ) ) ;
#5193=CARTESIAN_POINT ( 'NONE',  ( -70.92837670882107659, -23.80776546975053165, 0.000000000000000000 ) ) ;
#5196=CARTESIAN_POINT ( 'NONE',  ( 22.87897072576537738, 4.322970251960089882, 3.079858772812353429 ) ) ;
#5201=VERTEX_POINT ( 'NONE', #32962 ) ;
#5203=CARTESIAN_POINT ( 'NONE',  ( 22.29360747402898824, 0.2601931310903464190, 7.110083990419366451 ) ) ;
#5209=CARTESIAN_POINT ( 'NONE',  ( 35.37144363141613468, -3.783876837969972762, -5.514777695184551298 ) ) ;
#5211=CARTESIAN_POINT ( 'NONE',  ( 0.000000000000000000, 0.000000000000000000, -2.500000000000000000 ) ) ;
#5213=CARTESIAN_POINT ( 'NONE',  ( 30.13146195922598380, -4.635528103762326602, -0.9093114724505712010 ) ) ;
#5214=LINE ( 'NONE', #3185, #22783 ) ;
#5218=CARTESIAN_POINT ( 'NONE',  ( 27.42305978988358461, 1.006780081163760610, -4.486390501344786230 ) ) ;
#5225=CARTESIAN_POINT ( 'NONE',  ( 36.68443910100898364, -1.916675254377900872, -5.804134546349906998 ) ) ;
#5229=CARTESIAN_POINT ( 'NONE',  ( -71.84395654979768153, -48.30921343784671507, 5.930300998046988958 ) ) ;
#5233=CARTESIAN_POINT ( 'NONE',  ( 24.22011166491034473, 2.157244859911064960, -4.307574350163300814 ) ) ;
#5234=VECTOR ( 'NONE', #26582, 1000.000000000000000 ) ;
#5246=CIRCLE ( 'NONE', #34197, 12.80480339192541628 ) ;
#5251=CARTESIAN_POINT ( 'NONE',  ( 16.63788139911590847, 9.878167360688344445, -2.500000000000113243 ) ) ;
#5256=CARTESIAN_POINT ( 'NONE',  ( 15.61831370365439930, 11.17526387718623582, -2.611274213471738825 ) ) ;
#5258=CARTESIAN_POINT ( 'NONE',  ( 21.85643539959777826, -11.73360331217645225, -7.400322805736739618 ) ) ;
#5262=CARTESIAN_POINT ( 'NONE',  ( -73.66622939153592142, 5.992931831121631525, -9.675836161015377357 ) ) ;
#5277=CARTESIAN_POINT ( 'NONE',  ( -69.47640242684072120, -47.50614603290127036, 5.821697485475862521 ) ) ;
#5279=CARTESIAN_POINT ( 'NONE',  ( 32.78150442608843207, -0.9262738374823473730, 5.322744608008340705 ) ) ;
#5283=CARTESIAN_POINT ( 'NONE',  ( 85.86339947292255204, 1.596523033150343718, -5.427711696011725984 ) ) ;
#5285=CARTESIAN_POINT ( 'NONE',  ( 33.89705139301766224, -5.463269898809035574, -0.9834710557593000502 ) ) ;
#5288=CARTESIAN_POINT ( 'NONE',  ( 85.80507661318331714, 1.187011356922548666, 5.731706916149471809 ) ) ;
#5295=ADVANCED_FACE ( 'NONE', ( #10513 ), #23093, .F. ) ;
#5297=CARTESIAN_POINT ( 'NONE',  ( 22.33770448043473777, 0.2832778397994459296, 7.020340292902776724 ) ) ;
#5306=CARTESIAN_POINT ( 'NONE',  ( 14.77315594796471743, 13.19392823276620419, 2.499999999999996891 ) ) ;
#5310=CARTESIAN_POINT ( 'NONE',  ( 22.63677108660874637, 4.537383518013977657, -3.128882317202244856 ) ) ;
#5313=CARTESIAN_POINT ( 'NONE',  ( 23.92064240948634790, 4.179079982057642972, -0.5982227118658990372 ) ) ;
#5316=ADVANCED_FACE ( 'NONE', ( #21211 ), #12126, .T. ) ;
#5320=CARTESIAN_POINT ( 'NONE',  ( 84.60690941119878516, 3.085063967761199066, 1.108375916024202379 ) ) ;
#5324=CARTESIAN_POINT ( 'NONE',  ( -0.000000000000000000, 10.37661300689600097, -6.000000000000000000 ) ) ;
#5325=CARTESIAN_POINT ( 'NONE',  ( 19.68021815578885736, -2.835469129926569742, -3.275245259520223939 ) ) ;
#5328=CARTESIAN_POINT ( 'NONE',  ( 23.09295755050888843, 0.3657069220331809478, -5.919601208922279589 ) ) ;
#5331=CARTESIAN_POINT ( 'NONE',  ( 35.78599988003760757, -3.160010335899736678, 5.791668787594319134 ) ) ;
#5332=AXIS2_PLACEMENT_3D ( 'NONE', #5211, #16787, #36503 ) ;
#5333=CARTESIAN_POINT ( 'NONE',  ( 87.18327248044521127, 0.4293349789342923994, 4.780712506200352152 ) ) ;
#5337=CARTESIAN_POINT ( 'NONE',  ( 36.20129013013437458, -3.652211045159744707, 5.717050583165211641 ) ) ;
#5339=CARTESIAN_POINT ( 'NONE',  ( 17.38677253544971890, -3.246026456844883334, -2.884626868749156969 ) ) ;
#5343=VERTEX_POINT ( 'NONE', #11919 ) ;
#5346=ORIENTED_EDGE ( 'NONE', *, *, #39305, .F. ) ;
#5350=VERTEX_POINT ( 'NONE', #11713 ) ;
#5353=CARTESIAN_POINT ( 'NONE',  ( 23.65230220904194525, 3.215211265575084187, 3.706123801245496008 ) ) ;
#5358=DIRECTION ( 'NONE',  ( -0.000000000000000000, 1.000000000000000000, -0.000000000000000000 ) ) ;
#5360=PLANE ( 'NONE',  #7338 ) ;
#5362=CARTESIAN_POINT ( 'NONE',  ( 24.16851685081003254, 2.882859430398138301, -3.821847350340896288 ) ) ;
#5364=CYLINDRICAL_SURFACE ( 'NONE', #37247, 12.73502530973474123 ) ;
#5365=DIRECTION ( 'NONE',  ( 0.000000000000000000, 0.000000000000000000, -1.000000000000000000 ) ) ;
#5369=CARTESIAN_POINT ( 'NONE',  ( 85.29288036551089647, 2.552713125850948117, 2.517437320556888736 ) ) ;
#5373=CARTESIAN_POINT ( 'NONE',  ( 1.700390093233090871, -29.56993018339339940, 2.499999999999998668 ) ) ;
#5375=VECTOR ( 'NONE', #10061, 1000.000000000000000 ) ;
#5376=CARTESIAN_POINT ( 'NONE',  ( 35.33511153101647295, -3.174037457546911689, -5.721296755953630964 ) ) ;
#5384=CARTESIAN_POINT ( 'NONE',  ( 36.19298715789191334, -3.601780938441950575, 5.745406905112727891 ) ) ;
#5388=DIRECTION ( 'NONE',  ( 0.000000000000000000, -0.000000000000000000, 1.000000000000000000 ) ) ;
#5393=CARTESIAN_POINT ( 'NONE',  ( 14.84235502726276934, 12.12055237356136139, 2.522906484353911960 ) ) ;
#5394=CARTESIAN_POINT ( 'NONE',  ( -77.19718645414111791, 10.97120867451975279, 7.801112875662933099 ) ) ;
#5397=ORIENTED_EDGE ( 'NONE', *, *, #20884, .F. ) ;
#5398=CARTESIAN_POINT ( 'NONE',  ( 22.88074270852006009, 4.309495562975050653, 3.097908743967009659 ) ) ;
#5399=ADVANCED_FACE ( 'NONE', ( #17692, #30272 ), #5360, .T. ) ;
#5403=DIRECTION ( 'NONE',  ( 1.000000000000000000, 5.786005779812646808E-17, 0.000000000000000000 ) ) ;
#5406=CARTESIAN_POINT ( 'NONE',  ( 21.78353409329961465, 0.2137358133367803226, 8.397885858698352024 ) ) ;
#5407=CARTESIAN_POINT ( 'NONE',  ( 14.74007919223407370, -5.059642873582679279, -2.500266452831745312 ) ) ;
#5410=ORIENTED_EDGE ( 'NONE', *, *, #27668, .T. ) ;
#5411=VECTOR ( 'NONE', #3353, 1000.000000000000000 ) ;
#5413=CARTESIAN_POINT ( 'NONE',  ( 36.28349705958110150, -3.620525866554765049, -5.741672296196851377 ) ) ;
#5416=CARTESIAN_POINT ( 'NONE',  ( 87.04213330793392345, 0.5878691963682337596, -6.000000000000000000 ) ) ;
#5417=CARTESIAN_POINT ( 'NONE',  ( 31.27801355750085222, -2.827678977088778911, 5.603419278764796729 ) ) ;
#5421=CARTESIAN_POINT ( 'NONE',  ( 23.07493962920425190, 0.3584799070873228577, -5.937310339541745030 ) ) ;
#5427=CARTESIAN_POINT ( 'NONE',  ( 37.17546804304686248, -2.565784879737412982, -5.981171206039050503 ) ) ;
#5436=CARTESIAN_POINT ( 'NONE',  ( 24.70371381655884591, 2.049716166645646265, -4.246171004526042125 ) ) ;
#5438=CARTESIAN_POINT ( 'NONE',  ( -70.73084030234451802, -48.60722628301608950, 5.997527803321491824 ) ) ;
#5444=CARTESIAN_POINT ( 'NONE',  ( 86.71282820137585645, -0.9518751250403653108, -5.452277641718156431 ) ) ;
#5446=CARTESIAN_POINT ( 'NONE',  ( -70.92837670882107659, -48.61702805680358352, 10.00000000000000888 ) ) ;
#5459=CARTESIAN_POINT ( 'NONE',  ( 20.30405656617691434, 6.129814585338576371, -3.484773916750472100 ) ) ;
#5463=CARTESIAN_POINT ( 'NONE',  ( 22.77685072273605371, 3.733082073155330249, 3.761276434136069380 ) ) ;
#5464=CARTESIAN_POINT ( 'NONE',  ( 18.67745381493141110, 13.05554818434302966, 2.500000000000000000 ) ) ;
#5465=CARTESIAN_POINT ( 'NONE',  ( 21.85643539959777470, -5.354795180264900978, -13.61019886989645933 ) ) ;
#5466=VERTEX_POINT ( 'NONE', #18935 ) ;
#5467=CARTESIAN_POINT ( 'NONE',  ( -80.85729187619890013, 11.46329443280617788, 1.443597705564378053 ) ) ;
#5468=AXIS2_PLACEMENT_3D ( 'NONE', #34692, #33867, #3203 ) ;
#5469=CARTESIAN_POINT ( 'NONE',  ( -77.61396521033491069, 9.844637789582655785, -7.450128154136889336 ) ) ;
#5473=CARTESIAN_POINT ( 'NONE',  ( 14.65544684909820461, 12.77405410657241092, 2.493734942759960660 ) ) ;
#5475=CARTESIAN_POINT ( 'NONE',  ( -69.92837670882107659, -0.7829914368874778541, 9.949874371066204759 ) ) ;
#5479=CARTESIAN_POINT ( 'NONE',  ( 87.33194808155565170, 0.2623354871973614388, 4.590518720782623241 ) ) ;
#5480=CARTESIAN_POINT ( 'NONE',  ( 24.74244792756189426, 2.626221424013070571, -3.930118435553313638 ) ) ;
#5482=VERTEX_POINT ( 'NONE', #21622 ) ;
#5484=CARTESIAN_POINT ( 'NONE',  ( 36.44794194783038677, -2.352442707074569928, 5.894980856402876945 ) ) ;
#5487=CARTESIAN_POINT ( 'NONE',  ( 87.83080901603209156, -0.9320485544948414747, 4.955211484752597428 ) ) ;
#5499=CARTESIAN_POINT ( 'NONE',  ( 22.66994700586167255, 0.3178347913156189253, 6.420626853764989761 ) ) ;
#5506=DIRECTION ( 'NONE',  ( -1.000000000000000000, 0.000000000000000000, 0.000000000000000000 ) ) ;
#5510=CARTESIAN_POINT ( 'NONE',  ( 22.02803121022057198, 5.433847407666364759, -3.182498588599022238 ) ) ;
#5513=B_SPLINE_CURVE_WITH_KNOTS ( 'NONE', 3,
 ( #21854, #18752, #9478, #18966, #3752, #22681, #38296, #2942, #31530, #15458, #28018, #34430, #6209, #3153, #15668, #28216, #46, #12575, #13595, #25962, #32946, #35444, #7616, #32549, #4348, #26167, #38494, #1263, #36038, #26561, #4734, #7214, #10297, #3956, #19778, #19969, #4147, #17267, #23660, #32353, #17066, #29251, #32158, #1061, #38699, #10494, #16871, #13988, #29645, #23076, #855, #35643, #29451, #13385, #29841, #1656, #26367, #38900, #26764, #36228, #7413, #14191, #13800, #35841, #10694, #39303, #20170, #32753 ),
 .UNSPECIFIED., .F., .F.,
 ( 4, 2, 2, 2, 2, 2, 2, 1, 1, 2, 2, 2, 2, 2, 2, 2, 2, 2, 1, 1, 2, 2, 1, 1, 2, 2, 2, 2, 1, 1, 2, 2, 2, 1, 2, 2, 1, 2, 4 ),
 ( 0.000000000000000000, 0.03012276342170286392, 0.06024552684340572090, 0.09036829026510857787, 0.1204910536868114279, 0.1242563991145242547, 0.1251977354714524926, 0.1261390718283807444, 0.1280217445422372202, 0.1355524353976629293, 0.1506138171085143196, 0.1807365805302170170, 0.2409821073736224395, 0.2485127982290481208, 0.2560434890844738853, 0.2711048707953253034, 0.3012276342170281396, 0.3614731610604337009, 0.3690038519158592711, 0.3727691973435722783, 0.3746518700574291150, 0.3751225382358933658, 0.3755932064143576166, 0.3765345427712861182, 0.3915959244821413110, 0.4217186879038513081, 0.4367800696147063344, 0.4377214059716350025, 0.4386627423285636707, 0.4405454150424208404, 0.4443107604701349578, 0.4518414513255630260, 0.4669028330364197732, 0.4678441693933488854, 0.4683148375718130807, 0.4687855057502772760, 0.4706681784641342237, 0.4744335238918481190, 0.4819642147472753546 ),
 .UNSPECIFIED. ) ;
#5514=CARTESIAN_POINT ( 'NONE',  ( 25.11613067079463590, -2.903500246237137983, -5.705645831387469613 ) ) ;
#5515=CARTESIAN_POINT ( 'NONE',  ( 0.7201709579117279159, -51.60714625320436255, 6.000000000000000000 ) ) ;
#5518=CARTESIAN_POINT ( 'NONE',  ( 86.79384979562775015, -0.7021008148363506729, 5.624057257660853182 ) ) ;
#5525=CARTESIAN_POINT ( 'NONE',  ( 18.23157317310702652, -3.007012085376574717, -3.040421556899932209 ) ) ;
#5531=CARTESIAN_POINT ( 'NONE',  ( 30.51366675730394817, -0.1447508928393422822, 4.968793691933281131 ) ) ;
#5540=CARTESIAN_POINT ( 'NONE',  ( 35.73138356448509256, -1.302398868511517760, 5.536388820249604770 ) ) ;
#5541=CARTESIAN_POINT ( 'NONE',  ( 18.10821205226829278, -2.857188514361614473, 3.032622458156649881 ) ) ;
#5542=CARTESIAN_POINT ( 'NONE',  ( 22.07542296685559435, -3.076855778316415879, -3.556068286084799190 ) ) ;
#5543=ORIENTED_EDGE ( 'NONE', *, *, #4389, .T. ) ;
#5551=CARTESIAN_POINT ( 'NONE',  ( 14.75654458176583006, -5.136929176716047429, 2.500022312476919417 ) ) ;
#5553=CARTESIAN_POINT ( 'NONE',  ( 22.70712101228993873, 2.614415518154956430, 4.662403001875633279 ) ) ;
#5554=CARTESIAN_POINT ( 'NONE',  ( -12.99139449055068241, -10.90558813203967148, 2.500000000000000000 ) ) ;
#5559=CARTESIAN_POINT ( 'NONE',  ( 26.18165949521383951, -2.762208175416757339, -4.292679188692566150 ) ) ;
#5562=CARTESIAN_POINT ( 'NONE',  ( 23.71103289728280927, 3.002135961463958669, -3.868039065086897654 ) ) ;
#5564=CARTESIAN_POINT ( 'NONE',  ( 21.85643539959777470, 9.109670159223330899, 10.09094178405049647 ) ) ;
#5571=CARTESIAN_POINT ( 'NONE',  ( 86.87490948991990081, 0.7757029256828257280, 5.355124474773749199 ) ) ;
#5574=AXIS2_PLACEMENT_3D ( 'NONE', #22279, #34849, #28221 ) ;
#5576=CARTESIAN_POINT ( 'NONE',  ( 33.95810710317707759, -3.751921607304459005, 5.289039422336568208 ) ) ;
#5578=CARTESIAN_POINT ( 'NONE',  ( 36.42103784419850143, -3.116709639155254674, -5.890781820352805731 ) ) ;
#5584=EDGE_CURVE ( 'NONE', #16788, #5201, #2789, .T. ) ;
#5586=CARTESIAN_POINT ( 'NONE',  ( -69.79879845479261746, -46.12525168278317977, 5.893131031833197753 ) ) ;
#5588=CARTESIAN_POINT ( 'NONE',  ( 35.82506826730624283, -3.676139994978682601, 5.658754788095917476 ) ) ;
#5596=CIRCLE ( 'NONE', #31239, 8.080217238368755162 ) ;
#5599=CARTESIAN_POINT ( 'NONE',  ( 15.12608719890447695, 11.51997479474082020, 2.567189751827102295 ) ) ;
#5600=CARTESIAN_POINT ( 'NONE',  ( -80.85559708689355318, 11.46349645673830686, 1.470518245667309376 ) ) ;
#5607=CARTESIAN_POINT ( 'NONE',  ( 21.71895566332458571, 6.267330856689260266, 3.214934355689595957 ) ) ;
#5613=CARTESIAN_POINT ( 'NONE',  ( 22.29093078930348781, 0.2567994035360497973, 7.116204519797545203 ) ) ;
#5622=CARTESIAN_POINT ( 'NONE',  ( 30.65010716405877034, -0.4808061152566996399, -5.754690052858093097 ) ) ;
#5626=CARTESIAN_POINT ( 'NONE',  ( 24.73872378485249968, 0.6063834911445746823, -4.778905198491438355 ) ) ;
#5634=CARTESIAN_POINT ( 'NONE',  ( -72.42837670882107659, -47.11702805680359063, 9.886859966642603581 ) ) ;
#5635=CARTESIAN_POINT ( 'NONE',  ( 37.08867879065032724, -2.428124687478105947, -5.958193899595366716 ) ) ;
#5640=CARTESIAN_POINT ( 'NONE',  ( -62.92837670882106238, -23.80776546975053520, 6.000000000000000000 ) ) ;
#5645=CARTESIAN_POINT ( 'NONE',  ( 25.15062346579604480, 2.408171519380073899, -4.029033621008475841 ) ) ;
#5652=CARTESIAN_POINT ( 'NONE',  ( 84.69769694898896262, 2.275084749292730635, 4.163914512140848068 ) ) ;
#5659=CARTESIAN_POINT ( 'NONE',  ( 22.18507716018001474, 5.290272291513682390, 3.054672883570451081 ) ) ;
#5660=CARTESIAN_POINT ( 'NONE',  ( 22.64483291760767258, -3.096555847357584934, 3.637248286138076825 ) ) ;
#5671=CARTESIAN_POINT ( 'NONE',  ( 22.63946314531691328, -3.430231901737621492, -8.286483013797429464 ) ) ;
#5675=CARTESIAN_POINT ( 'NONE',  ( -77.86806181146356209, 9.955796112368622275, -7.213709624780306306 ) ) ;
#5677=CARTESIAN_POINT ( 'NONE',  ( 37.00868671504413498, -3.246586382702952633, -5.946932760037821453 ) ) ;
#5679=CARTESIAN_POINT ( 'NONE',  ( 15.37661900244130209, 11.52640166518511222, 2.577936354164439781 ) ) ;
#5683=EDGE_CURVE ( 'NONE', #13567, #10739, #17236, .T. ) ;
#5685=CARTESIAN_POINT ( 'NONE',  ( 18.18564233718114664, 13.54291529513208125, -2.500000000000000444 ) ) ;
#5686=CARTESIAN_POINT ( 'NONE',  ( 37.20079544340044464, -2.795532513595198054, -5.999424151161432128 ) ) ;
#5688=CARTESIAN_POINT ( 'NONE',  ( 24.35226569962506815, 2.912787986373579052, -3.759256437568978093 ) ) ;
#5692=CARTESIAN_POINT ( 'NONE',  ( 23.01849606021741579, 2.906675443451126384, 3.798991033265373130 ) ) ;
#5693=DIRECTION ( 'NONE',  ( -0.9999026450364576490, -0.01395351027862084224, 0.000000000000000000 ) ) ;
#5696=CARTESIAN_POINT ( 'NONE',  ( 85.01740037914012760, 2.610285099004062470, -3.580537606963684283 ) ) ;
#5697=CARTESIAN_POINT ( 'NONE',  ( 32.62845853548997610, -2.537451394787784142, 5.899574533259067444 ) ) ;
#5700=CARTESIAN_POINT ( 'NONE',  ( 11.29080664838498649, 1.564594260697056104E-15, -6.000000000000000000 ) ) ;
#5720=CARTESIAN_POINT ( 'NONE',  ( 22.05245566893604092, 5.319511344851127532, -3.238308893631721919 ) ) ;
#5724=CARTESIAN_POINT ( 'NONE',  ( 26.57131730419879290, 2.962615056577905026, -1.092182624680714254 ) ) ;
#5725=CARTESIAN_POINT ( 'NONE',  ( 23.31126753349915504, 9.638235383039575055, 2.500000000000000444 ) ) ;
#5728=CARTESIAN_POINT ( 'NONE',  ( 86.59537683758360060, -0.3992097724244685342, -5.811584838773467432 ) ) ;
#5729=CARTESIAN_POINT ( 'NONE',  ( 15.36874315909924249, 11.54028096791004998, 2.577200810392474839 ) ) ;
#5730=VERTEX_POINT ( 'NONE', #4512 ) ;
#5732=CARTESIAN_POINT ( 'NONE',  ( -72.05775109714784321, -46.12502802752712938, 9.936264230343166304 ) ) ;
#5733=CARTESIAN_POINT ( 'NONE',  ( 0.000000000000000000, 0.000000000000000000, -6.000000000000000000 ) ) ;
#5734=CARTESIAN_POINT ( 'NONE',  ( 31.36895993190770682, -3.421856983129734964, -5.044461153598384762 ) ) ;
#5737=CARTESIAN_POINT ( 'NONE',  ( 85.67377067720147465, 0.8449287747730311882, 5.870810042200333534 ) ) ;
#5740=CARTESIAN_POINT ( 'NONE',  ( 88.26779375368444391, -0.7888507896528732521, -1.681504516799547710 ) ) ;
#5744=CARTESIAN_POINT ( 'NONE',  ( 36.71960778968895056, -3.460346308713754038, 5.859997665240682885 ) ) ;
#5745=CARTESIAN_POINT ( 'NONE',  ( 26.16557211405898187, -2.761525329003165830, 4.290168363788568584 ) ) ;
#5747=CARTESIAN_POINT ( 'NONE',  ( 22.02893036045224662, -3.075429753726866888, -3.549435909675389578 ) ) ;
#5758=EDGE_CURVE ( 'NONE', #25658, #23544, #29419, .T. ) ;
#5759=CARTESIAN_POINT ( 'NONE',  ( 22.04698793031429105, 2.546066460137037524, 5.281988517684759188 ) ) ;
#5760=CARTESIAN_POINT ( 'NONE',  ( 31.36572658741310704, 0.5137713814500121101, 4.593329244990838056 ) ) ;
#5771=CARTESIAN_POINT ( 'NONE',  ( 23.46071017023546901, 3.155770004481628810, -3.834925600461499773 ) ) ;
#5775=CARTESIAN_POINT ( 'NONE',  ( 21.85643539959778181, 11.38078789530947788, 4.862784767728865809 ) ) ;
#5777=ORIENTED_EDGE ( 'NONE', *, *, #23425, .F. ) ;
#5779=CARTESIAN_POINT ( 'NONE',  ( 88.53816506398004549, -1.092544677973264378, 2.020403607635292254 ) ) ;
#5780=LINE ( 'NONE', #30909, #25421 ) ;
#5783=CARTESIAN_POINT ( 'NONE',  ( 31.36983548603388527, -3.544126911492940568, 4.957555829163103667 ) ) ;
#5784=CARTESIAN_POINT ( 'NONE',  ( 21.54940507516195680, 7.328906648784134781, -1.954559343662467308 ) ) ;
#5786=CARTESIAN_POINT ( 'NONE',  ( 27.40856500620434488, 0.9677877529870252404, -4.484167466504554334 ) ) ;
#5794=CARTESIAN_POINT ( 'NONE',  ( 33.91383790368941931, -0.5462175910584815552, 5.194263850780147074 ) ) ;
#5804=CARTESIAN_POINT ( 'NONE',  ( 14.93041183113045278, 11.91532239571927221, 2.536649878259312541 ) ) ;
#5809=CARTESIAN_POINT ( 'NONE',  ( 21.86077673335558202, 5.786921160339534964, 3.210078130593202683 ) ) ;
#5816=CARTESIAN_POINT ( 'NONE',  ( -72.42837670882109080, -47.01877623127393946, 5.809475019311129529 ) ) ;
#5824=CARTESIAN_POINT ( 'NONE',  ( -62.92837670882106238, 10.37661300689600097, -6.000000000000000000 ) ) ;
#5827=PLANE ( 'NONE',  #6671 ) ;
#5830=CARTESIAN_POINT ( 'NONE',  ( 33.42314280165584961, -3.731500252021894948, -5.214789010484834897 ) ) ;
#5834=CARTESIAN_POINT ( 'NONE',  ( 22.00567502167365319, 0.2472497164922489998, -7.635414579327273188 ) ) ;
#5837=FACE_OUTER_BOUND ( 'NONE', #30901, .T. ) ;
#5842=CARTESIAN_POINT ( 'NONE',  ( 27.74723518964530555, 1.752444360904438225, -4.134722068930840599 ) ) ;
#5848=CARTESIAN_POINT ( 'NONE',  ( -73.82198138812172772, 6.296306154009471356, 10.81584845386062810 ) ) ;
#5850=CIRCLE ( 'NONE', #12424, 10.00000000000000888 ) ;
#5852=CARTESIAN_POINT ( 'NONE',  ( 22.99834754057519248, 2.264180960916559293, -4.739916070323666020 ) ) ;
#5854=ORIENTED_EDGE ( 'NONE', *, *, #11768, .F. ) ;
#5856=DIRECTION ( 'NONE',  ( -0.000000000000000000, 0.000000000000000000, 1.000000000000000000 ) ) ;
#5860=CARTESIAN_POINT ( 'NONE',  ( 87.93534175303985023, -2.522256948347837202, 0.2133659395812929627 ) ) ;
#5861=CARTESIAN_POINT ( 'NONE',  ( 21.85643539959776760, -15.11427361947482062, -2.500000000000000000 ) ) ;
#5862=CARTESIAN_POINT ( 'NONE',  ( 21.63674588113149611, 6.916792737387225110, 2.999788494245204440 ) ) ;
#5866=VERTEX_POINT ( 'NONE', #27124 ) ;
#5867=CARTESIAN_POINT ( 'NONE',  ( 23.75598750291871042, 3.574640555080575322, 3.141240283659741284 ) ) ;
#5875=EDGE_CURVE ( 'NONE', #16084, #17878, #1620, .T. ) ;
#5879=CARTESIAN_POINT ( 'NONE',  ( 22.32070839933769690, 6.022037317923602195, -2.674548383380369376 ) ) ;
#5881=CARTESIAN_POINT ( 'NONE',  ( -76.33961693584673469, 9.111181514875148935, 8.435660748604236758 ) ) ;
#5882=CARTESIAN_POINT ( 'NONE',  ( 37.04963165681110127, -3.191030522870556219, 5.959957271559491510 ) ) ;
#5886=CARTESIAN_POINT ( 'NONE',  ( 32.91122043559692401, -3.130653418612100225, -5.342989928665543786 ) ) ;
#5887=CARTESIAN_POINT ( 'NONE',  ( 35.36827583184471990, -3.794046567535431347, -5.509537208948445119 ) ) ;
#5891=CARTESIAN_POINT ( 'NONE',  ( 21.85643539959776760, 1.710603452083953179E-15, 2.500000000000000000 ) ) ;
#5894=CARTESIAN_POINT ( 'NONE',  ( 37.19853941620289106, -2.831595418823658061, -6.000000013228142137 ) ) ;
#5895=CARTESIAN_POINT ( 'NONE',  ( 24.52768585756376751, 2.971958902176091044, -3.615748989836667704 ) ) ;
#5898=CARTESIAN_POINT ( 'NONE',  ( 37.07722502896399419, -2.790003627308526468, 5.993195700482429444 ) ) ;
#5903=CARTESIAN_POINT ( 'NONE',  ( 87.00256539079671825, 0.09090593131677454641, 5.889906316148251442 ) ) ;
#5904=CARTESIAN_POINT ( 'NONE',  ( -71.80179680180437174, -21.28723728285361005, 5.936304882227263491 ) ) ;
#5905=CARTESIAN_POINT ( 'NONE',  ( 35.96793650919964591, -2.128746960111746134, -5.820064398729031474 ) ) ;
#5907=CARTESIAN_POINT ( 'NONE',  ( 24.70447383357791793, 2.647224887469914467, 3.920167867705436571 ) ) ;
#5915=DIRECTION ( 'NONE',  ( 0.000000000000000000, 0.000000000000000000, -1.000000000000000000 ) ) ;
#5924=CARTESIAN_POINT ( 'NONE',  ( -71.43192785570207093, -21.65683240571980406, 9.988048282181825499 ) ) ;
#5925=CARTESIAN_POINT ( 'NONE',  ( 33.89873586150555695, -5.477242531774048295, 0.02003360515015548127 ) ) ;
#5926=CARTESIAN_POINT ( 'NONE',  ( 22.23079900249558349, 5.088912589733261882, -3.182692338938402532 ) ) ;
#5927=ORIENTED_EDGE ( 'NONE', *, *, #12119, .F. ) ;
#5930=CARTESIAN_POINT ( 'NONE',  ( -77.11750342460615570, -4.735368223276241295, -7.872399780471171837 ) ) ;
#5933=CARTESIAN_POINT ( 'NONE',  ( 88.36353413610991936, -2.347965962749813063, -0.8794284646705250452 ) ) ;
#5939=AXIS2_PLACEMENT_3D ( 'NONE', #5554, #34399, #28181 ) ;
#5940=CARTESIAN_POINT ( 'NONE',  ( 28.89993508709290282, -3.472368636922807728, -4.526205258352716143 ) ) ;
#5941=CARTESIAN_POINT ( 'NONE',  ( 33.62640329583895493, -1.235465025675091422, -5.454611510589393752 ) ) ;
#5944=CARTESIAN_POINT ( 'NONE',  ( 36.42068411451688092, -3.113243699955915211, 5.890726612280997365 ) ) ;
#5948=CARTESIAN_POINT ( 'NONE',  ( 27.81821396243497091, 1.847154100788544140, 3.899782868931562785 ) ) ;
#5949=CARTESIAN_POINT ( 'NONE',  ( 22.11550089188394352, -2.652446215743125002, 3.658056798225496564 ) ) ;
#5950=CARTESIAN_POINT ( 'NONE',  ( -70.92837670882107659, -45.61702805680359063, 10.00000000000000888 ) ) ;
#5952=ORIENTED_EDGE ( 'NONE', *, *, #19722, .F. ) ;
#5953=CARTESIAN_POINT ( 'NONE',  ( 28.37783869506044354, -4.100928795493604007, -4.014438774076839245 ) ) ;
#5954=VERTEX_POINT ( 'NONE', #33941 ) ;
#5958=VERTEX_POINT ( 'NONE', #36598 ) ;
#5959=CARTESIAN_POINT ( 'NONE',  ( 24.37905646352311351, 2.670070934302906540, 3.939568903014517343 ) ) ;
#5961=ORIENTED_EDGE ( 'NONE', *, *, #13331, .F. ) ;
#5969=CARTESIAN_POINT ( 'NONE',  ( 86.88012133546156690, 0.7698487334013246475, -5.007445623867876172 ) ) ;
#5974=CARTESIAN_POINT ( 'NONE',  ( 22.43120517420025806, 3.420092575442463367, -4.253115007774507461 ) ) ;
#5975=ORIENTED_EDGE ( 'NONE', *, *, #37729, .T. ) ;
#5977=CARTESIAN_POINT ( 'NONE',  ( 21.85643539959778892, 11.01376456104441104, -6.033145431426138572 ) ) ;
#5984=CARTESIAN_POINT ( 'NONE',  ( 88.28392341775159480, -0.8069683938931414557, -2.555979571574120257 ) ) ;
#5989=CARTESIAN_POINT ( 'NONE',  ( 14.68417304430366066, -5.052781308733836241, 2.495429214815205299 ) ) ;
#5991=CARTESIAN_POINT ( 'NONE',  ( 25.34284313847354397, 1.862862106151733643, -4.161761609372907067 ) ) ;
#5996=CARTESIAN_POINT ( 'NONE',  ( 21.79071535907295498, 5.485802459903661443, -3.529903039149067556 ) ) ;
#5997=CARTESIAN_POINT ( 'NONE',  ( -69.46739714565912038, -46.72383415856366895, 5.819932703929897144 ) ) ;
#6001=CARTESIAN_POINT ( 'NONE',  ( 36.65981812739566692, -1.958039781240433763, 5.826225346727439636 ) ) ;
#6005=ADVANCED_FACE ( 'NONE', ( #17637 ), #30642, .T. ) ;
#6007=CARTESIAN_POINT ( 'NONE',  ( 87.73487586818573902, -0.1902521268519785647, -3.837085321992326659 ) ) ;
#6008=CARTESIAN_POINT ( 'NONE',  ( -72.89579999368469032, 7.037834574950979416, -9.806287887461893504 ) ) ;
#6009=CARTESIAN_POINT ( 'NONE',  ( 22.01622206693788897, 4.835086392017111656, 3.641232820207879417 ) ) ;
#6014=CARTESIAN_POINT ( 'NONE',  ( 21.72140077180526418, 6.245282651313772249, 3.222889655586078206 ) ) ;
#6021=CARTESIAN_POINT ( 'NONE',  ( 14.61151433092574159, 13.01680870242209487, -2.486878210787180965 ) ) ;
#6034=CARTESIAN_POINT ( 'NONE',  ( 32.02627343617642453, -1.895034194620857315, -5.999511542327915947 ) ) ;
#6035=DIRECTION ( 'NONE',  ( -0.000000000000000000, 0.000000000000000000, 1.000000000000000000 ) ) ;
#6036=CARTESIAN_POINT ( 'NONE',  ( 30.76573472615519833, -3.583077396579174234, 4.803740791053209058 ) ) ;
#6038=CARTESIAN_POINT ( 'NONE',  ( 22.63464106450162916, 0.3019483094031678028, -6.468809234137039788 ) ) ;
#6044=CARTESIAN_POINT ( 'NONE',  ( 36.63484890502185465, -2.000711152530542325, -5.847404196664919951 ) ) ;
#6046=CARTESIAN_POINT ( 'NONE',  ( -12.99139449055068596, 10.37661300689600097, -2.500000000000000444 ) ) ;
#6063=CARTESIAN_POINT ( 'NONE',  ( 21.85643539959776760, -15.25441669702287939, -1.357504026734941416 ) ) ;
#6068=CARTESIAN_POINT ( 'NONE',  ( 22.18581564090588643, 5.276225145155845730, 3.069190463584780204 ) ) ;
#6076=DIRECTION ( 'NONE',  ( 1.000000000000000000, 0.000000000000000000, 0.000000000000000000 ) ) ;
#6079=CARTESIAN_POINT ( 'NONE',  ( 21.85643539959775694, 4.180186707270823199, 11.06385087694989799 ) ) ;
#6082=CARTESIAN_POINT ( 'NONE',  ( -73.27055294303096389, 7.677084106314387313, 9.725186251795168602 ) ) ;
#6084=EDGE_CURVE ( 'NONE', #20746, #14452, #16946, .T. ) ;
#6086=CARTESIAN_POINT ( 'NONE',  ( -80.90823458386326195, 10.55951580149532809, 0.6344085041158121774 ) ) ;
#6087=CARTESIAN_POINT ( 'NONE',  ( 32.91903012308263499, -3.045910662517542722, -5.344208819095712215 ) ) ;
#6088=CARTESIAN_POINT ( 'NONE',  ( 21.74038104888381895, 4.236694489823714882, -2.795633211743734581 ) ) ;
#6089=APPLICATION_CONTEXT ( 'automotive_design' ) ;
#6091=CARTESIAN_POINT ( 'NONE',  ( 14.62323830247504119, 13.01685296470267517, 2.488708020092772699 ) ) ;
#6093=CARTESIAN_POINT ( 'NONE',  ( 30.07655335801453234, -3.716434046306707373, 4.568522214145315452 ) ) ;
#6096=CARTESIAN_POINT ( 'NONE',  ( 18.41743161276554019, 13.31819020379082197, -2.500000000000000000 ) ) ;
#6097=CARTESIAN_POINT ( 'NONE',  ( 25.33510812559238801, 0.7739518545062052945, -4.607785389428086020 ) ) ;
#6098=CARTESIAN_POINT ( 'NONE',  ( 36.48031136538276087, -1.766077765691559831, -5.744066426338735099 ) ) ;
#6099=CARTESIAN_POINT ( 'NONE',  ( 24.35746132025820287, 2.925223658202782406, -3.744337438357647319 ) ) ;
#6102=EDGE_CURVE ( 'NONE', #36975, #15644, #7951, .T. ) ;
#6103=CARTESIAN_POINT ( 'NONE',  ( 30.55148721072670881, -0.03398917485607633182, 4.974696488381029624 ) ) ;
#6107=CARTESIAN_POINT ( 'NONE',  ( 84.68420644151177612, 2.996072101527111453, 1.894685230139086851 ) ) ;
#6111=CARTESIAN_POINT ( 'NONE',  ( 24.71577694999333374, 3.003426287302215947, 3.428006812919407231 ) ) ;
#6124=EDGE_LOOP ( 'NONE', ( #40131, #15007, #3733, #16778 ) ) ;
#6131=CARTESIAN_POINT ( 'NONE',  ( 21.87171821392831461, 5.720550014221652546, -3.238356660519563501 ) ) ;
#6133=CARTESIAN_POINT ( 'NONE',  ( 24.68629359590044459, -1.668547755296895696, 6.687296101055469677 ) ) ;
#6134=CARTESIAN_POINT ( 'NONE',  ( -76.78746716544362982, -5.933295494910943546, -8.113055081387594569 ) ) ;
#6137=CARTESIAN_POINT ( 'NONE',  ( 84.47734884986269321, 2.726878650076010491, -2.900369371603537694 ) ) ;
#6145=CARTESIAN_POINT ( 'NONE',  ( 16.08354769902080506, -3.539635827824002767, -2.696278765112280151 ) ) ;
#6150=CARTESIAN_POINT ( 'NONE',  ( 36.19339270046786794, -2.233506198504079610, 5.855252290054989928 ) ) ;
#6154=CARTESIAN_POINT ( 'NONE',  ( 85.70831578087668845, 2.086076349557777654, 3.711011680213312403 ) ) ;
#6158=CARTESIAN_POINT ( 'NONE',  ( -69.73576780118902718, -46.20203278094625432, 9.928780194719321273 ) ) ;
#6159=CARTESIAN_POINT ( 'NONE',  ( 14.67067689388392360, 13.26234298596911287, -2.496111959588981133 ) ) ;
#6169=CARTESIAN_POINT ( 'NONE',  ( 24.81493965045673633, 2.585987335596099168, 3.949178272049961969 ) ) ;
#6170=CARTESIAN_POINT ( 'NONE',  ( 36.09228681445222264, -1.514627514507355333, 5.635688615691564429 ) ) ;
#6171=ORIENTED_EDGE ( 'NONE', *, *, #13948, .T. ) ;
#6176=CARTESIAN_POINT ( 'NONE',  ( -2.697268050091675118E-17, 3.729367930467589076, 6.000000000000000000 ) ) ;
#6180=CARTESIAN_POINT ( 'NONE',  ( 21.85662909133909082, 3.729105680040489812, -4.537925847320513739 ) ) ;
#6183=CARTESIAN_POINT ( 'NONE',  ( 21.85643539959774628, 7.825395393543534972, -11.66269361450695108 ) ) ;
#6188=CARTESIAN_POINT ( 'NONE',  ( 85.42332570945818304, 2.406190724219733568, -3.391956346677281076 ) ) ;
#6189=ORIENTED_EDGE ( 'NONE', *, *, #32745, .F. ) ;
#6192=CARTESIAN_POINT ( 'NONE',  ( 31.36247516317754247, -3.421439689148831231, 5.043473584804893939 ) ) ;
#6195=CARTESIAN_POINT ( 'NONE',  ( -2.697268050091675118E-17, 3.729367930467589076, -2.500000000000000000 ) ) ;
#6196=CARTESIAN_POINT ( 'NONE',  ( 25.29915376873320199, 1.743595656015987538, -4.154942826593681637 ) ) ;
#6206=CARTESIAN_POINT ( 'NONE',  ( 37.10374867307626801, -3.125519533824888452, 5.976337534025341292 ) ) ;
#6209=CARTESIAN_POINT ( 'NONE',  ( 87.67710904054415266, -2.211298689107902504, -2.754471170594727791 ) ) ;
#6218=CARTESIAN_POINT ( 'NONE',  ( 22.62405152208049941, 4.580528983382354369, 3.090851274182689679 ) ) ;
#6225=CARTESIAN_POINT ( 'NONE',  ( -72.37992470321633220, -46.72631451928356228, 5.821804174376780772 ) ) ;
#6227=CARTESIAN_POINT ( 'NONE',  ( 18.39501626872469231, 7.834513951104746354, -3.077385192520857071 ) ) ;
#6237=CARTESIAN_POINT ( 'NONE',  ( 29.95345716813442749, -1.222334143750352764, -6.038643835265099291 ) ) ;
#6241=CARTESIAN_POINT ( 'NONE',  ( 22.62321569360657136, 0.2992175222827407333, -6.483806668115875027 ) ) ;
#6242=DIRECTION ( 'NONE',  ( 0.7877517966954343809, -0.6159927814537400348, 0.000000000000000000 ) ) ;
#6244=CARTESIAN_POINT ( 'NONE',  ( 1.700390093233090871, -29.56993018339339940, -15.49999999999999822 ) ) ;
#6246=CARTESIAN_POINT ( 'NONE',  ( 23.34994961758268062, 3.524620780518698204, -3.233128968679401360 ) ) ;
#6256=AXIS2_PLACEMENT_3D ( 'NONE', #2464, #21586, #27545 ) ;
#6268=CARTESIAN_POINT ( 'NONE',  ( 24.75999223784396719, 3.019925347883366307, 3.347241732953214477 ) ) ;
#6273=CARTESIAN_POINT ( 'NONE',  ( 21.73607458324352137, 0.2916839156606184091, 8.911482056295868759 ) ) ;
#6283=CARTESIAN_POINT ( 'NONE',  ( 22.59998850301547790, -2.767621054697568361, -8.672491381162554802 ) ) ;
#6284=CARTESIAN_POINT ( 'NONE',  ( 4.938390203311415748E-15, -42.37473357531882101, -2.500000000000000000 ) ) ;
#6286=CARTESIAN_POINT ( 'NONE',  ( -72.02191131938369040, 0.007829945179003310052, 9.944423546733684560 ) ) ;
#6287=CARTESIAN_POINT ( 'NONE',  ( 33.45749450797183044, -3.829747548865578555, 5.093667367007288505 ) ) ;
#6293=CARTESIAN_POINT ( 'NONE',  ( -4.444218661349752963, -35.94265729135299381, 6.000000000000000000 ) ) ;
#6294=CARTESIAN_POINT ( 'NONE',  ( 33.11411321054668377, -0.1504196223776565200, -4.940960329838760323 ) ) ;
#6296=CARTESIAN_POINT ( 'NONE',  ( 21.28478389403105098, 5.337957506763612692, 3.528403319744038313 ) ) ;
#6297=DIRECTION ( 'NONE',  ( 1.000000000000000000, 0.000000000000000000, 0.000000000000000000 ) ) ;
#6301=CARTESIAN_POINT ( 'NONE',  ( 21.84750790989929570, 0.3413277259319377754, -8.043973749180381105 ) ) ;
#6302=CARTESIAN_POINT ( 'NONE',  ( 31.19141131379476306, -3.759815128464405021, -4.641892418952871857 ) ) ;
#6303=CARTESIAN_POINT ( 'NONE',  ( 24.45511755102040752, 2.961865972188622020, -3.664620675852518161 ) ) ;
#6305=EDGE_LOOP ( 'NONE', ( #17678, #13196, #16388, #15364 ) ) ;
#6307=CARTESIAN_POINT ( 'NONE',  ( 33.43848875257462083, -3.435003965559634942, 5.407914039447962118 ) ) ;
#6311=CARTESIAN_POINT ( 'NONE',  ( 86.59537683758360060, -0.3992097724244685342, -5.811584838773467432 ) ) ;
#6312=CARTESIAN_POINT ( 'NONE',  ( 35.93014311948857653, -3.156885213570711723, -5.814165826228037126 ) ) ;
#6315=CARTESIAN_POINT ( 'NONE',  ( 24.43316465493469636, 2.958069255867872727, 3.679139778253121662 ) ) ;
#6319=ORIENTED_EDGE ( 'NONE', *, *, #18792, .T. ) ;
#6321=CYLINDRICAL_SURFACE ( 'NONE', #39952, 21.28220113893567245 ) ;
#6331=CARTESIAN_POINT ( 'NONE',  ( 25.13391170364226923, -5.621210998728720654, 2.945584106497509236 ) ) ;
#6332=DIRECTION ( 'NONE',  ( -0.000000000000000000, -0.000000000000000000, -1.000000000000000000 ) ) ;
#6336=CARTESIAN_POINT ( 'NONE',  ( 22.88263960910827777, 4.299920287885681702, -3.109403903331433128 ) ) ;
#6342=DIRECTION ( 'NONE',  ( -1.682730792515357087E-16, 1.000000000000000000, 0.000000000000000000 ) ) ;
#6344=CARTESIAN_POINT ( 'NONE',  ( -77.62820146566370738, -4.987354577580212833, -7.432037137499030166 ) ) ;
#6345=DIRECTION ( 'NONE',  ( 0.000000000000000000, 0.000000000000000000, -1.000000000000000000 ) ) ;
#6347=CARTESIAN_POINT ( 'NONE',  ( 86.22674662394152278, 0.2046669357502599595, -6.014203425234573963 ) ) ;
#6360=CARTESIAN_POINT ( 'NONE',  ( 35.86856226912744461, -2.087698133915266929, 5.804554645190663997 ) ) ;
#6361=CARTESIAN_POINT ( 'NONE',  ( 87.66750401967712492, -0.1145768689462967616, 4.387407120178886899 ) ) ;
#6362=ORIENTED_EDGE ( 'NONE', *, *, #3882, .T. ) ;
#6364=CARTESIAN_POINT ( 'NONE',  ( 14.70526687707813629, -5.034966368804535186, 2.499999999999956035 ) ) ;
#6365=DIRECTION ( 'NONE',  ( 1.000000000000000000, 8.966158204770716457E-16, 0.000000000000000000 ) ) ;
#6367=CARTESIAN_POINT ( 'NONE',  ( 24.97507460369484278, -5.746002789830511936, -2.897263417418799669 ) ) ;
#6368=ADVANCED_FACE ( 'NONE', ( #7136 ), #1183, .T. ) ;
#6370=CARTESIAN_POINT ( 'NONE',  ( -71.81426791222166628, 3.509262911811426022, 9.960721438266951111 ) ) ;
#6375=AXIS2_PLACEMENT_3D ( 'NONE', #35302, #28904, #9549 ) ;
#6376=CARTESIAN_POINT ( 'NONE',  ( 35.97003858198674209, -3.154676479323113458, 5.820392478026279903 ) ) ;
#6378=CARTESIAN_POINT ( 'NONE',  ( 23.38749234610577687, 2.689796015418254083, 4.224764990934100517 ) ) ;
#6379=CARTESIAN_POINT ( 'NONE',  ( 20.94977919345308948, 9.634852852900486653, -2.522469388968830994 ) ) ;
#6381=EDGE_CURVE ( 'NONE', #19379, #16251, #11612, .T. ) ;
#6384=LINE ( 'NONE', #31497, #19992 ) ;
#6390=CARTESIAN_POINT ( 'NONE',  ( 22.02121393394833149, 4.117315833306967932, -4.097082391610725516 ) ) ;
#6392=CARTESIAN_POINT ( 'NONE',  ( 21.85643539959775694, 0.6980322203039187601, 15.81276153107902616 ) ) ;
#6396=CARTESIAN_POINT ( 'NONE',  ( 85.93841924537714760, 1.827613216861550205, 4.619486236290579306 ) ) ;
#6399=CARTESIAN_POINT ( 'NONE',  ( 14.65885757255257893, 12.91887598177978624, 2.499999999999996891 ) ) ;
#6400=CARTESIAN_POINT ( 'NONE',  ( 28.88870942992270940, -3.138682824899541313, 4.706547700740843609 ) ) ;
#6402=CARTESIAN_POINT ( 'NONE',  ( 37.04571469918683135, -2.801042461011243212, -5.988277751440494789 ) ) ;
#6410=CARTESIAN_POINT ( 'NONE',  ( 35.72972106090838906, -1.305514564919402432, 5.539022487619330803 ) ) ;
#6414=EDGE_CURVE ( 'NONE', #19825, #36582, #14796, .T. ) ;
#6415=VERTEX_POINT ( 'NONE', #14103 ) ;
#6416=CARTESIAN_POINT ( 'NONE',  ( 87.04213330793400871, 0.5878691963681514920, -4.891134986362597914 ) ) ;
#6417=CARTESIAN_POINT ( 'NONE',  ( -80.91065676098010329, -6.597313057213482601, -0.5950503846463383040 ) ) ;
#6419=CARTESIAN_POINT ( 'NONE',  ( -17.27251170661583402, 0.7293679304675921848, -6.000000000000000000 ) ) ;
#6421=DIRECTION ( 'NONE',  ( -0.000000000000000000, -0.000000000000000000, -1.000000000000000000 ) ) ;
#6432=CARTESIAN_POINT ( 'NONE',  ( 16.93405020700152264, 9.102874499958653942, -2.849366104991231996 ) ) ;
#6441=EDGE_CURVE ( 'NONE', #25138, #15211, #28813, .T. ) ;
#6448=CARTESIAN_POINT ( 'NONE',  ( 26.86540377008237357, 1.668949755151340586, -4.708546860826485769 ) ) ;
#6457=CARTESIAN_POINT ( 'NONE',  ( 36.98471844170311584, -3.196209668142826921, -5.957689647507654840 ) ) ;
#6458=PLANE ( 'NONE',  #18725 ) ;
#6475=CARTESIAN_POINT ( 'NONE',  ( 21.84156485433835471, 4.525468657295988351, 4.021517308586185280 ) ) ;
#6476=DIRECTION ( 'NONE',  ( -0.000000000000000000, -0.000000000000000000, -1.000000000000000000 ) ) ;
#6479=CARTESIAN_POINT ( 'NONE',  ( 24.40779208807497369, 3.164677091567920542, 3.266067496624623256 ) ) ;
#6486=CARTESIAN_POINT ( 'NONE',  ( 21.73675671614552485, 0.3116768600389830390, 8.862532426860488144 ) ) ;
#6495=CARTESIAN_POINT ( 'NONE',  ( 22.34899403049013245, 4.475801132629629642, -6.347516269785208998 ) ) ;
#6497=VERTEX_POINT ( 'NONE', #31200 ) ;
#6498=CARTESIAN_POINT ( 'NONE',  ( -73.25168990586664108, 4.982336816971301374, 10.91515532190027571 ) ) ;
#6504=CARTESIAN_POINT ( 'NONE',  ( 33.45777346496446825, -3.169730459255029054, -5.428292747153331099 ) ) ;
#6505=CARTESIAN_POINT ( 'NONE',  ( 25.73534323679438174, 2.638937876048334630, -3.514020203366912121 ) ) ;
#6508=CARTESIAN_POINT ( 'NONE',  ( 22.17103036364695257, 4.944193875442659980, 3.666723515279467271 ) ) ;
#6513=CARTESIAN_POINT ( 'NONE',  ( 22.52933421130244795, 0.9543590913064874393, -6.221134177511584262 ) ) ;
#6517=ORIENTED_EDGE ( 'NONE', *, *, #20967, .F. ) ;
#6519=CARTESIAN_POINT ( 'NONE',  ( 36.24022540957366090, -2.130119347149664222, 5.862561666964295704 ) ) ;
#6520=EDGE_CURVE ( 'NONE', #32354, #12694, #40432, .T. ) ;
#6522=CARTESIAN_POINT ( 'NONE',  ( 86.69339609521894374, -0.1977197225095213562, 5.906572220802119411 ) ) ;
#6523=LINE ( 'NONE', #34134, #19133 ) ;
#6525=CARTESIAN_POINT ( 'NONE',  ( 25.44052111716949582, 2.260287636792247756, 4.091035459148633535 ) ) ;
#6529=( LENGTH_UNIT ( ) NAMED_UNIT ( * ) SI_UNIT ( .MILLI., .METRE. ) );
#6543=CARTESIAN_POINT ( 'NONE',  ( 14.61802081865033820, -4.461849342347350422, 2.500000000000000000 ) ) ;
#6544=CARTESIAN_POINT ( 'NONE',  ( 24.03936073869400403, 3.329292850658597036, -3.281681657426043675 ) ) ;
#6550=CARTESIAN_POINT ( 'NONE',  ( -80.59239215695774305, -6.629469220045966615, -2.601833008578107620 ) ) ;
#6551=DIRECTION ( 'NONE',  ( 1.000000000000000000, 0.000000000000000000, 0.000000000000000000 ) ) ;
#6554=CARTESIAN_POINT ( 'NONE',  ( 86.84125380892929513, -1.134812445414097981, 5.244953511127716794 ) ) ;
#6558=CARTESIAN_POINT ( 'NONE',  ( 22.07282434680287153, 4.440933931123326239, -0.7814465169830903113 ) ) ;
#6563=CARTESIAN_POINT ( 'NONE',  ( 85.76727974192220927, 0.6799405750822806738, 5.934655056445743426 ) ) ;
#6564=VERTEX_POINT ( 'NONE', #15330 ) ;
#6565=CARTESIAN_POINT ( 'NONE',  ( 36.99247513494067618, -2.719144141632455103, 5.979968429836247878 ) ) ;
#6566=CARTESIAN_POINT ( 'NONE',  ( 86.99908277331161344, 0.6362256001576577225, -5.325422653610870860 ) ) ;
#6570=CARTESIAN_POINT ( 'NONE',  ( 29.49009503893727313, 1.222200888372551253, 4.216489851707110326 ) ) ;
#6578=CARTESIAN_POINT ( 'NONE',  ( -72.02865492783033119, 4.746890789902021623, 9.939612967181826519 ) ) ;
#6582=CARTESIAN_POINT ( 'NONE',  ( 22.52364110764304428, 1.987705025956313598, 5.323102857299951474 ) ) ;
#6583=CARTESIAN_POINT ( 'NONE',  ( 37.17836410518969359, -2.593987027605573203, 5.983491823951893274 ) ) ;
#6590=CARTESIAN_POINT ( 'NONE',  ( -72.42837670882107659, -47.11702805680359063, 9.886859966642603581 ) ) ;
#6591=CARTESIAN_POINT ( 'NONE',  ( 86.34446901633954496, 1.371518841831834701, -4.801737237486140231 ) ) ;
#6595=CARTESIAN_POINT ( 'NONE',  ( 24.11329568594008421, 3.020242353435997895, -3.707757905648319419 ) ) ;
#6598=CARTESIAN_POINT ( 'NONE',  ( 21.85643539959774273, -6.795129563591141064, 12.90182208710982259 ) ) ;
#6603=CARTESIAN_POINT ( 'NONE',  ( 85.57721755140556752, 2.175474006149249018, 4.430974418963669059 ) ) ;
#6606=CARTESIAN_POINT ( 'NONE',  ( 18.26218337247781420, -3.004532202463449764, 3.045102850035385611 ) ) ;
#6607=CARTESIAN_POINT ( 'NONE',  ( 34.77297214516959656, -3.162885276882883900, -5.633561309399683914 ) ) ;
#6613=CARTESIAN_POINT ( 'NONE',  ( 28.28279320485486181, -3.656816081275314545, 4.586715715233614432 ) ) ;
#6615=CARTESIAN_POINT ( 'NONE',  ( 34.79219435089648016, -3.832416447686303851, 5.379528067116686074 ) ) ;
#6627=B_SPLINE_CURVE_WITH_KNOTS ( 'NONE', 3,
 ( #21647, #11944, #36875, #11734, #2108, #18124, #30921, #5586, #30718, #30294, #31119, #5997, #15046, #24311 ),
 .UNSPECIFIED., .F., .F.,
 ( 4, 2, 2, 2, 2, 2, 4 ),
 ( 0.004708422389589472963, 0.005296932628068655100, 0.005591187747308264816, 0.005885442866547874533, 0.006179697985787484249, 0.006473953105027094833, 0.007062463343506314266 ),
 .UNSPECIFIED. ) ;
#6636=VERTEX_POINT ( 'NONE', #19848 ) ;
#6638=CARTESIAN_POINT ( 'NONE',  ( 21.73378977745097629, 0.2086431185004669342, 9.125156574515591146 ) ) ;
#6640=CARTESIAN_POINT ( 'NONE',  ( 17.53208774037409867, 9.003388688526223760, -2.875468385787739667 ) ) ;
#6649=CARTESIAN_POINT ( 'NONE',  ( 30.56085893896448269, -1.894852608703655017, -5.974852047816421319 ) ) ;
#6657=CARTESIAN_POINT ( 'NONE',  ( 36.54096646249387703, -2.167736877196097645, -5.903366266952701835 ) ) ;
#6660=CARTESIAN_POINT ( 'NONE',  ( 14.62224959569264371, -5.050472350199410876, -2.488553708487371008 ) ) ;
#6662=CARTESIAN_POINT ( 'NONE',  ( -76.88335714230863971, 9.426892421563488611, 9.554449558844057222 ) ) ;
#6664=CARTESIAN_POINT ( 'NONE',  ( 21.88155215452677282, -13.30971194246768619, -2.500000000000000444 ) ) ;
#6667=CARTESIAN_POINT ( 'NONE',  ( 31.81893016007982666, -2.964826676376706160, 5.172511613851138890 ) ) ;
#6671=AXIS2_PLACEMENT_3D ( 'NONE', #31559, #3382, #24763 ) ;
#6677=CARTESIAN_POINT ( 'NONE',  ( 23.28355779755547772, 3.054638135287742973, 3.997861808092709079 ) ) ;
#6684=CIRCLE ( 'NONE', #21811, 10.00000000000000888 ) ;
#6689=CARTESIAN_POINT ( 'NONE',  ( 23.08452066313556728, 0.3618351664096016718, 5.927938974875374356 ) ) ;
#6696=ORIENTED_EDGE ( 'NONE', *, *, #31062, .T. ) ;
#6697=CARTESIAN_POINT ( 'NONE',  ( 22.79820677575384380, -6.119817767430131283, -4.702819652331462486 ) ) ;
#6699=CARTESIAN_POINT ( 'NONE',  ( -75.59643797491145278, 8.517404848297713826, 8.876789325663764885 ) ) ;
#6700=CARTESIAN_POINT ( 'NONE',  ( 24.74478317148397366, 0.5639450319252965471, -4.778967461423221152 ) ) ;
#6701=VERTEX_POINT ( 'NONE', #26241 ) ;
#6705=CARTESIAN_POINT ( 'NONE',  ( 28.39194851430366029, -3.973459996416360163, -4.268407213906094455 ) ) ;
#6706=CARTESIAN_POINT ( 'NONE',  ( 30.88299797002222746, 0.6986532466800533525, -4.492965408520093185 ) ) ;
#6708=CARTESIAN_POINT ( 'NONE',  ( 16.69500445109213160, 9.542985874932153223, 2.812057233438115755 ) ) ;
#6710=B_SPLINE_CURVE_WITH_KNOTS ( 'NONE', 3,
 ( #16033, #199, #16238, #25107, #31902, #28390 ),
 .UNSPECIFIED., .F., .F.,
 ( 4, 2, 4 ),
 ( 0.000000000000000000, 0.5000000000000001110, 1.000000000000000000 ),
 .UNSPECIFIED. ) ;
#6715=CARTESIAN_POINT ( 'NONE',  ( 33.24375687178804384, -0.2091650819081217472, -4.975944415730187309 ) ) ;
#6720=CARTESIAN_POINT ( 'NONE',  ( -4.224659823956008253, -51.67615071827237472, 6.000000000000000000 ) ) ;
#6721=CARTESIAN_POINT ( 'NONE',  ( 88.27260010123318068, -2.240648412321151639, -1.886171102315310266 ) ) ;
#6722=ADVANCED_FACE ( 'NONE', ( #4422 ), #33605, .T. ) ;
#6725=CARTESIAN_POINT ( 'NONE',  ( 24.53930908985638482, 2.973372590794613135, 3.607145940306804466 ) ) ;
#6739=CARTESIAN_POINT ( 'NONE',  ( -71.92837670882107659, -20.78299143688747819, 9.949874371066202983 ) ) ;
#6740=CARTESIAN_POINT ( 'NONE',  ( 33.78539320900111420, -4.844129098076136231, -3.475568256863553529 ) ) ;
#6741=CARTESIAN_POINT ( 'NONE',  ( 24.72484072709785252, 3.007097173862428363, -3.410376447172846159 ) ) ;
#6747=CARTESIAN_POINT ( 'NONE',  ( -78.65221700006590311, -5.324689618735268581, -8.103210926880651144 ) ) ;
#6748=CIRCLE ( 'NONE', #31730, 8.080217238368755162 ) ;
#6753=CARTESIAN_POINT ( 'NONE',  ( 25.06944232269932016, 3.214832799815183328, -2.439993125860743017 ) ) ;
#6756=FACE_OUTER_BOUND ( 'NONE', #38190, .T. ) ;
#6762=CARTESIAN_POINT ( 'NONE',  ( 34.77305544684841010, -3.164287952476340315, 5.633574310641240146 ) ) ;
#6763=CARTESIAN_POINT ( 'NONE',  ( 86.17935586795600500, 1.556981766839054426, 4.792924669753763744 ) ) ;
#6764=EDGE_CURVE ( 'NONE', #8980, #12694, #1869, .T. ) ;
#6767=CARTESIAN_POINT ( 'NONE',  ( 14.73380738849293792, -5.106256559584044119, 2.499999999999999556 ) ) ;
#6779=CARTESIAN_POINT ( 'NONE',  ( 21.78575280733538122, 1.236091024911973202, 7.097413734593241763 ) ) ;
#6785=CARTESIAN_POINT ( 'NONE',  ( 85.13283666514081460, 2.732481806238816535, 0.06822753118436197806 ) ) ;
#6791=CARTESIAN_POINT ( 'NONE',  ( 22.21123912593981231, 3.886607422916119159, -4.083038617570321271 ) ) ;
#6794=CARTESIAN_POINT ( 'NONE',  ( 21.85643539959772497, -11.05315871940826078, 3.104450560420165317 ) ) ;
#6795=CARTESIAN_POINT ( 'NONE',  ( 21.86697325016263349, 4.291357277889674471, -2.119771864009106999 ) ) ;
#6798=CARTESIAN_POINT ( 'NONE',  ( 86.38515361113813640, 1.239318396469950123, 5.566871328843018496 ) ) ;
#6803=CARTESIAN_POINT ( 'NONE',  ( 17.10999649532181976, -3.067137622865070412, 2.876826778560678033 ) ) ;
#6806=CARTESIAN_POINT ( 'NONE',  ( 20.42490770359840369, 3.667757226666287007, -3.394198844042774166 ) ) ;
#6807=CARTESIAN_POINT ( 'NONE',  ( 4.938390203311415748E-15, -42.37473357531882101, -6.000000000000000000 ) ) ;
#6809=CARTESIAN_POINT ( 'NONE',  ( -72.85689734034554021, 1.996344439234811086, 10.96066712856931602 ) ) ;
#6818=CARTESIAN_POINT ( 'NONE',  ( 33.68493938990636849, -3.838059396421490188, 5.140109112596683794 ) ) ;
#6825=ORIENTED_EDGE ( 'NONE', *, *, #38525, .T. ) ;
#6830=CARTESIAN_POINT ( 'NONE',  ( -80.90861860399088812, 11.45717611192839591, 0.6283086135788885640 ) ) ;
#6835=CARTESIAN_POINT ( 'NONE',  ( 20.81692704467059585, 6.281028057870155834, -3.335911822296410811 ) ) ;
#6844=CARTESIAN_POINT ( 'NONE',  ( 15.80745327116133936, 8.002139867661446360, 3.484773800359248774 ) ) ;
#6845=CARTESIAN_POINT ( 'NONE',  ( 29.34753533916922308, -2.431376398363487734, 5.582488461359439214 ) ) ;
#6849=DIRECTION ( 'NONE',  ( 0.000000000000000000, -0.000000000000000000, -1.000000000000000000 ) ) ;
#6856=CARTESIAN_POINT ( 'NONE',  ( 33.44745999691134131, -3.711946420718001516, -5.220912322284510410 ) ) ;
#6857=CARTESIAN_POINT ( 'NONE',  ( 36.92452998447934931, -2.367281692537941407, -5.951679316537522801 ) ) ;
#6862=CARTESIAN_POINT ( 'NONE',  ( -77.03546220438488490, 9.512508967889075961, 9.454972000433079060 ) ) ;
#6863=CARTESIAN_POINT ( 'NONE',  ( 21.88182916724444382, -13.30283805793968277, -2.499999999999999112 ) ) ;
#6864=CARTESIAN_POINT ( 'NONE',  ( 21.88116416870838066, -13.31970824832912825, 2.499999999999999112 ) ) ;
#6865=CARTESIAN_POINT ( 'NONE',  ( 31.79659951825298947, -2.963653280094607823, 5.169026377125449656 ) ) ;
#6867=EDGE_LOOP ( 'NONE', ( #10647, #31968 ) ) ;
#6868=CARTESIAN_POINT ( 'NONE',  ( -12.99139449055068241, -10.90558813203967148, 6.000000000000000000 ) ) ;
#6873=CARTESIAN_POINT ( 'NONE',  ( 21.84694118651422201, 4.320250114505405747, 4.147421643609518149 ) ) ;
#6877=CARTESIAN_POINT ( 'NONE',  ( 22.38249921582006507, 4.935340343470858926, 3.052593005165685991 ) ) ;
#6885=CARTESIAN_POINT ( 'NONE',  ( 27.41509945826695471, 1.020312500805418132, 4.485089514595300919 ) ) ;
#6889=ADVANCED_FACE ( 'NONE', ( #2349, #9107 ), #27440, .F. ) ;
#6895=CARTESIAN_POINT ( 'NONE',  ( -73.50257855008051422, -0.7799437568714130409, 9.721213065138739395 ) ) ;
#6897=ADVANCED_FACE ( 'NONE', ( #28047 ), #21684, .F. ) ;
#6902=CARTESIAN_POINT ( 'NONE',  ( 32.00493796099151922, -3.634882110226827390, -4.956983323664922558 ) ) ;
#6903=CARTESIAN_POINT ( 'NONE',  ( 33.94631716816222422, -0.4876237784438076095, -5.120956352787560562 ) ) ;
#6905=CARTESIAN_POINT ( 'NONE',  ( 16.86343556102044872, 9.686623936461598916, 2.782464905949770362 ) ) ;
#6909=VECTOR ( 'NONE', #18088, 1000.000000000000114 ) ;
#6910=DIRECTION ( 'NONE',  ( 1.000000000000000000, -1.061555284671232059E-15, 0.000000000000000000 ) ) ;
#6911=CARTESIAN_POINT ( 'NONE',  ( 29.63503081302897968, 1.162161518828512152, -4.256401061717856926 ) ) ;
#6916=CARTESIAN_POINT ( 'NONE',  ( 88.80100535589549793, -2.068446212231642711, -0.8863989573356614304 ) ) ;
#6918=CARTESIAN_POINT ( 'NONE',  ( 26.58413863979593827, 1.645201016816646877, 4.327475460437605115 ) ) ;
#6919=CARTESIAN_POINT ( 'NONE',  ( -4.266520354791871306, -48.67644278316300444, 6.000000000000000000 ) ) ;
#6935=CARTESIAN_POINT ( 'NONE',  ( 21.85643539959775339, -7.728916438363212293, -14.50668795789714771 ) ) ;
#6936=CARTESIAN_POINT ( 'NONE',  ( 24.74506495819852248, 3.013726380158780582, -3.376567986019525680 ) ) ;
#6942=CARTESIAN_POINT ( 'NONE',  ( -18.27651686900387418, -64.04014080848075707, -2.500000000000000000 ) ) ;
#6944=CARTESIAN_POINT ( 'NONE',  ( -73.25156588610681752, -0.1223437846077502639, -10.91517253786405028 ) ) ;
#6948=CARTESIAN_POINT ( 'NONE',  ( 84.14932678670007249, 2.958124188176427083, -1.306863746360770184 ) ) ;
#6950=CARTESIAN_POINT ( 'NONE',  ( -17.69482985384422236, -39.37473357531881391, 6.000000000000000000 ) ) ;
#6951=CARTESIAN_POINT ( 'NONE',  ( 23.06591706423118637, -8.086835649431872497, -2.500000000000005773 ) ) ;
#6952=CARTESIAN_POINT ( 'NONE',  ( 34.81584145744843539, -1.659602413401581211, 5.640252102379137433 ) ) ;
#6954=CIRCLE ( 'NONE', #39834, 10.00000000000000888 ) ;
#6956=DIRECTION ( 'NONE',  ( 0.000000000000000000, -0.000000000000000000, -1.000000000000000000 ) ) ;
#6960=CARTESIAN_POINT ( 'NONE',  ( 33.68706075914577269, -3.105129560293249380, 5.464078574745403927 ) ) ;
#6963=CARTESIAN_POINT ( 'NONE',  ( 86.81546468666313388, 0.8424741501213859340, -5.177899619954967392 ) ) ;
#6968=CARTESIAN_POINT ( 'NONE',  ( -69.93649553638499583, -48.24651348640838222, 9.950929893704707041 ) ) ;
#6973=CARTESIAN_POINT ( 'NONE',  ( -72.13633209003711499, 5.157242105139857813, 9.927673127863286595 ) ) ;
#6974=ORIENTED_EDGE ( 'NONE', *, *, #40112, .T. ) ;
#6977=CARTESIAN_POINT ( 'NONE',  ( 22.83085956305526310, 1.197354866361570513, 5.675763816237461512 ) ) ;
#6982=CARTESIAN_POINT ( 'NONE',  ( 14.77222812468899349, 12.33286846116284252, -2.511961485181726239 ) ) ;
#6987=CARTESIAN_POINT ( 'NONE',  ( 23.01932435154908418, 3.404353093427882726, -3.868829002755526325 ) ) ;
#6991=CARTESIAN_POINT ( 'NONE',  ( 21.85643539959777470, 7.942361823516107755, 9.319573164223585948 ) ) ;
#6992=CARTESIAN_POINT ( 'NONE',  ( 21.76122352783369251, 6.560793838969577685, -3.350653129111269113 ) ) ;
#6997=CARTESIAN_POINT ( 'NONE',  ( 87.54376689718995408, -0.1385995495200708916, -5.388168202639758597 ) ) ;
#7000=CARTESIAN_POINT ( 'NONE',  ( 33.11529288468890542, -3.093421031358547513, 5.374840369677361451 ) ) ;
#7002=CARTESIAN_POINT ( 'NONE',  ( 35.86909678445674388, -2.086596214755629397, -5.804638069235120490 ) ) ;
#7004=CARTESIAN_POINT ( 'NONE',  ( 85.57577930415899914, 1.015208198401525541, 5.782835925834406865 ) ) ;
#7005=CARTESIAN_POINT ( 'NONE',  ( -75.55726679169593751, -3.620980792413103000, 10.26686770233818535 ) ) ;
#7010=ORIENTED_EDGE ( 'NONE', *, *, #9148, .T. ) ;
#7011=CARTESIAN_POINT ( 'NONE',  ( 36.44367144241243039, -1.735187743863684684, 5.732522741015722012 ) ) ;
#7018=CYLINDRICAL_SURFACE ( 'NONE', #20031, 10.00000000000000533 ) ;
#7024=ADVANCED_FACE ( 'NONE', ( #16303 ), #14405, .F. ) ;
#7040=CARTESIAN_POINT ( 'NONE',  ( 31.90185279284946773, -4.312872639525808793, -3.838359570106229413 ) ) ;
#7043=CARTESIAN_POINT ( 'NONE',  ( 21.85643539959777115, -11.26372485911396737, 0.7475790860009233763 ) ) ;
#7048=CARTESIAN_POINT ( 'NONE',  ( 36.82690608461941650, -3.168782876732829656, -5.951696020828944889 ) ) ;
#7050=CARTESIAN_POINT ( 'NONE',  ( 14.77222812468949442, 12.59898556833855032, -2.511961485181804843 ) ) ;
#7054=CARTESIAN_POINT ( 'NONE',  ( -12.99139449055068241, -10.90558813203967148, 6.000000000000000000 ) ) ;
#7055=EDGE_CURVE ( 'NONE', #21186, #1813, #24243, .T. ) ;
#7056=CARTESIAN_POINT ( 'NONE',  ( 22.03291717603176636, -11.53685166237917947, 2.500000000000000000 ) ) ;
#7063=CARTESIAN_POINT ( 'NONE',  ( 30.57637419526079725, -3.206146428843060114, 4.965636198024955483 ) ) ;
#7064=CARTESIAN_POINT ( 'NONE',  ( 22.19267663920264511, 4.186142737966082272, 3.887493867850188689 ) ) ;
#7067=VERTEX_POINT ( 'NONE', #13391 ) ;
#7068=EDGE_CURVE ( 'NONE', #24796, #34269, #1230, .T. ) ;
#7070=CIRCLE ( 'NONE', #12321, 6.000000000000002665 ) ;
#7074=LINE ( 'NONE', #4599, #28049 ) ;
#7079=CARTESIAN_POINT ( 'NONE',  ( 26.03581818370150103, 0.8240965440397407527, 4.423294059681629697 ) ) ;
#7090=CARTESIAN_POINT ( 'NONE',  ( 24.83717141299267794, -2.182840666565796006, 6.391756413845674167 ) ) ;
#7093=CARTESIAN_POINT ( 'NONE',  ( -80.16996465541035377, -5.617423336303677850, 6.125224573262133099 ) ) ;
#7094=CARTESIAN_POINT ( 'NONE',  ( 26.06744311131525649, 0.7515804080732310100, -4.421654772982752668 ) ) ;
#7095=CARTESIAN_POINT ( 'NONE',  ( -70.92837670882107659, 13.87661300689599742, -10.00000000000000533 ) ) ;
#7099=CARTESIAN_POINT ( 'NONE',  ( 34.79206662659809979, -3.832422124991777146, -5.379499388740839549 ) ) ;
#7100=CARTESIAN_POINT ( 'NONE',  ( 30.31649042712836817, -3.037113472960369265, -4.938316272775912452 ) ) ;
#7102=CARTESIAN_POINT ( 'NONE',  ( 15.70676156960853298, 10.60592294505261357, 2.657818031038195805 ) ) ;
#7105=PLANE ( 'NONE',  #29589 ) ;
#7109=CARTESIAN_POINT ( 'NONE',  ( 23.18429543757034139, 0.8410905956396856897, -5.610387443514746053 ) ) ;
#7110=CARTESIAN_POINT ( 'NONE',  ( 33.93434842054367095, -0.4888659768199489219, -5.123735918607922990 ) ) ;
#7112=ORIENTED_EDGE ( 'NONE', *, *, #40454, .F. ) ;
#7115=CARTESIAN_POINT ( 'NONE',  ( 86.69422455818764206, -0.1941184515037400471, -5.886102099071623073 ) ) ;
#7118=ORIENTED_EDGE ( 'NONE', *, *, #18334, .T. ) ;
#7119=CARTESIAN_POINT ( 'NONE',  ( -81.78216522710987135, 10.46482146603914209, -1.037938286043770253 ) ) ;
#7123=LINE ( 'NONE', #35350, #39777 ) ;
#7133=CARTESIAN_POINT ( 'NONE',  ( 24.24184507690288015, 2.646254481897600819, 3.989924234126151159 ) ) ;
#7135=CARTESIAN_POINT ( 'NONE',  ( 27.52856511457626709, -4.375065239674293949, 3.731061453272236150 ) ) ;
#7136=FACE_OUTER_BOUND ( 'NONE', #27715, .T. ) ;
#7137=CARTESIAN_POINT ( 'NONE',  ( 21.85643539959774273, -11.65679437655345474, 11.20963770477306554 ) ) ;
#7138=CARTESIAN_POINT ( 'NONE',  ( 23.14098296504576524, 4.020346899343795855, -3.126915550736968363 ) ) ;
#7143=CARTESIAN_POINT ( 'NONE',  ( -71.75682404118637692, 2.644744199176562560, -9.965669106298006952 ) ) ;
#7148=CARTESIAN_POINT ( 'NONE',  ( 86.43572624768424362, -0.5192074800720991590, -5.777013305174518720 ) ) ;
#7152=ORIENTED_EDGE ( 'NONE', *, *, #7837, .T. ) ;
#7156=DIRECTION ( 'NONE',  ( -0.000000000000000000, -0.000000000000000000, -1.000000000000000000 ) ) ;
#7157=ORIENTED_EDGE ( 'NONE', *, *, #36678, .F. ) ;
#7159=CARTESIAN_POINT ( 'NONE',  ( 36.91107007784989236, -2.639074378160587209, 5.967263201888431290 ) ) ;
#7160=ADVANCED_FACE ( 'NONE', ( #3284 ), #12855, .F. ) ;
#7162=CARTESIAN_POINT ( 'NONE',  ( 85.88453125851971492, 1.888142761377891832, -4.329341218647970280 ) ) ;
#7168=ORIENTED_EDGE ( 'NONE', *, *, #5758, .F. ) ;
#7171=CARTESIAN_POINT ( 'NONE',  ( -77.60377033239008426, -6.254646173284871935, 7.448572753700554827 ) ) ;
#7173=ORIENTED_EDGE ( 'NONE', *, *, #8684, .F. ) ;
#7178=CARTESIAN_POINT ( 'NONE',  ( 25.03740577281743285, 1.729533793843111678, 4.338254701037809191 ) ) ;
#7185=CARTESIAN_POINT ( 'NONE',  ( 23.67583169985504910, 3.109125002522015624, -3.791247457039441660 ) ) ;
#7190=CARTESIAN_POINT ( 'NONE',  ( 21.85643539959776760, 6.468309080218945795, -8.875946301973074881 ) ) ;
#7191=CARTESIAN_POINT ( 'NONE',  ( 21.89426278105499435, 4.196054223286251883, 2.573115994139398661E-12 ) ) ;
#7195=CARTESIAN_POINT ( 'NONE',  ( 88.02721697999687933, -0.6980542412123691420, -4.669518943469966210 ) ) ;
#7201=CARTESIAN_POINT ( 'NONE',  ( 30.51645556077223631, -0.1367088690802835960, -4.969228952161986790 ) ) ;
#7208=CARTESIAN_POINT ( 'NONE',  ( 28.62762293107049416, -3.097373597580966642, 4.674430938707033967 ) ) ;
#7211=CARTESIAN_POINT ( 'NONE',  ( 33.94565407617458419, -0.4887086158907474887, 5.122328562820444908 ) ) ;
#7214=CARTESIAN_POINT ( 'NONE',  ( 87.70554304502432785, -2.246019397594158473, 2.665219128644956914 ) ) ;
#7221=DIRECTION ( 'NONE',  ( -0.000000000000000000, -1.000000000000000000, -0.000000000000000000 ) ) ;
#7228=CYLINDRICAL_SURFACE ( 'NONE', #35135, 2.500000000000000444 ) ;
#7238=CARTESIAN_POINT ( 'NONE',  ( 23.52943196063522535, 3.064722609491274952, -3.878734937556255868 ) ) ;
#7242=CARTESIAN_POINT ( 'NONE',  ( 30.13572739226143327, -4.670734905539763560, 0.4584422186006349986 ) ) ;
#7248=CARTESIAN_POINT ( 'NONE',  ( 20.76538241992246014, 4.421523770943674769, -3.217089656416562082 ) ) ;
#7257=CARTESIAN_POINT ( 'NONE',  ( 36.68208917225820187, -3.313352327499882843, 5.912027108166803657 ) ) ;
#7263=CARTESIAN_POINT ( 'NONE',  ( 30.89397235467784597, -3.431564488292946358, 4.935950646977611989 ) ) ;
#7265=CARTESIAN_POINT ( 'NONE',  ( 22.60554062051026136, 3.598027713168910235, 3.981257213926762795 ) ) ;
#7271=CARTESIAN_POINT ( 'NONE',  ( 24.06785808357873080, 3.349623670569857659, 3.203142401354519553 ) ) ;
#7275=FACE_OUTER_BOUND ( 'NONE', #10490, .T. ) ;
#7278=CARTESIAN_POINT ( 'NONE',  ( 22.29898859944773903, 0.2633200660602942333, 7.098944222140404214 ) ) ;
#7279=CARTESIAN_POINT ( 'NONE',  ( 14.69274635589773581, -4.522481898537247247, -2.499999999999558575 ) ) ;
#7286=CARTESIAN_POINT ( 'NONE',  ( 22.33594428049882197, 5.124660873843202680, 5.347558210918236909 ) ) ;
#7287=EDGE_CURVE ( 'NONE', #9413, #8630, #36911, .T. ) ;
#7290=CARTESIAN_POINT ( 'NONE',  ( -79.27250537723340074, -5.532529408078902478, 5.525611224659603415 ) ) ;
#7291=CARTESIAN_POINT ( 'NONE',  ( 22.28290334446566945, 0.2420565227163372635, -7.135904416810470607 ) ) ;
#7296=CARTESIAN_POINT ( 'NONE',  ( 36.71877240845051205, -3.457495992918012906, -5.861073688215565625 ) ) ;
#7297=CARTESIAN_POINT ( 'NONE',  ( 30.43983800511932358, -3.117243395012541995, -4.952810734695171746 ) ) ;
#7300=PLANE ( 'NONE',  #17299 ) ;
#7306=CARTESIAN_POINT ( 'NONE',  ( 24.08611371057580186, 0.7123248832134593256, -5.071621260587827251 ) ) ;
#7310=ORIENTED_EDGE ( 'NONE', *, *, #24184, .T. ) ;
#7312=CARTESIAN_POINT ( 'NONE',  ( 85.62750488955801131, 0.9367966501063212936, -5.850367371124844063 ) ) ;
#7315=CARTESIAN_POINT ( 'NONE',  ( -75.87812283331165020, 8.749605185975593002, -10.12194526897379099 ) ) ;
#7320=DIRECTION ( 'NONE',  ( -0.000000000000000000, -1.000000000000000000, -0.000000000000000000 ) ) ;
#7324=CARTESIAN_POINT ( 'NONE',  ( 33.87523647309109265, -5.320081038359204761, 1.808392000078312467 ) ) ;
#7332=DIRECTION ( 'NONE',  ( -0.000000000000000000, -1.000000000000000000, -0.000000000000000000 ) ) ;
#7334=CARTESIAN_POINT ( 'NONE',  ( 22.18599700961289756, 5.272392256036439129, -3.073166440102835573 ) ) ;
#7336=CARTESIAN_POINT ( 'NONE',  ( 14.75467646479344097, -5.149013399961007487, -2.500000000000000000 ) ) ;
#7337=LINE ( 'NONE', #6942, #33326 ) ;
#7338=AXIS2_PLACEMENT_3D ( 'NONE', #2088, #14600, #27172 ) ;
#7339=CARTESIAN_POINT ( 'NONE',  ( -73.13193655429402895, 4.589176838546805470, -10.93047759564017696 ) ) ;
#7341=DIRECTION ( 'NONE',  ( 1.000000000000000000, -1.061555284671232059E-15, 0.000000000000000000 ) ) ;
#7344=CARTESIAN_POINT ( 'NONE',  ( 21.58874331597417040, 7.202613857503122219, -2.924296597703472500 ) ) ;
#7348=EDGE_CURVE ( 'NONE', #30583, #35921, #38973, .T. ) ;
#7351=CARTESIAN_POINT ( 'NONE',  ( 14.77222812468899349, 12.33286846116284252, -2.511961485181726239 ) ) ;
#7356=CARTESIAN_POINT ( 'NONE',  ( 34.33282722039242429, -1.486069782136362205, 5.564866048942920251 ) ) ;
#7359=CARTESIAN_POINT ( 'NONE',  ( 86.12362567153361681, 1.619580568575353485, 4.895344567657775592 ) ) ;
#7363=CARTESIAN_POINT ( 'NONE',  ( 87.73735837800707316, -0.1930405997103058768, -3.830955553240402711 ) ) ;
#7368=ORIENTED_EDGE ( 'NONE', *, *, #15054, .F. ) ;
#7370=DIRECTION ( 'NONE',  ( -0.000000000000000000, -0.000000000000000000, -1.000000000000000000 ) ) ;
#7372=CARTESIAN_POINT ( 'NONE',  ( 23.45630354681979313, 1.541145148875956883, 5.001686380149122257 ) ) ;
#7376=CARTESIAN_POINT ( 'NONE',  ( 14.73750015949766023, 12.90700633730901359, -2.501527175807457759 ) ) ;
#7377=CARTESIAN_POINT ( 'NONE',  ( 85.15174684586190779, 2.711240993721571790, -0.5174129942806917626 ) ) ;
#7381=ORIENTED_EDGE ( 'NONE', *, *, #16004, .F. ) ;
#7382=CARTESIAN_POINT ( 'NONE',  ( 23.17191900141983041, 3.801330203260075091, -3.394942160406552834 ) ) ;
#7387=CARTESIAN_POINT ( 'NONE',  ( 21.85643539959776049, -13.25144142801168634, -1.676981927294508345 ) ) ;
#7389=CARTESIAN_POINT ( 'NONE',  ( 21.80882946373430542, 5.293150380057753956, 3.367598806148119905 ) ) ;
#7393=CARTESIAN_POINT ( 'NONE',  ( 88.18839210903504977, -0.8832026502337909646, 4.329116466421397469 ) ) ;
#7397=CARTESIAN_POINT ( 'NONE',  ( -81.15124214773400979, -5.648850483656841170, 4.015016724928055503 ) ) ;
#7398=CARTESIAN_POINT ( 'NONE',  ( 14.59363405247780321, -5.046850784924433064, 2.484087560899213010 ) ) ;
#7399=CARTESIAN_POINT ( 'NONE',  ( 31.28009924878942627, -3.760136573936985194, 4.659093935210213644 ) ) ;
#7400=CARTESIAN_POINT ( 'NONE',  ( 17.00076660167203357, -3.039841025278140041, -2.859778811921668940 ) ) ;
#7401=CARTESIAN_POINT ( 'NONE',  ( 20.42384695622214963, 3.665139109075679524, -3.394033288760437639 ) ) ;
#7403=CARTESIAN_POINT ( 'NONE',  ( 85.08263568025058987, 1.762786880713592463, 5.091211749826051403 ) ) ;
#7410=CARTESIAN_POINT ( 'NONE',  ( 34.63713585988073618, -0.7818613632861374230, 5.275101436747132055 ) ) ;
#7413=CARTESIAN_POINT ( 'NONE',  ( 86.30560996193628398, -0.3002381051633802866, 5.887336558433836409 ) ) ;
#7414=ORIENTED_EDGE ( 'NONE', *, *, #7837, .F. ) ;
#7420=CARTESIAN_POINT ( 'NONE',  ( 22.73433657433409749, 4.113458136755731687, 3.466401380080733396 ) ) ;
#7422=B_SPLINE_CURVE_WITH_KNOTS ( 'NONE', 3,
 ( #4574, #11882, #29672, #17493, #27747, #2872, #40494, #26590, #5732, #17296, #29874, #1484, #14018, #14989 ),
 .UNSPECIFIED., .F., .F.,
 ( 4, 2, 2, 2, 2, 2, 4 ),
 ( 0.000000000000000000, 0.0002935890969200457981, 0.0005871781938400915963, 0.0008807672907601373944, 0.001174356387680183193, 0.001761534581520288884, 0.002348712775360395008 ),
 .UNSPECIFIED. ) ;
#7428=CARTESIAN_POINT ( 'NONE',  ( 21.28603936774592498, 5.337095168022400138, -3.528599266780989563 ) ) ;
#7438=CARTESIAN_POINT ( 'NONE',  ( 32.02627343617642453, -1.895034194620857315, -5.999511542327915947 ) ) ;
#7443=CARTESIAN_POINT ( 'NONE',  ( -75.12839812606507905, -3.199487166374271663, -10.43546860170108026 ) ) ;
#7448=EDGE_CURVE ( 'NONE', #11412, #34747, #17551, .T. ) ;
#7449=CARTESIAN_POINT ( 'NONE',  ( 30.74497410374950945, 0.4681497935174912528, -4.860627807659219535 ) ) ;
#7457=CARTESIAN_POINT ( 'NONE',  ( -4.444218661349752963, -35.94265729135299381, 6.000000000000000000 ) ) ;
#7459=CARTESIAN_POINT ( 'NONE',  ( 36.58893514583110118, -2.079415496222606574, 5.884068123001751083 ) ) ;
#7465=CARTESIAN_POINT ( 'NONE',  ( 30.79039095446131213, -3.336666825807130810, 4.961975926287203187 ) ) ;
#7466=CARTESIAN_POINT ( 'NONE',  ( 85.00501152238103941, 1.866990000816762585, -4.914164337049770737 ) ) ;
#7471=CARTESIAN_POINT ( 'NONE',  ( 21.83074723418732432, 5.960639454754549149, 3.136932506330722514 ) ) ;
#7480=CARTESIAN_POINT ( 'NONE',  ( 22.62344975043419026, 0.2992865745580874370, 6.483493247686526573 ) ) ;
#7484=B_SPLINE_CURVE_WITH_KNOTS ( 'NONE', 3,
 ( #18490, #3502, #28592, #13651 ),
 .UNSPECIFIED., .F., .F.,
 ( 4, 4 ),
 ( 0.6621368017907995895, 0.8210829304512126114 ),
 .UNSPECIFIED. ) ;
#7489=CARTESIAN_POINT ( 'NONE',  ( 22.42980438978510449, 1.271109115893125585, 8.904229291692644210 ) ) ;
#7492=CARTESIAN_POINT ( 'NONE',  ( -76.49288603080218252, -4.334318986430696796, 9.797079263697156648 ) ) ;
#7493=CARTESIAN_POINT ( 'NONE',  ( 24.12420224480490916, 0.5001390095518741807, -5.094071010228495844 ) ) ;
#7496=CARTESIAN_POINT ( 'NONE',  ( 37.18637049283714191, -2.963493602741866351, -6.000003475307118528 ) ) ;
#7497=DIRECTION ( 'NONE',  ( -0.000000000000000000, 0.000000000000000000, 1.000000000000000000 ) ) ;
#7511=CARTESIAN_POINT ( 'NONE',  ( 88.16134551068515179, -2.448791080374484341, 0.2153404935567143075 ) ) ;
#7514=CARTESIAN_POINT ( 'NONE',  ( -81.79890681550139675, 10.46299657128043314, 0.6911394749367771873 ) ) ;
#7523=CARTESIAN_POINT ( 'NONE',  ( 37.14386006597155898, -2.493502119373617099, 5.967606418918435907 ) ) ;
#7532=CARTESIAN_POINT ( 'NONE',  ( -70.92837670882107659, -37.87473357531881391, 0.000000000000000000 ) ) ;
#7533=CARTESIAN_POINT ( 'NONE',  ( 21.71190961143752673, 6.329471954421165059, -3.192818159646633625 ) ) ;
#7539=CARTESIAN_POINT ( 'NONE',  ( -74.65853108593573495, -2.675584617184129765, -9.325032285645074026 ) ) ;
#7554=CARTESIAN_POINT ( 'NONE',  ( 37.04382469011167700, -2.892849699906013150, 5.987982769814347073 ) ) ;
#7556=AXIS2_PLACEMENT_3D ( 'NONE', #11274, #39288, #4720 ) ;
#7558=CARTESIAN_POINT ( 'NONE',  ( 84.79389884800966115, 3.063713526918731223, 0.3112276665278714827 ) ) ;
#7561=VECTOR ( 'NONE', #16166, 1000.000000000000000 ) ;
#7564=CARTESIAN_POINT ( 'NONE',  ( -80.67007510693973416, 11.48218648236320050, -2.296920554925718339 ) ) ;
#7565=CARTESIAN_POINT ( 'NONE',  ( 21.78047190118184773, 5.616103730238553027, 3.473245441588607374 ) ) ;
#7573=CARTESIAN_POINT ( 'NONE',  ( 25.01091298175105848, 3.329590532566609529, -1.936828115965013142 ) ) ;
#7576=CARTESIAN_POINT ( 'NONE',  ( 21.77340129706707472, 1.030455091318688288, 7.426159514375072490 ) ) ;
#7578=ADVANCED_FACE ( 'NONE', ( #24565 ), #40608, .F. ) ;
#7580=CARTESIAN_POINT ( 'NONE',  ( 39.57450465021913999, -13.08403409140692553, 6.000000000000001776 ) ) ;
#7582=B_SPLINE_SURFACE_WITH_KNOTS ( 'NONE', 5, 3, ( 
 ( #25392, #1248, #13975, #26353, #38885, #12818, #14177, #29825, #10678, #7400, #23453, #19212, #26544, #10481, #16854, #4530, #15914 ),
 ( #36021, #4334, #32340, #23259, #13578, #35826, #28473, #26747, #32929, #17252, #4133, #20351, #9524, #22108, #7601, #17052, #7798 ),
 ( #1044, #4718, #1638, #32735, #34685, #19012, #29629, #31573, #1443, #19953, #39082, #37931, #280, #6660, #16648, #29236, #26151 ),
 ( #38684, #23061, #24043, #40106, #8183, #14992, #39690, #5325, #33746, #33131, #36411, #11886, #33550, #20755, #39903, #2052, #14774 ),
 ( #15192, #21384, #5734, #33346, #8800, #39286, #11074, #30441, #5525, #24459, #30237, #14565, #37017, #18274, #20969, #17860, #27139 ),
 ( #30866, #5122, #33960, #14371, #23644, #4913, #2251, #27550, #36211, #17655, #27345, #17444, #7990, #18069, #8600, #2673, #20547 ),
 ( #11677, #24254, #30034, #36817, #1849, #26941, #39483, #11272, #23835, #11478, #36612, #8396, #21178, #30658, #2468, #37221, #12308 ),
 ( #9012, #12928, #28159, #5940, #9217, #18478, #19309, #31065, #21591, #25293, #6145, #34785, #27750, #21796, #37828, #27954, #2875 ) ),
 .UNSPECIFIED., .F., .F., .F.,
 ( 6, 2, 6 ),
 ( 4, 1, 1, 1, 1, 1, 1, 1, 1, 1, 1, 1, 1, 1, 4 ),
 ( 0.000000000000000000, 0.5000000000000000000, 1.000000000000000000 ),
 ( 0.006307410990057117292, 0.008855845011544563258, 0.01161705605602081880, 0.01384754710661961243, 0.01682153517408467233, 0.01905202622468346596, 0.02091076876684912558, 0.02239776280058165467, 0.02351300832588105669, 0.02462825385118044830, 0.02555762512226328331, 0.02630112213912954092, 0.02685874490177924193, 0.02741636766442894294, 0.02797399042707864047 ),
 .UNSPECIFIED. ) ;
#7584=CARTESIAN_POINT ( 'NONE',  ( 21.79149120270722406, 5.488331395040956018, -3.526327173381369917 ) ) ;
#7588=CARTESIAN_POINT ( 'NONE',  ( 22.68001568621454567, -4.050230952900990111, -7.789969220879865652 ) ) ;
#7590=CARTESIAN_POINT ( 'NONE',  ( 20.24823138111565868, 11.68787526792871567, -3.842642712661572979 ) ) ;
#7591=CARTESIAN_POINT ( 'NONE',  ( 18.62546845537173823, 11.49410710365845034, 2.500000000000000444 ) ) ;
#7596=CARTESIAN_POINT ( 'NONE',  ( 88.31640312351544253, -1.506181138579067103, 3.771763452802144201 ) ) ;
#7599=CARTESIAN_POINT ( 'NONE',  ( 26.28491678605064052, -2.762637008470093303, 4.308794986214664391 ) ) ;
#7601=CARTESIAN_POINT ( 'NONE',  ( 14.65806710266428858, -5.610108328300923652, -2.494143896700089957 ) ) ;
#7602=CARTESIAN_POINT ( 'NONE',  ( 35.33510954239903867, -3.168965055208807780, -5.721296445581753431 ) ) ;
#7604=CARTESIAN_POINT ( 'NONE',  ( 84.10606912909534572, 3.010615857166643927, -0.2786395050580429689 ) ) ;
#7605=CARTESIAN_POINT ( 'NONE',  ( 30.38040035538539385, -3.658749391580585986, -4.669445293200252145 ) ) ;
#7611=CARTESIAN_POINT ( 'NONE',  ( 36.88815924642239708, -3.351591737224890899, 5.910525939546068308 ) ) ;
#7612=B_SPLINE_CURVE_WITH_KNOTS ( 'NONE', 3,
 ( #4878, #30407, #21349, #27309, #11644, #36782, #8565, #9384, #25456, #28129 ),
 .UNSPECIFIED., .F., .F.,
 ( 4, 2, 2, 2, 4 ),
 ( 0.000000000000000000, 0.0003915841590506205440, 0.0007831683181012410880, 0.001174752477151861686, 0.001566336636202482176 ),
 .UNSPECIFIED. ) ;
#7616=CARTESIAN_POINT ( 'NONE',  ( 87.93119157070556469, -2.517311565827366593, -0.4176833736063458868 ) ) ;
#7626=CARTESIAN_POINT ( 'NONE',  ( 21.96632414918468257, 4.998869592191663713, 3.577591828290626275 ) ) ;
#7636=CARTESIAN_POINT ( 'NONE',  ( 23.74466947080636103, 2.426168263719876261, -4.268781924364951408 ) ) ;
#7641=CARTESIAN_POINT ( 'NONE',  ( -9.796229648729232409, -33.54387950140292673, 2.500000000000000000 ) ) ;
#7643=CARTESIAN_POINT ( 'NONE',  ( 8.290806648384990041, -10.90558813203967148, 6.000000000000000000 ) ) ;
#7645=CARTESIAN_POINT ( 'NONE',  ( 87.04213330793400871, 0.5878691963681530464, -4.891134986362597914 ) ) ;
#7646=CARTESIAN_POINT ( 'NONE',  ( 31.36201648005763332, -1.233860125724708379, -5.969386505766030915 ) ) ;
#7653=CARTESIAN_POINT ( 'NONE',  ( 33.65804166975612333, -1.144990435965010711, -5.459549444016131403 ) ) ;
#7657=AXIS2_PLACEMENT_3D ( 'NONE', #8432, #30484, #39121 ) ;
#7661=ORIENTED_EDGE ( 'NONE', *, *, #34680, .F. ) ;
#7662=CARTESIAN_POINT ( 'NONE',  ( 34.12202789009461412, -3.607432811949276896, 5.453396193817899196 ) ) ;
#7668=CARTESIAN_POINT ( 'NONE',  ( 86.43572624768425783, -0.5192074800720990480, -5.777013305174518720 ) ) ;
#7674=CARTESIAN_POINT ( 'NONE',  ( 24.39331214698706063, 3.157612729095597093, 3.298590225890907668 ) ) ;
#7676=CARTESIAN_POINT ( 'NONE',  ( -70.92837670882107659, -47.11702805680359063, 38.00000000000000711 ) ) ;
#7680=CARTESIAN_POINT ( 'NONE',  ( 15.71855938504309158, -1.673920629206014921, -2.500000000000009770 ) ) ;
#7684=CARTESIAN_POINT ( 'NONE',  ( 24.12554661758536412, 0.5101533851207924464, 5.092830807977074770 ) ) ;
#7693=CARTESIAN_POINT ( 'NONE',  ( 27.90799128822289177, 2.452171383980988661, -2.014541967423249424 ) ) ;
#7696=CARTESIAN_POINT ( 'NONE',  ( -77.66794378176071234, -6.280236162145751422, 7.398505571724361296 ) ) ;
#7697=CARTESIAN_POINT ( 'NONE',  ( 23.58963810436863184, 0.4214879312981080761, -5.525765152133263136 ) ) ;
#7701=CARTESIAN_POINT ( 'NONE',  ( 36.20057779688249866, -3.648500508209620907, -5.719125637313637434 ) ) ;
#7707=CARTESIAN_POINT ( 'NONE',  ( 21.56351936394880653, 7.350594945348953857, 2.885250585115055166 ) ) ;
#7710=( GEOMETRIC_REPRESENTATION_CONTEXT ( 3 ) GLOBAL_UNCERTAINTY_ASSIGNED_CONTEXT ( ( #34143 ) ) GLOBAL_UNIT_ASSIGNED_CONTEXT ( ( #37895, #37681, #35048 ) ) REPRESENTATION_CONTEXT ( 'NONE', 'WORKASPACE' ) );
#7712=AXIS2_PLACEMENT_3D ( 'NONE', #24148, #37114, #17961 ) ;
#7715=CARTESIAN_POINT ( 'NONE',  ( 87.52985346608603834, -1.683278932971326691, -4.201117388013917875 ) ) ;
#7716=CARTESIAN_POINT ( 'NONE',  ( 23.06591706423118637, -8.086835649431872497, -2.500000000000005773 ) ) ;
#7718=LINE ( 'NONE', #26066, #20840 ) ;
#7728=CARTESIAN_POINT ( 'NONE',  ( 33.79019614278077199, -4.865436059503933208, 3.423093293932546022 ) ) ;
#7735=CARTESIAN_POINT ( 'NONE',  ( 21.85643539959774273, 8.980655621775115449, -3.220279653634019468 ) ) ;
#7736=CARTESIAN_POINT ( 'NONE',  ( 23.43555436076258047, 3.792607145904837829, -3.105262516303788800 ) ) ;
#7740=CARTESIAN_POINT ( 'NONE',  ( -74.03255566204833826, -1.800923653458333273, -9.560995967708043608 ) ) ;
#7748=CARTESIAN_POINT ( 'NONE',  ( -70.31483849620295246, 0.01762406564628603983, 9.981599438687137393 ) ) ;
#7754=AXIS2_PLACEMENT_3D ( 'NONE', #37603, #3277, #37202 ) ;
#7756=CARTESIAN_POINT ( 'NONE',  ( 34.13608517534122910, -3.137549310921635470, 5.534159694588579370 ) ) ;
#7759=CARTESIAN_POINT ( 'NONE',  ( 86.31714526353648864, 1.402210177843808081, 5.108895447378689170 ) ) ;
#7765=CARTESIAN_POINT ( 'NONE',  ( -80.88140849387957587, 11.46041792646347268, -1.055489314687744207 ) ) ;
#7766=DIRECTION ( 'NONE',  ( 0.000000000000000000, -0.000000000000000000, 1.000000000000000000 ) ) ;
#7771=ORIENTED_EDGE ( 'NONE', *, *, #29780, .T. ) ;
#7775=CARTESIAN_POINT ( 'NONE',  ( 27.06702955060504578, 1.340722218708290114, 4.422313656526443815 ) ) ;
#7779=CARTESIAN_POINT ( 'NONE',  ( 14.69558838330753936, 10.99631180437154399, 5.999999999999998224 ) ) ;
#7784=CARTESIAN_POINT ( 'NONE',  ( 22.26302464024987060, 4.951729634934853408, -3.260511412105697282 ) ) ;
#7786=CARTESIAN_POINT ( 'NONE',  ( -83.92837670882109080, 2.429809908903242999, -12.50000000000000000 ) ) ;
#7787=CARTESIAN_POINT ( 'NONE',  ( 22.42980438978510449, 1.271109115893125585, 8.904229291692644210 ) ) ;
#7788=CARTESIAN_POINT ( 'NONE',  ( 16.28258120957830712, 10.03625422200891570, 2.499999999999521272 ) ) ;
#7791=CARTESIAN_POINT ( 'NONE',  ( 86.69422455818764206, -0.1941184515037400471, -5.886102099071623073 ) ) ;
#7798=CARTESIAN_POINT ( 'NONE',  ( 14.83377924836928763, -6.137502382583376992, -2.521568026651588301 ) ) ;
#7799=CARTESIAN_POINT ( 'NONE',  ( 36.44628851498989519, -2.355918992659408406, -5.894722798219696358 ) ) ;
#7800=CARTESIAN_POINT ( 'NONE',  ( -70.92837670882107659, 13.87661300689599386, 0.000000000000000000 ) ) ;
#7801=CARTESIAN_POINT ( 'NONE',  ( 84.11566709744786863, 2.998976903239075842, -0.6299403505785813318 ) ) ;
#7803=CARTESIAN_POINT ( 'NONE',  ( 30.05768800033484567, -3.720313780293153183, -4.561934355542292430 ) ) ;
#7812=CARTESIAN_POINT ( 'NONE',  ( 23.38580533471466438, 3.559992555223038924, 3.092799683450411230 ) ) ;
#7814=CARTESIAN_POINT ( 'NONE',  ( 33.45208957067621469, -3.251134754649326553, 5.427405637984302089 ) ) ;
#7820=ORIENTED_EDGE ( 'NONE', *, *, #1697, .F. ) ;
#7824=ORIENTED_EDGE ( 'NONE', *, *, #30559, .F. ) ;
#7825=CARTESIAN_POINT ( 'NONE',  ( 24.54631049625050565, 2.974125097758586911, 3.602083437275587219 ) ) ;
#7829=ORIENTED_EDGE ( 'NONE', *, *, #28970, .T. ) ;
#7833=CARTESIAN_POINT ( 'NONE',  ( 21.58930880649559469, 5.738281464677914556, -3.444703897471878218 ) ) ;
#7835=CARTESIAN_POINT ( 'NONE',  ( 22.94681503686735979, 2.560486077929890136, -4.549303765806815392 ) ) ;
#7837=EDGE_CURVE ( 'NONE', #17583, #13035, #16112, .T. ) ;
#7838=DIRECTION ( 'NONE',  ( -1.000000000000000000, 0.000000000000000000, 0.000000000000000000 ) ) ;
#7839=AXIS2_PLACEMENT_3D ( 'NONE', #1426, #29807, #33112 ) ;
#7844=CARTESIAN_POINT ( 'NONE',  ( 86.36291470068610465, 1.350799773688788674, 4.987004148466622766 ) ) ;
#7845=CARTESIAN_POINT ( 'NONE',  ( 31.00707005056823817, -0.8718966892480422004, 5.891928739871540088 ) ) ;
#7847=CARTESIAN_POINT ( 'NONE',  ( -81.79890681550139675, 10.46299657128043314, 0.6911394749367771873 ) ) ;
#7848=CARTESIAN_POINT ( 'NONE',  ( -72.99860296447080543, 0.8259586708074142525, -10.94618862030606898 ) ) ;
#7851=CARTESIAN_POINT ( 'NONE',  ( 36.24028759768958707, -2.130151203274132765, -5.862571372923810031 ) ) ;
#7854=ADVANCED_FACE ( 'NONE', ( #34881 ), #19205, .T. ) ;
#7861=CARTESIAN_POINT ( 'NONE',  ( 37.05414849786873788, -3.059465710589756249, 5.984234486237220985 ) ) ;
#7866=EDGE_LOOP ( 'NONE', ( #9943, #193, #30943, #22848 ) ) ;
#7875=VERTEX_POINT ( 'NONE', #14616 ) ;
#7881=CARTESIAN_POINT ( 'NONE',  ( 24.74497300857456850, 0.5733567267288544045, 4.778227254168478488 ) ) ;
#7887=CARTESIAN_POINT ( 'NONE',  ( 37.17969408807407916, -3.008184067405535345, -5.999999779455217563 ) ) ;
#7889=CARTESIAN_POINT ( 'NONE',  ( 14.69558838330753758, 3.996311804371543985, 6.000000000000000000 ) ) ;
#7890=CARTESIAN_POINT ( 'NONE',  ( 26.56638717734885802, 2.990222579127657099, 1.122734419917069237 ) ) ;
#7894=CARTESIAN_POINT ( 'NONE',  ( 24.12519416928313731, 0.5064133828745956967, -5.093109222506538636 ) ) ;
#7901=CARTESIAN_POINT ( 'NONE',  ( 37.00777520336294657, -3.244670941504010919, -5.947354996402821392 ) ) ;
#7902=FACE_OUTER_BOUND ( 'NONE', #32845, .T. ) ;
#7906=CARTESIAN_POINT ( 'NONE',  ( -69.92837670882107659, -23.80776546975053520, 9.949874371066204759 ) ) ;
#7909=EDGE_CURVE ( 'NONE', #14684, #20444, #39749, .T. ) ;
#7910=VERTEX_POINT ( 'NONE', #15241 ) ;
#7915=CARTESIAN_POINT ( 'NONE',  ( 86.43572624768424362, -0.5192074800720991590, -5.777013305174518720 ) ) ;
#7916=CARTESIAN_POINT ( 'NONE',  ( -81.80090188080514224, -5.603160304130404334, -0.6545554231109831367 ) ) ;
#7932=CARTESIAN_POINT ( 'NONE',  ( 21.85643539959776760, 10.44946649885084966, 7.640826779728119078 ) ) ;
#7936=CARTESIAN_POINT ( 'NONE',  ( 14.61802060940782155, -4.492733667522514907, 2.499999999999997780 ) ) ;
#7937=CARTESIAN_POINT ( 'NONE',  ( -77.10359778981232637, 9.587385728467753054, -7.883471332551708066 ) ) ;
#7939=CARTESIAN_POINT ( 'NONE',  ( -4.266520354791871306, -48.67644278316300444, -6.000000000000000000 ) ) ;
#7941=LINE ( 'NONE', #23198, #25539 ) ;
#7943=DIRECTION ( 'NONE',  ( 0.000000000000000000, 0.000000000000000000, 1.000000000000000000 ) ) ;
#7951=B_SPLINE_CURVE_WITH_KNOTS ( 'NONE', 3,
 ( #15799, #9399, #15590, #5924, #21986, #34767, #163, #37806, #18463, #6739 ),
 .UNSPECIFIED., .F., .F.,
 ( 4, 2, 2, 2, 4 ),
 ( 0.001564566806966613413, 0.001955354412007498724, 0.002346142017048383818, 0.002736929622089268911, 0.003127717227130154005 ),
 .UNSPECIFIED. ) ;
#7953=CARTESIAN_POINT ( 'NONE',  ( 36.78962651020381713, -3.042574519117287490, 5.948308996033500939 ) ) ;
#7955=CARTESIAN_POINT ( 'NONE',  ( 87.78348876263190448, -0.2448564372010923473, 4.525229423219702340 ) ) ;
#7962=CARTESIAN_POINT ( 'NONE',  ( -61.24591834330252027, -49.47158280949359010, -2.500000000000000000 ) ) ;
#7966=CARTESIAN_POINT ( 'NONE',  ( 24.91734749558309758, 3.524439253337528832, -0.6529367285399855225 ) ) ;
#7968=CARTESIAN_POINT ( 'NONE',  ( 25.84367263793748393, 1.600840454158463322, 4.297283297516126588 ) ) ;
#7976=CARTESIAN_POINT ( 'NONE',  ( 24.46786998095842591, 2.964482678099346291, -3.659345439263766764 ) ) ;
#7980=CARTESIAN_POINT ( 'NONE',  ( 21.85643539959774273, 9.214175136349357587, -0.8338435668127727185 ) ) ;
#7981=CARTESIAN_POINT ( 'NONE',  ( 16.14085267862078510, 12.58767977203877741, 2.500000000000000444 ) ) ;
#7984=CARTESIAN_POINT ( 'NONE',  ( 84.35358620389857265, 3.041238144818853684, 1.123552906098365112 ) ) ;
#7989=LINE ( 'NONE', #27749, #35511 ) ;
#7990=CARTESIAN_POINT ( 'NONE',  ( 14.83986818923396456, -4.481383445363374740, -2.516351727591476184 ) ) ;
#7991=EDGE_CURVE ( 'NONE', #8630, #15393, #17185, .T. ) ;
#7992=CARTESIAN_POINT ( 'NONE',  ( 34.77305545370109030, -3.160087570433653514, -5.633574311711002203 ) ) ;
#7994=CARTESIAN_POINT ( 'NONE',  ( 25.26334528616294151, 0.8481682192316492008, -4.614059732833895033 ) ) ;
#7995=CARTESIAN_POINT ( 'NONE',  ( 29.71865375326818537, -3.785866092356776402, -4.452099570374444149 ) ) ;
#7997=CARTESIAN_POINT ( 'NONE',  ( 36.14140113770966423, -3.140483868442980775, 5.847137749265862716 ) ) ;
#8003=CARTESIAN_POINT ( 'NONE',  ( 21.73971162413815250, 4.236108717388963996, 2.798398138428574100 ) ) ;
#8010=VERTEX_POINT ( 'NONE', #18117 ) ;
#8018=CARTESIAN_POINT ( 'NONE',  ( 22.75783442990022820, 3.925414047687008523, 3.607444980655814870 ) ) ;
#8022=CARTESIAN_POINT ( 'NONE',  ( 18.11164821838002581, -2.856713029497280232, -3.033158754982376859 ) ) ;
#8025=CARTESIAN_POINT ( 'NONE',  ( 23.12551116169677812, 2.829306214856787349, -4.256801911362003921 ) ) ;
#8027=EDGE_CURVE ( 'NONE', #15998, #6497, #27600, .T. ) ;
#8033=CARTESIAN_POINT ( 'NONE',  ( 86.17935586795600500, 1.556981766839054426, 4.792924669753763744 ) ) ;
#8034=CARTESIAN_POINT ( 'NONE',  ( 33.81722006525239266, -4.984950771528167124, -3.153948780582495726 ) ) ;
#8042=CARTESIAN_POINT ( 'NONE',  ( 36.43203232075673270, -3.203092416211517524, -5.892497774322134951 ) ) ;
#8047=VERTEX_POINT ( 'NONE', #30709 ) ;
#8048=CARTESIAN_POINT ( 'NONE',  ( 35.81810683760681968, -3.623504837237730314, 5.691522942300115240 ) ) ;
#8056=CARTESIAN_POINT ( 'NONE',  ( 86.00134810727946899, 0.2530519298808260320, -5.999722280616810899 ) ) ;
#8057=CARTESIAN_POINT ( 'NONE',  ( -78.38494362056192699, 11.33516465962242670, 6.676281561881168614 ) ) ;
#8062=CARTESIAN_POINT ( 'NONE',  ( 22.19016211074803380, 5.251790732463271105, 3.087872149380293418 ) ) ;
#8068=CARTESIAN_POINT ( 'NONE',  ( 21.97297751200100535, 0.2232358743075266438, 7.728093094151400777 ) ) ;
#8070=EDGE_CURVE ( 'NONE', #9413, #8271, #34961, .T. ) ;
#8075=LINE ( 'NONE', #21064, #16182 ) ;
#8079=CARTESIAN_POINT ( 'NONE',  ( 26.62075075102985267, 2.678422205045695392, 2.704210781993271695 ) ) ;
#8080=VERTEX_POINT ( 'NONE', #17228 ) ;
#8082=CARTESIAN_POINT ( 'NONE',  ( 23.05347533656128078, 0.3447057208869356293, -5.959858412725844268 ) ) ;
#8087=CARTESIAN_POINT ( 'NONE',  ( 29.48679710191445480, 1.217383870121761857, -4.226918706498755007 ) ) ;
#8112=CARTESIAN_POINT ( 'NONE',  ( 17.82514639985922855, 11.84176496571321202, -2.500000000000005773 ) ) ;
#8118=CARTESIAN_POINT ( 'NONE',  ( 18.33573041183021957, 13.40081273568012676, 2.499999999999999556 ) ) ;
#8119=CARTESIAN_POINT ( 'NONE',  ( 21.85643539959779602, 5.813509198596546135, -11.62788251339591206 ) ) ;
#8121=CARTESIAN_POINT ( 'NONE',  ( -76.85200812145377824, 9.438718831883464944, 8.072108724517537581 ) ) ;
#8123=CARTESIAN_POINT ( 'NONE',  ( 14.62957350336051299, -4.708282797761865979, 2.500000000000223377 ) ) ;
#8126=CARTESIAN_POINT ( 'NONE',  ( -78.25485146663302771, 11.30612734474080305, -6.818008430746309578 ) ) ;
#8127=CARTESIAN_POINT ( 'NONE',  ( 14.61802081865033820, 12.33286846116140190, 2.500000000000000000 ) ) ;
#8133=CARTESIAN_POINT ( 'NONE',  ( 31.50273333289666766, -0.4788391926020078571, 5.123161451720045001 ) ) ;
#8136=CARTESIAN_POINT ( 'NONE',  ( 87.88065579682655937, -0.3539990618341573025, 3.436608579331488666 ) ) ;
#8141=CARTESIAN_POINT ( 'NONE',  ( 37.06191389059799945, -2.795325952453375784, 5.990806027039132786 ) ) ;
#8142=ORIENTED_EDGE ( 'NONE', *, *, #36261, .F. ) ;
#8144=CARTESIAN_POINT ( 'NONE',  ( 88.05979627311084812, -0.5552181473167765446, -3.927858985986737661 ) ) ;
#8158=CARTESIAN_POINT ( 'NONE',  ( 21.97258699089572787, 0.9762916292323234879, 6.992449600740251014 ) ) ;
#8166=CARTESIAN_POINT ( 'NONE',  ( 59.69572451838116933, -0.8894979772356270686, -6.000000000000000000 ) ) ;
#8170=CARTESIAN_POINT ( 'NONE',  ( 22.52956484789606506, 4.299479892231873102, -3.494393047605991676 ) ) ;
#8173=CARTESIAN_POINT ( 'NONE',  ( 22.56491764776242803, -2.112007571549842755, -8.936849366082922685 ) ) ;
#8175=DIRECTION ( 'NONE',  ( 0.000000000000000000, 1.000000000000000000, 0.000000000000000000 ) ) ;
#8177=CARTESIAN_POINT ( 'NONE',  ( 88.70663687723717317, -1.959581838532896025, -1.901098908833099621 ) ) ;
#8181=CIRCLE ( 'NONE', #38435, 2.500000000000000444 ) ;
#8182=CARTESIAN_POINT ( 'NONE',  ( 23.38224997196427069, 4.144869090478608520, -2.193203930993182116 ) ) ;
#8183=CARTESIAN_POINT ( 'NONE',  ( 26.27012936093719020, -2.986060737681520916, -4.299671860209199892 ) ) ;
#8184=CARTESIAN_POINT ( 'NONE',  ( 37.04540850726244372, -2.801148728805186394, -5.988229962785414529 ) ) ;
#8186=CARTESIAN_POINT ( 'NONE',  ( 21.81064708091828663, 0.2586250352159095711, -8.253171913261097004 ) ) ;
#8189=CARTESIAN_POINT ( 'NONE',  ( 36.64484841828976869, -2.463732939319398074, 5.925712873318776275 ) ) ;
#8194=CARTESIAN_POINT ( 'NONE',  ( 37.11057928807143469, -2.402894445895731756, 5.951415949967167052 ) ) ;
#8195=B_SPLINE_CURVE_WITH_KNOTS ( 'NONE', 3,
 ( #21607, #5953, #18918, #18495, #12528, #2891, #15410, #15624, #27969, #12325, #24899, #18703, #9430, #28172, #22018, #34593, #6367, #31486, #20120, #39044, #16427, #32899, #23421, #13754, #16822 ),
 .UNSPECIFIED., .F., .F.,
 ( 4, 2, 1, 2, 2, 1, 1, 2, 2, 1, 2, 2, 1, 2, 4 ),
 ( 0.3785350882168260211, 0.4562182021897382977, 0.4950597591761943805, 0.4999149537995015713, 0.5023425511111547781, 0.5047701484228080959, 0.5144805376694194798, 0.5339013161626424697, 0.6892675441084263888, 0.7281091010948728126, 0.7475298795880955804, 0.7572402688347070754, 0.7669506580813184593, 0.8446337720542123062, 1.000000000000000000 ),
 .UNSPECIFIED. ) ;
#8201=ORIENTED_EDGE ( 'NONE', *, *, #7448, .F. ) ;
#8206=CARTESIAN_POINT ( 'NONE',  ( 14.74038269587535233, -4.698843100384389793, 2.506102901012715822 ) ) ;
#8211=CARTESIAN_POINT ( 'NONE',  ( 24.14924257540585728, 3.081831650159815084, 3.622205791944524744 ) ) ;
#8218=CARTESIAN_POINT ( 'NONE',  ( -70.92837670882107659, -65.19654454972992141, 0.000000000000000000 ) ) ;
#8219=CARTESIAN_POINT ( 'NONE',  ( 22.74155280133190260, -2.655454342507609145, -3.755767339817497774 ) ) ;
#8222=CARTESIAN_POINT ( 'NONE',  ( 22.97307122621484865, 2.409484201040166251, -4.646973716149349620 ) ) ;
#8223=EDGE_LOOP ( 'NONE', ( #27328, #37364, #8201, #28998 ) ) ;
#8225=CARTESIAN_POINT ( 'NONE',  ( 16.11725891508299924, 15.27317977276803873, 2.500000000000000000 ) ) ;
#8230=CARTESIAN_POINT ( 'NONE',  ( 87.61456772748933020, -0.05511631305283664489, -4.124113870075747812 ) ) ;
#8231=CARTESIAN_POINT ( 'NONE',  ( 29.93139500891458127, 0.4880113553092989553, -5.118255730029571460 ) ) ;
#8232=CARTESIAN_POINT ( 'NONE',  ( -77.05165876229449395, -4.661780768167600009, -9.444144087646179742 ) ) ;
#8234=FACE_OUTER_BOUND ( 'NONE', #24737, .T. ) ;
#8236=CARTESIAN_POINT ( 'NONE',  ( 36.81799887185016473, -2.525268165826815459, -5.952737189256588124 ) ) ;
#8246=CARTESIAN_POINT ( 'NONE',  ( 36.70930901955060222, -3.420528228347338828, 5.875135601664768892 ) ) ;
#8250=ORIENTED_EDGE ( 'NONE', *, *, #1516, .F. ) ;
#8254=CARTESIAN_POINT ( 'NONE',  ( -79.60043556232082551, 11.50163111191179866, 4.996739675375823531 ) ) ;
#8260=CARTESIAN_POINT ( 'NONE',  ( 21.71651422438785417, 6.289002153562915254, 3.207190368607817810 ) ) ;
#8265=ORIENTED_EDGE ( 'NONE', *, *, #34074, .T. ) ;
#8267=CARTESIAN_POINT ( 'NONE',  ( 22.28288117080667163, 0.2420143529008198235, 7.135959080246487396 ) ) ;
#8268=CARTESIAN_POINT ( 'NONE',  ( 14.74221411508265689, -5.125435651542595394, -2.499999999999999556 ) ) ;
#8271=VERTEX_POINT ( 'NONE', #37399 ) ;
#8272=CARTESIAN_POINT ( 'NONE',  ( 36.86728531260331465, -3.360612826157867605, -5.906623357289592313 ) ) ;
#8278=CARTESIAN_POINT ( 'NONE',  ( 26.75871784592184710, 2.055338430770167424, -4.125980934060708982 ) ) ;
#8282=CARTESIAN_POINT ( 'NONE',  ( -80.83308087135290521, -6.606543372238043332, 1.435207014940032444 ) ) ;
#8283=CARTESIAN_POINT ( 'NONE',  ( 21.73414427015508110, 0.2235801105871568495, -9.085705942277243707 ) ) ;
#8289=CARTESIAN_POINT ( 'NONE',  ( 37.00800308128324190, -3.245149801803746570, -5.947249437311571185 ) ) ;
#8290=CARTESIAN_POINT ( 'NONE',  ( 30.80771206660583061, -3.555147752975252651, -4.834189129258772866 ) ) ;
#8298=CARTESIAN_POINT ( 'NONE',  ( 23.71146206689260083, 1.800196029863365688, -4.690086670497853660 ) ) ;
#8300=EDGE_CURVE ( 'NONE', #10467, #32354, #1979, .T. ) ;
#8306=CARTESIAN_POINT ( 'NONE',  ( 87.91343731185466481, -2.496140582104141359, -0.8634702502314072214 ) ) ;
#8308=AXIS2_PLACEMENT_3D ( 'NONE', #18489, #31483, #191 ) ;
#8317=EDGE_CURVE ( 'NONE', #30447, #7067, #33848, .T. ) ;
#8320=CARTESIAN_POINT ( 'NONE',  ( 19.55994200078226797, 8.628030550684337996, -2.500000000001137757 ) ) ;
#8325=CARTESIAN_POINT ( 'NONE',  ( 21.78047233922835346, 5.616103166486084319, -3.473245622192032034 ) ) ;
#8326=CARTESIAN_POINT ( 'NONE',  ( -17.69482985384421880, -29.56993018339339940, 6.000000000000000000 ) ) ;
#8328=CARTESIAN_POINT ( 'NONE',  ( 21.85643539959778892, -10.77729622265174392, -9.134175241038137827 ) ) ;
#8330=CARTESIAN_POINT ( 'NONE',  ( -77.61846184184865649, 9.846684257009661323, 7.446037897971843122 ) ) ;
#8331=CARTESIAN_POINT ( 'NONE',  ( 14.72854306895793286, -5.062769318467021051, 2.500000000002235101 ) ) ;
#8333=CARTESIAN_POINT ( 'NONE',  ( -79.87311179269229910, 11.51046329118718958, -4.489559985497344030 ) ) ;
#8335=FACE_OUTER_BOUND ( 'NONE', #623, .T. ) ;
#8348=CARTESIAN_POINT ( 'NONE',  ( 33.68694953669930925, -3.106715461681162971, 5.464061215791960358 ) ) ;
#8352=CARTESIAN_POINT ( 'NONE',  ( 85.96608680028057847, 1.729603650198207054, 5.123763289084741324 ) ) ;
#8354=CARTESIAN_POINT ( 'NONE',  ( 31.24780275965614962, -0.3897380699759783740, -5.083373370246649259 ) ) ;
#8359=ORIENTED_EDGE ( 'NONE', *, *, #11986, .F. ) ;
#8368=CARTESIAN_POINT ( 'NONE',  ( 26.96776543102747681, 1.407182095274382982, 4.403121069298014056 ) ) ;
#8374=CARTESIAN_POINT ( 'NONE',  ( 87.04213330793392345, 0.5878691963682337596, 6.000000000000000000 ) ) ;
#8378=CARTESIAN_POINT ( 'NONE',  ( 23.42523798194068974, 3.747132905502745359, -3.204823688547873139 ) ) ;
#8381=ADVANCED_FACE ( 'NONE', ( #38407 ), #4463, .T. ) ;
#8382=CARTESIAN_POINT ( 'NONE',  ( 22.49462040199967916, -0.5704057512449431933, -9.208717712401224276 ) ) ;
#8386=CARTESIAN_POINT ( 'NONE',  ( 85.22136629666657370, 2.371628277241609517, -4.205523829021379001 ) ) ;
#8389=ORIENTED_EDGE ( 'NONE', *, *, #24928, .T. ) ;
#8396=CARTESIAN_POINT ( 'NONE',  ( 15.29064274479596719, -3.935957078823225874, -2.582637740313979968 ) ) ;
#8397=CARTESIAN_POINT ( 'NONE',  ( 36.79680087876906214, -2.557513486141199444, -5.949428729760880330 ) ) ;
#8398=DIRECTION ( 'NONE',  ( 0.000000000000000000, 1.000000000000000000, 0.000000000000000000 ) ) ;
#8399=CARTESIAN_POINT ( 'NONE',  ( 23.62653219015538042, 0.5414986629106450788, -5.462610290562567528 ) ) ;
#8402=CARTESIAN_POINT ( 'NONE',  ( 36.19294238595723812, -2.234500302844026010, 5.855182007584707193 ) ) ;
#8405=CARTESIAN_POINT ( 'NONE',  ( 85.36681891225420316, 2.469661840813765608, 2.484336716295309166 ) ) ;
#8409=CARTESIAN_POINT ( 'NONE',  ( 35.83265631856147593, -3.731003872579450764, 5.622499855908868582 ) ) ;
#8410=CARTESIAN_POINT ( 'NONE',  ( 30.67406393699503298, -3.593393542108534344, -4.777508688867102116 ) ) ;
#8418=VECTOR ( 'NONE', #18263, 1000.000000000000114 ) ;
#8421=CARTESIAN_POINT ( 'NONE',  ( 22.18094696048607517, 4.340889477042914280, 3.790884728818065597 ) ) ;
#8425=CARTESIAN_POINT ( 'NONE',  ( -5.316495087772350914, -32.84709638682603838, 0.000000000000000000 ) ) ;
#8426=CARTESIAN_POINT ( 'NONE',  ( 21.92193887068393110, -2.651946117302231620, -3.627846763502060590 ) ) ;
#8429=CARTESIAN_POINT ( 'NONE',  ( 24.01376084489890417, 2.453835260611390456, -4.174832439456215738 ) ) ;
#8432=CARTESIAN_POINT ( 'NONE',  ( -4.220127061295482087E-17, 0.7293679304675931840, 6.000000000000000000 ) ) ;
#8433=CARTESIAN_POINT ( 'NONE',  ( -4.890026461918814071, -8.228598103685714525E-16, -2.500000000000000000 ) ) ;
#8436=CARTESIAN_POINT ( 'NONE',  ( 88.35060396620406209, -0.8818671507646100860, -0.7863509125847466530 ) ) ;
#8437=CARTESIAN_POINT ( 'NONE',  ( 29.97939791730999914, 0.4010955892747467555, 5.210136963171234648 ) ) ;
#8444=CARTESIAN_POINT ( 'NONE',  ( 36.42653508247762772, -3.159901027683388985, -5.891639797337469453 ) ) ;
#8449=EDGE_CURVE ( 'NONE', #34557, #25138, #764, .T. ) ;
#8453=CARTESIAN_POINT ( 'NONE',  ( 29.41998804195583972, 1.119444561410238625, 4.432470294405459477 ) ) ;
#8456=CARTESIAN_POINT ( 'NONE',  ( -71.54296365563132554, 0.01656620227473614565, 9.981524770340062247 ) ) ;
#8462=CARTESIAN_POINT ( 'NONE',  ( -73.84684882489183622, 8.474083953686129433, 9.568945070976022649 ) ) ;
#8463=B_SPLINE_CURVE_WITH_KNOTS ( 'NONE', 3,
 ( #17494, #33399, #36458, #7848, #36070, #17297, #29876, #20595, #23506, #1486, #1690, #7443, #20400, #14223, #39334, #26990, #33181, #17100, #8232, #32978, #20803, #26592, #4378, #5171, #26796, #29280, #1092, #11124, #23694, #1901, #20201, #32784, #14421, #13629, #10927, #36262 ),
 .UNSPECIFIED., .F., .F.,
 ( 4, 2, 2, 2, 2, 2, 2, 2, 2, 2, 2, 2, 2, 2, 2, 2, 2, 4 ),
 ( 0.02000509599350686063, 0.02121644006951485875, 0.02242778414552285687, 0.02363912822153085153, 0.02485047229753884965, 0.02606181637354684777, 0.02666748841155085897, 0.02727316044955487018, 0.02848450452556289259, 0.02909017656356688991, 0.02969584860157088724, 0.03090719267757885066, 0.03211853675358681409, 0.03454122490560271319, 0.03575256898161066621, 0.03696391305761861923, 0.03817525713362657225, 0.03938660120963451833 ),
 .UNSPECIFIED. ) ;
#8468=CARTESIAN_POINT ( 'NONE',  ( 23.14034614274038049, 4.027993350838696252, 3.114739222192818069 ) ) ;
#8471=AXIS2_PLACEMENT_3D ( 'NONE', #33940, #15173, #5506 ) ;
#8475=CARTESIAN_POINT ( 'NONE',  ( 23.58567603336324225, 0.4095245276899994180, 5.530613567852399548 ) ) ;
#8476=CARTESIAN_POINT ( 'NONE',  ( 14.72888393404697638, -5.064079573351400576, -2.499999999997913669 ) ) ;
#8481=CARTESIAN_POINT ( 'NONE',  ( 37.19747295490952155, -2.841588721108153415, -5.999818660317219887 ) ) ;
#8485=CARTESIAN_POINT ( 'NONE',  ( 63.05383694556373797, -7.271989087314214117, 6.000000000000000000 ) ) ;
#8486=ORIENTED_EDGE ( 'NONE', *, *, #25680, .F. ) ;
#8487=CARTESIAN_POINT ( 'NONE',  ( 27.99192205930350497, 2.110044335382625924, -3.171593750069938711 ) ) ;
#8491=CARTESIAN_POINT ( 'NONE',  ( 21.73475704421919374, 0.2471461942093770570, -9.024413037465413012 ) ) ;
#8492=AXIS2_PLACEMENT_3D ( 'NONE', #6244, #275, #12413 ) ;
#8493=PLANE ( 'NONE',  #7712 ) ;
#8494=DIRECTION ( 'NONE',  ( 0.9616058754224561245, -0.2744342186262704875, 0.000000000000000000 ) ) ;
#8497=CARTESIAN_POINT ( 'NONE',  ( 36.88745072424094218, -3.349843832818609979, -5.911037807513603859 ) ) ;
#8505=CARTESIAN_POINT ( 'NONE',  ( 23.79294960832602257, 1.583767941604382390, -4.781311079654926743 ) ) ;
#8507=EDGE_CURVE ( 'NONE', #1678, #12553, #38128, .T. ) ;
#8509=ORIENTED_EDGE ( 'NONE', *, *, #35184, .F. ) ;
#8520=CARTESIAN_POINT ( 'NONE',  ( -16.27783086239806210, 25.90100547710869705, 2.500000000000000000 ) ) ;
#8525=ORIENTED_EDGE ( 'NONE', *, *, #34074, .F. ) ;
#8528=CARTESIAN_POINT ( 'NONE',  ( 15.87703798546623801, 7.971370176595764079, -3.484773916741099153 ) ) ;
#8535=CARTESIAN_POINT ( 'NONE',  ( 8.290806648384990041, -33.63722727088462250, 27.90461065042423527 ) ) ;
#8537=CARTESIAN_POINT ( 'NONE',  ( 21.85643539959774273, 10.54442680926682208, -0.8960936389291185300 ) ) ;
#8542=CARTESIAN_POINT ( 'NONE',  ( -76.33197261733621986, 9.105972672263392909, -8.440813136491913227 ) ) ;
#8545=B_SPLINE_CURVE_WITH_KNOTS ( 'NONE', 5,
 ( #2779, #40618, #90, #31373, #15511, #37529, #27857, #24786 ),
 .UNSPECIFIED., .F., .F.,
 ( 6, 2, 6 ),
 ( 0.000000000000000000, 0.5000000000000000000, 1.000000000000000000 ),
 .UNSPECIFIED. ) ;
#8547=CARTESIAN_POINT ( 'NONE',  ( 14.82857513895052293, 12.56830691318596038, 2.515104768166851468 ) ) ;
#8549=LINE ( 'NONE', #11625, #24727 ) ;
#8558=CARTESIAN_POINT ( 'NONE',  ( 85.16823716249373888, 2.433965874742513247, 4.055466505201608562 ) ) ;
#8560=CARTESIAN_POINT ( 'NONE',  ( -71.92837670882107659, -20.91528738869522286, 5.916079783099629452 ) ) ;
#8564=CARTESIAN_POINT ( 'NONE',  ( 86.41986477775893150, 1.286830744106879143, 5.024081974984663468 ) ) ;
#8565=CARTESIAN_POINT ( 'NONE',  ( -70.42514326790677615, -21.65690572916051693, 5.980075040747969695 ) ) ;
#8567=ORIENTED_EDGE ( 'NONE', *, *, #15859, .T. ) ;
#8571=ORIENTED_EDGE ( 'NONE', *, *, #624, .F. ) ;
#8575=CARTESIAN_POINT ( 'NONE',  ( 25.90465186428314581, 0.9472713440299531662, 4.432119623292119392 ) ) ;
#8587=CARTESIAN_POINT ( 'NONE',  ( 22.66364520782453340, 4.448174091865554125, -3.201175655495145378 ) ) ;
#8592=CARTESIAN_POINT ( 'NONE',  ( 22.53035139435667844, 7.500704155568330478, 2.500000000000002220 ) ) ;
#8595=CARTESIAN_POINT ( 'NONE',  ( 87.73660070961769009, -1.594395026316068220, -4.241058185374163791 ) ) ;
#8600=CARTESIAN_POINT ( 'NONE',  ( 14.77855825630049225, -5.586149576324408450, -2.503853264347463803 ) ) ;
#8607=CARTESIAN_POINT ( 'NONE',  ( 85.75774791330482572, 2.030551832223961295, -3.840166728450957301 ) ) ;
#8611=CARTESIAN_POINT ( 'NONE',  ( 21.74038206013705121, 4.236694097800127068, 2.795633394849727615 ) ) ;
#8612=CARTESIAN_POINT ( 'NONE',  ( 17.88044828116697005, -3.178183975948303264, -2.955689043506722236 ) ) ;
#8613=CARTESIAN_POINT ( 'NONE',  ( 14.65885757255328414, 12.91887598178976937, -2.499999999999998668 ) ) ;
#8623=CARTESIAN_POINT ( 'NONE',  ( 23.47273670061042594, 2.435374625252711756, 4.369794992912356513 ) ) ;
#8630=VERTEX_POINT ( 'NONE', #23584 ) ;
#8637=CARTESIAN_POINT ( 'NONE',  ( 23.51549670196803632, 2.969767605084016715, -3.961303977705219914 ) ) ;
#8640=CARTESIAN_POINT ( 'NONE',  ( 21.85643539959775694, 5.983772091205654675, 13.40455955530236487 ) ) ;
#8643=DIRECTION ( 'NONE',  ( 1.000000000000000000, 1.682730792515357087E-16, -0.000000000000000000 ) ) ;
#8645=CARTESIAN_POINT ( 'NONE',  ( 86.49834695356116754, 1.198675839257056230, 5.248227958817050620 ) ) ;
#8646=CARTESIAN_POINT ( 'NONE',  ( -61.57369240569498459, -49.47615685354814019, -3.769463484964756361 ) ) ;
#8649=CARTESIAN_POINT ( 'NONE',  ( 15.62809155304131004, -3.765067253224523736, 2.629774229783644834 ) ) ;
#8651=CARTESIAN_POINT ( 'NONE',  ( 33.68680002607173662, -3.106704734317021099, -5.464037881042599132 ) ) ;
#8658=CARTESIAN_POINT ( 'NONE',  ( 37.19501073558123494, -2.749265500231607096, 6.000935497143758290 ) ) ;
#8663=ORIENTED_EDGE ( 'NONE', *, *, #12031, .T. ) ;
#8665=CARTESIAN_POINT ( 'NONE',  ( -72.01455954249333047, 4.687226239598052402, -9.941142508676179546 ) ) ;
#8667=DIRECTION ( 'NONE',  ( -0.000000000000000000, -0.000000000000000000, -1.000000000000000000 ) ) ;
#8672=CARTESIAN_POINT ( 'NONE',  ( 23.42902919107597981, 3.774424825821157459, 3.149840774630959128 ) ) ;
#8678=CARTESIAN_POINT ( 'NONE',  ( 24.12053105157879784, 0.4789250373359598689, 5.097972069152276298 ) ) ;
#8679=CARTESIAN_POINT ( 'NONE',  ( 14.70693164707954459, -5.039500861583466218, -2.499999999999853895 ) ) ;
#8684=EDGE_CURVE ( 'NONE', #18532, #8010, #22112, .T. ) ;
#8685=EDGE_CURVE ( 'NONE', #38217, #21520, #5246, .T. ) ;
#8686=CARTESIAN_POINT ( 'NONE',  ( 36.15253105956762170, -3.657967514016432720, -5.706993152568901273 ) ) ;
#8692=CARTESIAN_POINT ( 'NONE',  ( 29.60575365153160732, -0.8332953136462766253, 6.005451346670388268 ) ) ;
#8695=CARTESIAN_POINT ( 'NONE',  ( -80.88216618113609968, -5.699911949738533323, 1.044490278467241184 ) ) ;
#8696=CARTESIAN_POINT ( 'NONE',  ( 21.73453909374078563, 0.2390742653956647312, -9.045263263313582769 ) ) ;
#8701=CARTESIAN_POINT ( 'NONE',  ( 30.84892909652827697, 0.6455663479207958133, -4.592247333245458307 ) ) ;
#8703=CARTESIAN_POINT ( 'NONE',  ( 27.14650909609752816, 1.283972158900671623, -4.437200329386957520 ) ) ;
#8708=CARTESIAN_POINT ( 'NONE',  ( -75.54006495261842247, 8.454230440140586111, 10.26970949974186986 ) ) ;
#8711=CARTESIAN_POINT ( 'NONE',  ( 23.12838916460015071, 1.463821817805705194, -5.240134305553244332 ) ) ;
#8713=VERTEX_POINT ( 'NONE', #10677 ) ;
#8718=CARTESIAN_POINT ( 'NONE',  ( 85.71231987865445490, 0.7872592507033150389, 5.912482239253596283 ) ) ;
#8726=CARTESIAN_POINT ( 'NONE',  ( 24.76601816127300637, 3.022843676862287499, 3.334302330152292271 ) ) ;
#8730=CARTESIAN_POINT ( 'NONE',  ( 23.31126841323469989, 9.638235061640909151, -2.500000000000000444 ) ) ;
#8737=CARTESIAN_POINT ( 'NONE',  ( 21.85643539959776760, 7.145415623174192987, -7.905327125498018859 ) ) ;
#8739=CARTESIAN_POINT ( 'NONE',  ( -79.86284581725708165, 10.49264010779607048, 4.509636572782145691 ) ) ;
#8741=CARTESIAN_POINT ( 'NONE',  ( -69.92837670882107659, -20.78299143688747819, 5.916079783099617906 ) ) ;
#8742=CARTESIAN_POINT ( 'NONE',  ( -73.23469688983234960, 4.928437080168684759, -9.790059002995628035 ) ) ;
#8744=CARTESIAN_POINT ( 'NONE',  ( 36.71952137777376635, -3.460392053857834327, -5.859972560675125841 ) ) ;
#8746=CARTESIAN_POINT ( 'NONE',  ( 15.16058069087244853, 11.94051475997482648, 2.549013982532239098 ) ) ;
#8748=CARTESIAN_POINT ( 'NONE',  ( 29.06645441453732559, -3.924731372528510676, 4.240759432255150507 ) ) ;
#8750=CARTESIAN_POINT ( 'NONE',  ( -4.890026461918809630, -25.50263309590217276, -2.500000000000002220 ) ) ;
#8754=CARTESIAN_POINT ( 'NONE',  ( 24.77204021038152959, 2.610204331802961963, -3.937606257336461635 ) ) ;
#8756=CARTESIAN_POINT ( 'NONE',  ( -69.50551526817780257, -47.60185046458123281, 5.828975448080927713 ) ) ;
#8761=CARTESIAN_POINT ( 'NONE',  ( 88.42327724305060599, -1.151963697325209202, 3.685007885677881401 ) ) ;
#8762=CARTESIAN_POINT ( 'NONE',  ( 29.20860690094596634, 2.240472738085125037, 1.050758983225395848 ) ) ;
#8763=CARTESIAN_POINT ( 'NONE',  ( 33.60333658342298691, -1.218927361606251702, -5.451011392246272180 ) ) ;
#8772=CARTESIAN_POINT ( 'NONE',  ( 8.290806648384990041, -33.63722727088462250, 27.90461065042423527 ) ) ;
#8774=DIRECTION ( 'NONE',  ( 0.000000000000000000, 0.000000000000000000, -1.000000000000000000 ) ) ;
#8781=DIRECTION ( 'NONE',  ( 1.000000000000000000, 1.165409145176969993E-16, 0.000000000000000000 ) ) ;
#8784=CARTESIAN_POINT ( 'NONE',  ( 22.88660608767791160, 4.282592626049536833, -3.128843504308600920 ) ) ;
#8792=CARTESIAN_POINT ( 'NONE',  ( 85.28131701390645958, 1.700283277630491030, -5.218886290300497777 ) ) ;
#8800=CARTESIAN_POINT ( 'NONE',  ( 26.27016240683699877, -3.098343122671453731, -4.267664985417156664 ) ) ;
#8801=CARTESIAN_POINT ( 'NONE',  ( 35.45227351365613089, -1.918039355012105762, -5.739582716917785987 ) ) ;
#8804=CARTESIAN_POINT ( 'NONE',  ( 36.78876423199966439, -3.039631217886890724, 5.948174416665469089 ) ) ;
#8806=CARTESIAN_POINT ( 'NONE',  ( 88.35060396620406209, -0.8818671507646100860, -0.7863509125847466530 ) ) ;
#8807=ORIENTED_EDGE ( 'NONE', *, *, #6441, .F. ) ;
#8810=CARTESIAN_POINT ( 'NONE',  ( 37.01095259801031290, -2.247694374308371046, 5.912577408341228136 ) ) ;
#8811=EDGE_CURVE ( 'NONE', #8271, #21802, #18134, .T. ) ;
#8812=EDGE_CURVE ( 'NONE', #36468, #22420, #1848, .T. ) ;
#8813=CARTESIAN_POINT ( 'NONE',  ( 21.75262081531260350, -3.067555067785914691, -3.510010962324494610 ) ) ;
#8814=CARTESIAN_POINT ( 'NONE',  ( 14.68773611677202773, 12.90757323259234823, -2.500000034696362672 ) ) ;
#8825=CARTESIAN_POINT ( 'NONE',  ( 24.45417550923406935, 2.604819814871429884, 3.970987390700944086 ) ) ;
#8834=CARTESIAN_POINT ( 'NONE',  ( 85.15856829264210148, 2.703578820932674542, -0.6845625252714587772 ) ) ;
#8837=CARTESIAN_POINT ( 'NONE',  ( 23.91035688797384751, 2.995239222824085168, -3.797843349976805172 ) ) ;
#8839=CARTESIAN_POINT ( 'NONE',  ( 21.85643539959775694, 3.570402768353612810, -13.15459721397892423 ) ) ;
#8846=CARTESIAN_POINT ( 'NONE',  ( 88.00102923632725549, -0.4892082223494365611, 4.076460784956554839 ) ) ;
#8848=CARTESIAN_POINT ( 'NONE',  ( -4.890026461918807854, -25.50263309590217276, -6.000000000000001776 ) ) ;
#8852=CARTESIAN_POINT ( 'NONE',  ( 21.53525890830123046, 7.395493054481637074, 0.9774100666432447015 ) ) ;
#8853=CARTESIAN_POINT ( 'NONE',  ( 35.86956930648597108, -2.085467868944065550, -5.804711817725769940 ) ) ;
#8861=ORIENTED_EDGE ( 'NONE', *, *, #20884, .T. ) ;
#8862=CARTESIAN_POINT ( 'NONE',  ( 36.87708760085472903, -3.319687905980674536, 5.920000889922525822 ) ) ;
#8872=CARTESIAN_POINT ( 'NONE',  ( -75.29779855868427774, -5.030202623681788054, -9.000969684516388014 ) ) ;
#8873=CARTESIAN_POINT ( 'NONE',  ( 15.84007060359406083, 10.41087468735547716, 2.678624129882808180 ) ) ;
#8875=VERTEX_POINT ( 'NONE', #29824 ) ;
#8879=CARTESIAN_POINT ( 'NONE',  ( 24.68756320289947936, 2.996584696271434201, 3.466125977230326782 ) ) ;
#8895=ORIENTED_EDGE ( 'NONE', *, *, #37764, .F. ) ;
#8896=CARTESIAN_POINT ( 'NONE',  ( 31.79760674661912745, -3.928098387035230843, -4.516596916592202859 ) ) ;
#8900=CARTESIAN_POINT ( 'NONE',  ( 21.99536180190331791, 0.2400875630283233197, -7.664209021738525252 ) ) ;
#8902=EDGE_CURVE ( 'NONE', #14684, #22934, #7989, .T. ) ;
#8907=CARTESIAN_POINT ( 'NONE',  ( 36.87700637240019574, -3.319742436231731819, -5.919978869301625757 ) ) ;
#8916=CARTESIAN_POINT ( 'NONE',  ( 21.43086650153212247, 7.999394493581059251, 2.743190574498553413 ) ) ;
#8917=CARTESIAN_POINT ( 'NONE',  ( 22.27214042976725494, 1.964039760382519040, -5.564636450190440620 ) ) ;
#8924=ADVANCED_FACE ( 'NONE', ( #12307, #30657 ), #2467, .F. ) ;
#8932=CARTESIAN_POINT ( 'NONE',  ( 23.75454047524076273, 3.573438420936730253, 3.145647371460261965 ) ) ;
#8938=CARTESIAN_POINT ( 'NONE',  ( 21.85642363622424256, 10.16974155675050895, -2.500000000000000444 ) ) ;
#8944=CARTESIAN_POINT ( 'NONE',  ( 21.85643539959775339, 5.487231995601864476, 10.01193108169250578 ) ) ;
#8946=CARTESIAN_POINT ( 'NONE',  ( -72.89934385729463884, 3.418700917153234098, 9.863801266169547333 ) ) ;
#8950=CARTESIAN_POINT ( 'NONE',  ( 30.69044931928128150, -3.119424076483234387, -4.996384886243276924 ) ) ;
#8951=CARTESIAN_POINT ( 'NONE',  ( 36.20119281512496912, -3.652236176559757741, -5.717025003991615506 ) ) ;
#8954=CARTESIAN_POINT ( 'NONE',  ( 15.23756541667567177, 11.44821579467915917, 2.584588623821235220 ) ) ;
#8959=CARTESIAN_POINT ( 'NONE',  ( 24.58814725198859463, 2.979487925962025052, -3.568875956100880042 ) ) ;
#8963=CARTESIAN_POINT ( 'NONE',  ( 36.64797015977908501, -3.154251671283775593, 5.926200096577949772 ) ) ;
#8966=EDGE_CURVE ( 'NONE', #28414, #8713, #15773, .T. ) ;
#8968=CARTESIAN_POINT ( 'NONE',  ( 86.69901843299427924, 0.4902165918510832388, 5.965927736749048194 ) ) ;
#8972=CARTESIAN_POINT ( 'NONE',  ( 35.89239603134597445, -2.095832607348167453, -5.808274480206606860 ) ) ;
#8975=CARTESIAN_POINT ( 'NONE',  ( 24.55420261656340486, 2.734525497827099638, 3.876975801173430103 ) ) ;
#8980=VERTEX_POINT ( 'NONE', #37220 ) ;
#8985=CARTESIAN_POINT ( 'NONE',  ( 14.72021916802316710, 13.05558383789457189, 2.500000000000000444 ) ) ;
#8988=VECTOR ( 'NONE', #780, 1000.000000000000000 ) ;
#8992=CARTESIAN_POINT ( 'NONE',  ( 27.05168840568772737, -4.558788516904208166, 3.571571921055567866 ) ) ;
#8994=AXIS2_PLACEMENT_3D ( 'NONE', #23025, #4099, #23417 ) ;
#8995=DIRECTION ( 'NONE',  ( 1.000000000000000000, 1.385724075720358314E-16, -0.000000000000000000 ) ) ;
#8998=CARTESIAN_POINT ( 'NONE',  ( 22.03617269645906518, 5.395735386727952054, -3.201102023609922131 ) ) ;
#9002=CARTESIAN_POINT ( 'NONE',  ( -78.62055188009620110, -5.380212206548604215, -6.429298165712081570 ) ) ;
#9005=CARTESIAN_POINT ( 'NONE',  ( 88.33724419093491065, -2.316998127210522007, 1.237639510709749091 ) ) ;
#9007=VERTEX_POINT ( 'NONE', #40103 ) ;
#9012=CARTESIAN_POINT ( 'NONE',  ( 33.97726142433466379, -3.803478383426091458, -5.244974327395966363 ) ) ;
#9014=CARTESIAN_POINT ( 'NONE',  ( 85.59323660014052848, 0.9850445873831121801, 5.800130443767659294 ) ) ;
#9017=CARTESIAN_POINT ( 'NONE',  ( 36.99213799685487203, -2.719433212406895173, 5.979915811284242544 ) ) ;
#9019=LINE ( 'NONE', #30665, #36418 ) ;
#9023=CARTESIAN_POINT ( 'NONE',  ( 14.67630592591299532, -4.947493968569943945, 2.499999999999956035 ) ) ;
#9027=CARTESIAN_POINT ( 'NONE',  ( 14.62016757377762843, 13.26415307787954490, -2.488228758613686864 ) ) ;
#9028=CIRCLE ( 'NONE', #20200, 2.500000000000000444 ) ;
#9029=ORIENTED_EDGE ( 'NONE', *, *, #9667, .T. ) ;
#9036=CARTESIAN_POINT ( 'NONE',  ( 24.92005442864145692, 2.530202585715988217, 3.974294703006678642 ) ) ;
#9037=CARTESIAN_POINT ( 'NONE',  ( 34.15825286562033369, -0.5798779905139902491, 5.173835020267440576 ) ) ;
#9038=ORIENTED_EDGE ( 'NONE', *, *, #11639, .T. ) ;
#9048=CARTESIAN_POINT ( 'NONE',  ( 21.85761542531931667, 3.396825223608685995, -4.782081994692843452 ) ) ;
#9051=CARTESIAN_POINT ( 'NONE',  ( 21.85643539959774273, 11.87467848218428834, -0.9583437110454642305 ) ) ;
#9056=CARTESIAN_POINT ( 'NONE',  ( 88.25986434197210428, -0.7799440980648532085, -3.332403339731401015 ) ) ;
#9062=CARTESIAN_POINT ( 'NONE',  ( 23.84525472439710114, -3.061681620743719190, 3.851870993270792187 ) ) ;
#9064=CARTESIAN_POINT ( 'NONE',  ( 24.98419795007806599, 3.112932432632140145, 2.907112638396472715 ) ) ;
#9065=CARTESIAN_POINT ( 'NONE',  ( 36.79834255099314078, -2.555168371936516358, -5.949669344996932452 ) ) ;
#9067=B_SPLINE_CURVE_WITH_KNOTS ( 'NONE', 3,
 ( #23958, #27470, #5862, #2381 ),
 .UNSPECIFIED., .F., .F.,
 ( 4, 4 ),
 ( 0.1795419177415450984, 0.3391172959757620120 ),
 .UNSPECIFIED. ) ;
#9073=CARTESIAN_POINT ( 'NONE',  ( 34.13640354093743667, -3.787416915700777764, 5.295493011275766548 ) ) ;
#9080=CARTESIAN_POINT ( 'NONE',  ( 87.29047730454419707, 0.3089174322584790633, -4.712845393775586977 ) ) ;
#9081=CARTESIAN_POINT ( 'NONE',  ( -72.53275211461026117, 6.278950858466555651, -9.872183956496360935 ) ) ;
#9086=EDGE_LOOP ( 'NONE', ( #20552, #39708, #5410, #30730, #28705, #34228 ) ) ;
#9087=B_SPLINE_CURVE_WITH_KNOTS ( 'NONE', 3,
 ( #3317, #30888, #6379, #40130, #21203, #27577, #33777, #11910, #2700, #15218, #15417, #15837 ),
 .UNSPECIFIED., .F., .F.,
 ( 4, 2, 2, 2, 1, 1, 4 ),
 ( 0.000000000000000000, 0.3310684008954036806, 0.4966026013431050767, 0.5172943763990670574, 0.5379861514550290380, 0.5793697015669526662, 0.6621368017907995895 ),
 .UNSPECIFIED. ) ;
#9088=CARTESIAN_POINT ( 'NONE',  ( 22.88251133645001190, 4.300788154828764753, 3.108290358268387177 ) ) ;
#9107=FACE_OUTER_BOUND ( 'NONE', #6867, .T. ) ;
#9109=CARTESIAN_POINT ( 'NONE',  ( 33.86666996155606313, -5.260714354287511441, -2.203027216165969637 ) ) ;
#9114=CARTESIAN_POINT ( 'NONE',  ( 24.73558894963412769, 0.6121252408484304519, -4.779902904745515713 ) ) ;
#9119=CARTESIAN_POINT ( 'NONE',  ( 33.44004484032286229, -3.434887717533713580, -5.408154456503273977 ) ) ;
#9120=CARTESIAN_POINT ( 'NONE',  ( 21.67022219558699803, 4.173608694407422881, -3.080183803507759333 ) ) ;
#9128=VECTOR ( 'NONE', #32250, 1000.000000000000000 ) ;
#9130=CARTESIAN_POINT ( 'NONE',  ( 24.03622579959568029, 1.870140213503554527, -4.518823370007700291 ) ) ;
#9141=CARTESIAN_POINT ( 'NONE',  ( 22.18551630692656218, 5.282241039200648025, 3.062960712820621101 ) ) ;
#9148=EDGE_CURVE ( 'NONE', #20444, #13284, #35182, .T. ) ;
#9151=B_SPLINE_SURFACE_WITH_KNOTS ( 'NONE', 3, 3, ( 
 ( #4840, #24182, #1978, #17370, #29948, #14496, #27263, #36946, #18602, #5659, #21518, #9340, #2387 ),
 ( #40635, #2597, #18200, #34494, #28083, #37144, #37346, #27674, #37543, #12013, #19031, #18815, #34091 ),
 ( #34703, #105, #30992, #34300, #25210, #2797, #40421, #3008, #24806, #9141, #11802, #15733, #27479 ),
 ( #8726, #15116, #30790, #5867, #15525, #28285, #40229, #14912, #21715, #40032, #27875, #21918, #12638 ),
 ( #21306, #12438, #24590, #8932, #24386, #33882, #37739, #15321, #12228, #6068, #9548, #31187, #25005 ),
 ( #6268, #6479, #31389, #3213, #22129, #16529, #16720, #29106, #13657, #909, #26226, #13446, #28493 ),
 ( #1124, #514, #7271, #10147, #22738, #34905, #35699, #10553, #26021, #16329, #38761, #9955, #19834 ),
 ( #38352, #38551, #9757, #22538, #23130, #35301, #35101, #10361, #6877, #22936, #22337, #7471, #31593 ),
 ( #19432, #32007, #3417, #15929, #303, #12841, #3812, #28903, #32810, #30312, #20423, #30115, #29509 ),
 ( #36488, #4598, #1716, #14045, #39155, #4792, #14246, #33004, #35897, #23719, #4994, #11150, #10747 ),
 ( #14446, #1318, #17519, #17322, #29901, #29700, #26820, #39775, #36286, #24120, #36688, #23328, #20029 ),
 ( #32610, #7674, #33427, #2125, #23912, #4407, #5196, #17127, #20622, #8062, #33208, #13857, #17728 ),
 ( #1924, #26424, #20228, #1512, #23532, #27017, #14642, #26620, #16931, #39564, #10950, #11347, #8260 ),
 ( #27214, #36098, #20831, #11549, #8672, #8468, #5398, #34440, #21461, #14851, #21052, #3162, #5607 ),
 ( #18550, #17939, #55, #31134, #39980, #36893, #9088, #6218, #21664, #31338, #34242, #15680, #6014 ),
 ( #37294, #21864, #21252, #12386, #27818, #40370, #11752, #12585, #28228, #2952, #34036, #9285, #18145 ),
 ( #8879, #15267, #15468, #2330, #30734, #18763, #2744, #2538, #28029, #11958, #24745, #27417, #25151 ),
 ( #33623, #15063, #30520, #24329, #33824, #12174, #40576, #27621, #40177, #24535, #37089, #5809, #30938 ),
 ( #18348, #24954, #37490, #35453, #25561, #13603, #9491, #22077, #18979, #3965, #458, #9908, #31543 ),
 ( #16484, #37686, #28440, #16284, #248, #12786, #9706, #25361, #37899, #19179, #22285, #29057, #864 ),
 ( #34854, #13397, #31743, #3557, #22489, #35053, #25970, #19384, #31954, #38503, #36239, #35650, #23280 ),
 ( #7825, #20180, #4552, #10904, #20374, #13999, #1270, #29856, #11101, #4742, #4357, #23086, #20571 ),
 ( #23673, #26570, #39107, #35847, #32956, #5148, #1667, #30263, #2082, #29459, #26175, #13809, #26377 ),
 ( #23480, #8211, #20785, #39516, #39311, #10701, #36048, #7420, #11297, #17275, #32558, #7626, #38909 ),
 ( #19978, #14200, #32763, #17077, #33158, #38708, #29654, #8018, #1465, #26774, #17472, #4944, #30064 ),
 ( #1876, #14399, #26970, #10504, #23862, #33379, #17683, #30472, #17891, #24069, #8421, #14595, #36642 ),
 ( #33576, #27166, #39723, #5353, #20997, #11504, #19025, #16132, #32403, #31589, #7064, #19428, #6475 ),
 ( #13441, #25806, #4196, #3805, #903, #16714, #19828, #31999, #16325, #28898, #13241, #4006, #6873 ),
 ( #19633, #32207, #38346, #705, #22732, #10354, #16524, #15924, #7265, #10142, #35296, #9543, #12836 ),
 ( #19225, #25407, #29100, #29304, #26016, #38546, #22926, #35495, #37945, #12632, #13042, #3413, #25202 ),
 ( #37734, #28488, #31790, #22124, #34698, #6677, #296, #9753, #22332, #34900, #3606, #28696, #508 ),
 ( #25604, #38147, #9950, #22533, #35097, #40323, #33776, #27369, #22026, #24484, #31088, #37441, #36842 ),
 ( #9239, #18091, #15013, #27976, #12537, #40524, #9443, #12333, #34600, #24907, #24282, #15416, #5 ),
 ( #31291, #5959, #18504, #30684, #31492, #6378, #21816, #12116, #28180, #37040, #3113, #27771, #34194 ),
 ( #21202, #8825, #25109, #21614, #21410, #34398, #30887, #2898, #5553, #3316, #18926, #39930, #33985 ),
 ( #6169, #11705, #18710, #15631, #37638, #8623, #40129, #2491, #24694, #27576, #11909, #5759, #18299 ),
 ( #9036, #2699, #15217, #37244, #38259, #3714, #31695, #19538, #812, #35206, #34805, #12738, #10255 ),
 ( #13344, #16240, #28809, #25513, #10056, #35603, #32118, #19929, #32507, #6582, #15836, #3512, #19128 ),
 ( #613, #38657, #10454, #29207, #29008, #411, #13153, #25317, #1019, #25715, #22238, #38059, #22638 ),
 ( #28392, #23036, #12950, #3921, #25918, #37848, #7372, #38453, #16034, #28602, #16434, #13551, #22836 ),
 ( #35405, #200, #7178, #9653, #19737, #26127, #9861, #32311, #6977, #4108, #22435, #35005, #6779 ),
 ( #16624, #19333, #31903, #39258, #10653, #39457, #11246, #17419, #33103, #14344, #2025, #8158, #7576 ),
 ( #20519, #7968, #1227, #4506, #4888, #10852, #17028, #30004, #39665, #36188, #20730, #33315, #36386 ),
 ( #14541, #4695, #26915, #13761, #1418, #5095, #29603, #26721, #39053, #23429, #29801, #11049, #32905 ),
 ( #1822, #23810, #23624, #23232, #26325, #17628, #38862, #30208, #17227, #1613, #13954, #27115, #24015 ),
 ( #8368, #20940, #35798, #4307, #32711, #20129, #26520, #14148, #11449, #36591, #16829, #29413, #35994 ),
 ( #7775, #20323, #34499, #39877, #15532, #11654, #13053, #27317, #9553, #36790, #12443, #311, #33526 ),
 ( #31600, #33720, #8575, #25416, #19038, #28089, #28291, #18042, #28499, #2443, #9964, #9764, #25010 ),
 ( #3423, #31803, #37957, #21154, #28707, #22136, #37748, #30417, #5499, #34710, #40640, #30635, #6486 ),
 ( #12848, #34914, #37549, #9344, #19237, #520, #15739, #111, #21925, #5297, #22344, #3617, #6273 ),
 ( #17834, #2224, #14746, #25218, #18821, #31394, #24229, #6689, #16145, #25615, #3223, #12644, #38158 ),
 ( #15934, #4208, #1519, #38767, #26627, #39161, #13253, #22545, #10155, #715, #32216, #10367, #4605 ),
 ( #35903, #35704, #7079, #22944, #32013, #7684, #35506, #28909, #4018, #25822, #14052, #16338, #10563 ),
 ( #919, #29516, #35107, #16536, #20037, #22744, #38359, #13864, #7480, #29113, #16728, #19645, #16938 ),
 ( #6885, #38959, #13454, #4413, #19438, #20233, #38557, #13663, #17134, #7278, #19842, #32618, #3821 ),
 ( #29314, #26026, #32817, #35309, #32413, #1130, #26233, #1325, #23137, #26432, #10755, #23334, #29709 ),
 ( #2131, #39987, #15071, #18153, #30323, #17734, #27221, #11556, #2337, #5203, #17330, #5406, #17945 ),
 ( #24129, #11156, #23727, #10956, #7881, #36901, #23920, #29908, #23540, #5613, #8068, #14649, #21058 ),
 ( #2545, #33630, #1723, #39366, #36694, #8678, #8475, #33832, #30528, #30741, #14857, #20431, #39784 ),
 ( #36293, #27427, #11758, #24337, #14253, #27627, #36105, #21260, #36496, #33010, #20629, #4799, #11354 ),
 ( #26825, #33216, #5001, #17526, #30121, #1933, #14454, #27025, #39570, #8267, #20838, #33433, #6638 ) ),
 .UNSPECIFIED., .F., .F., .F.,
 ( 4, 3, 3, 3, 3, 3, 3, 3, 3, 3, 3, 3, 3, 3, 3, 3, 3, 3, 3, 3, 4 ),
 ( 4, 3, 3, 3, 4 ),
 ( 0.01398653888977024161, 0.01402123637946461540, 0.01403858512431180317, 0.01405593386915899093, 0.01412532884854774198, 0.01426411880732524062, 0.01454169872488023790, 0.01509685855999023593, 0.01620717823021022852, 0.01676233806532022655, 0.01731749790043022458, 0.01787265773554021914, 0.01842781757065021717, 0.01953813724087020975, 0.02064845691109020581, 0.02175877658131019840, 0.02231393641642019643, 0.02259151633397519371, 0.02273030629275269235, 0.02279970127214143993, 0.02286909625153019099 ),
 ( 0.000000000000000000, 0.2500000000000000000, 0.5000000000000000000, 0.7500000000000000000, 1.000000000000000000 ),
 .UNSPECIFIED. ) ;
#9153=CARTESIAN_POINT ( 'NONE',  ( 21.85643539959773207, -8.152057848754798997, -9.377623736650162911 ) ) ;
#9155=CARTESIAN_POINT ( 'NONE',  ( -74.65391122663345413, 7.539060228346531112, 9.329047404371412000 ) ) ;
#9158=CARTESIAN_POINT ( 'NONE',  ( -70.92837670882107659, -65.19654454972992141, -6.000000000000002665 ) ) ;
#9161=VECTOR ( 'NONE', #17485, 1000.000000000000000 ) ;
#9162=CARTESIAN_POINT ( 'NONE',  ( 32.88580308198496738, -3.566010387612386090, -5.242313469937768033 ) ) ;
#9163=CARTESIAN_POINT ( 'NONE',  ( 37.11022902811986768, -2.403443262945340830, -5.951558886896759937 ) ) ;
#9171=CARTESIAN_POINT ( 'NONE',  ( 17.21125213350858374, 14.40030432582220321, -2.500000000000000000 ) ) ;
#9172=CARTESIAN_POINT ( 'NONE',  ( 22.07014027993533745, 0.3234589711692046343, -7.440383244949039465 ) ) ;
#9173=CARTESIAN_POINT ( 'NONE',  ( 36.58489777812268784, -1.843467954662745711, -5.775056006311750423 ) ) ;
#9174=CARTESIAN_POINT ( 'NONE',  ( 24.50653798433103248, 2.969344662950985203, -3.630665793498612626 ) ) ;
#9177=CARTESIAN_POINT ( 'NONE',  ( 34.12768836152103802, -3.289258482637194891, 5.532849168731702960 ) ) ;
#9181=CARTESIAN_POINT ( 'NONE',  ( 87.20660408302002509, 0.2574974038930863407, -5.635807106906071340 ) ) ;
#9182=CARTESIAN_POINT ( 'NONE',  ( -70.92837670882201451, -21.78299143689573469, 6.000000000001379341 ) ) ;
#9183=CARTESIAN_POINT ( 'NONE',  ( 21.63111991302532289, 6.952063906928881210, 2.990424737892750429 ) ) ;
#9185=CARTESIAN_POINT ( 'NONE',  ( 24.71424333793793693, 2.641769286553297125, 3.922768386337302626 ) ) ;
#9195=ORIENTED_EDGE ( 'NONE', *, *, #15997, .T. ) ;
#9200=CARTESIAN_POINT ( 'NONE',  ( 33.89869710337333686, -5.476906865792886769, -0.08692379071555116077 ) ) ;
#9201=CARTESIAN_POINT ( 'NONE',  ( 23.14461240764244110, 3.993051640458494589, -3.167054870709993697 ) ) ;
#9206=CARTESIAN_POINT ( 'NONE',  ( -77.88159744744395141, -5.098111721919734940, -7.193586285049241802 ) ) ;
#9209=CARTESIAN_POINT ( 'NONE',  ( 87.30284416890829391, -1.044652313481390760, -5.185858056390752147 ) ) ;
#9217=CARTESIAN_POINT ( 'NONE',  ( 26.27924180621979033, -3.292740819196297686, -4.154355880966675407 ) ) ;
#9221=CARTESIAN_POINT ( 'NONE',  ( 32.77968338845805363, -0.9315752336664611111, 5.322460391044158357 ) ) ;
#9222=DIRECTION ( 'NONE',  ( 1.000000000000000000, 0.000000000000000000, 0.000000000000000000 ) ) ;
#9226=CARTESIAN_POINT ( 'NONE',  ( 18.75851303975696993, -2.772082833101076282, 3.134117654843073364 ) ) ;
#9227=CARTESIAN_POINT ( 'NONE',  ( -12.99139449055068241, -10.90558813203967148, -6.000000000000000000 ) ) ;
#9229=EDGE_LOOP ( 'NONE', ( #20121, #22176 ) ) ;
#9239=CARTESIAN_POINT ( 'NONE',  ( 24.54955273022989104, 2.736081411429597487, 3.876714146131560401 ) ) ;
#9240=CARTESIAN_POINT ( 'NONE',  ( 36.08394752551300400, -1.509676803322822503, 5.633451637947094248 ) ) ;
#9245=CARTESIAN_POINT ( 'NONE',  ( -69.95461280117120850, -0.5204835624159770413, 5.920672442023852788 ) ) ;
#9250=CARTESIAN_POINT ( 'NONE',  ( 22.04453315957904991, 3.307593561896943868, -4.656839850646330881 ) ) ;
#9252=CARTESIAN_POINT ( 'NONE',  ( 21.85643539959777826, -3.868027658932458479, -14.06783426539529458 ) ) ;
#9253=CARTESIAN_POINT ( 'NONE',  ( 17.12093179650376129, 14.48834468576525047, 3.790908043361841617 ) ) ;
#9258=CARTESIAN_POINT ( 'NONE',  ( 87.73528170195316989, -0.1907079786014589107, -4.255344914058586170 ) ) ;
#9259=ORIENTED_EDGE ( 'NONE', *, *, #19722, .T. ) ;
#9262=CARTESIAN_POINT ( 'NONE',  ( 21.52115149856448539, -2.719794669569747469, 3.565294201003603280 ) ) ;
#9263=CARTESIAN_POINT ( 'NONE',  ( 21.58862418887968460, 7.202556094215188054, 2.923978954502209682 ) ) ;
#9264=CARTESIAN_POINT ( 'NONE',  ( 36.78955161406895513, -3.042595920340447346, -5.948297306680297325 ) ) ;
#9266=CARTESIAN_POINT ( 'NONE',  ( 22.01622206693788897, 4.835086392017111656, 3.641232820207879417 ) ) ;
#9272=EDGE_LOOP ( 'NONE', ( #28139, #19471, #19436, #14663 ) ) ;
#9273=CARTESIAN_POINT ( 'NONE',  ( 34.63594631419880443, -0.7840636577548021346, 5.277534085818968990 ) ) ;
#9280=CARTESIAN_POINT ( 'NONE',  ( -76.25573767795857805, -5.662030444549658981, -8.470992006596512525 ) ) ;
#9285=CARTESIAN_POINT ( 'NONE',  ( 21.84668416186902817, 5.868252050249999741, 3.176222544669724090 ) ) ;
#9295=CARTESIAN_POINT ( 'NONE',  ( 17.88216549226283192, 8.679122384522569789, -2.924350684386651356 ) ) ;
#9306=CARTESIAN_POINT ( 'NONE',  ( 29.20850709934801159, 2.242166301403143880, -0.5075834600922535245 ) ) ;
#9310=CARTESIAN_POINT ( 'NONE',  ( 26.72022203379254890, 0.9438563279275373752, -4.381701199652399126 ) ) ;
#9315=DIRECTION ( 'NONE',  ( -0.000000000000000000, -0.000000000000000000, -1.000000000000000000 ) ) ;
#9316=CARTESIAN_POINT ( 'NONE',  ( 25.69802509246645172, 2.595865368573306409, -3.649276983290203447 ) ) ;
#9318=CARTESIAN_POINT ( 'NONE',  ( 32.22182423589296008, -3.776180706330447112, 4.844886202978563539 ) ) ;
#9324=EDGE_CURVE ( 'NONE', #28414, #5730, #9369, .T. ) ;
#9326=DIRECTION ( 'NONE',  ( 0.000000000000000000, -0.000000000000000000, -1.000000000000000000 ) ) ;
#9334=EDGE_CURVE ( 'NONE', #36858, #17221, #13705, .T. ) ;
#9338=VERTEX_POINT ( 'NONE', #35531 ) ;
#9340=CARTESIAN_POINT ( 'NONE',  ( 21.82753364412623043, 5.984910655522465817, 3.124155445945005383 ) ) ;
#9344=CARTESIAN_POINT ( 'NONE',  ( 25.35072175385260707, 0.7578666051937779091, 4.606083722016952819 ) ) ;
#9352=CARTESIAN_POINT ( 'NONE',  ( 21.85643539959778536, -7.083161344002194326, -10.43125315386002860 ) ) ;
#9355=CARTESIAN_POINT ( 'NONE',  ( -73.66952994497191298, 5.999622647709867529, 9.674874949366538246 ) ) ;
#9356=CARTESIAN_POINT ( 'NONE',  ( 36.07013428979532677, -3.674804590447603658, 5.686060082110223846 ) ) ;
#9361=CARTESIAN_POINT ( 'NONE',  ( 37.10469866122600990, -3.126968154306207115, -5.976136871014097629 ) ) ;
#9369=LINE ( 'NONE', #30610, #20399 ) ;
#9370=CARTESIAN_POINT ( 'NONE',  ( 25.85236391290114710, 0.9906390358642165328, -4.433872417139598454 ) ) ;
#9372=CARTESIAN_POINT ( 'NONE',  ( 24.72152762843544593, 2.637715318777088758, -3.924694980037289227 ) ) ;
#9375=CARTESIAN_POINT ( 'NONE',  ( 37.02720035777826268, -2.689369851865129224, 5.985388140692741388 ) ) ;
#9379=CARTESIAN_POINT ( 'NONE',  ( 86.75210013534866960, -0.2795847087395720298, -5.842668109216860195 ) ) ;
#9381=CARTESIAN_POINT ( 'NONE',  ( 35.97396611704095193, -3.154454633011662068, -5.821005464859283940 ) ) ;
#9383=CARTESIAN_POINT ( 'NONE',  ( 25.86470230964163619, 2.040241906511436998, 4.181023058831703665 ) ) ;
#9384=CARTESIAN_POINT ( 'NONE',  ( -70.66582705103253659, -21.75666374495045474, 5.995465708869195609 ) ) ;
#9399=CARTESIAN_POINT ( 'NONE',  ( -71.05882934118332628, -21.78299143688722239, 9.999999999999980460 ) ) ;
#9401=CARTESIAN_POINT ( 'NONE',  ( 23.14002857363139753, 4.041596889213259658, -3.091365628204219007 ) ) ;
#9408=CARTESIAN_POINT ( 'NONE',  ( 85.51010218477300384, 1.603708918324822541, 5.381112834985590787 ) ) ;
#9413=VERTEX_POINT ( 'NONE', #3643 ) ;
#9414=EDGE_CURVE ( 'NONE', #24982, #36231, #21716, .T. ) ;
#9415=DIRECTION ( 'NONE',  ( 0.000000000000000000, 0.000000000000000000, 1.000000000000000000 ) ) ;
#9418=CARTESIAN_POINT ( 'NONE',  ( 85.57589026689105083, 1.015016660241817359, 5.782947816673639885 ) ) ;
#9419=ORIENTED_EDGE ( 'NONE', *, *, #11873, .F. ) ;
#9420=CARTESIAN_POINT ( 'NONE',  ( 36.63317992190049210, -3.078756398745077227, 5.923891722253738834 ) ) ;
#9422=CARTESIAN_POINT ( 'NONE',  ( 87.79476240240137486, -0.2575195244695515639, -3.704994186184041194 ) ) ;
#9429=ORIENTED_EDGE ( 'NONE', *, *, #19381, .T. ) ;
#9430=CARTESIAN_POINT ( 'NONE',  ( 26.41406563113697104, -4.824719389755182775, -3.358585079837815623 ) ) ;
#9433=LINE ( 'NONE', #27013, #12323 ) ;
#9434=AXIS2_PLACEMENT_3D ( 'NONE', #29581, #6956, #13739 ) ;
#9441=CARTESIAN_POINT ( 'NONE',  ( 35.96670479602093451, -3.154862874710424592, 5.819872160098396918 ) ) ;
#9443=CARTESIAN_POINT ( 'NONE',  ( 23.11908726903853406, 2.858206452918472529, 4.238382280009368230 ) ) ;
#9449=DIRECTION ( 'NONE',  ( 0.000000000000000000, 0.000000000000000000, -1.000000000000000000 ) ) ;
#9450=CARTESIAN_POINT ( 'NONE',  ( 86.14814696281284512, 1.592037090359822882, -4.564681075395820464 ) ) ;
#9453=CARTESIAN_POINT ( 'NONE',  ( 23.47264373427338313, 3.111346557503597676, -3.866181119602032368 ) ) ;
#9455=CARTESIAN_POINT ( 'NONE',  ( 21.85643539959778536, -9.383538770078029501, -13.42257110913290141 ) ) ;
#9460=CARTESIAN_POINT ( 'NONE',  ( 88.11777217834651310, -0.6203394357796320202, -3.242821525125987758 ) ) ;
#9462=CARTESIAN_POINT ( 'NONE',  ( 14.61802080322508424, 12.62870316935584647, 2.500000000000000000 ) ) ;
#9463=CARTESIAN_POINT ( 'NONE',  ( 33.94289416639321644, -3.572325359806576284, 5.436201825232916285 ) ) ;
#9465=CARTESIAN_POINT ( 'NONE',  ( 34.77293049090385324, -3.164284130107499315, -5.633554808244025658 ) ) ;
#9467=LINE ( 'NONE', #28419, #27902 ) ;
#9470=CARTESIAN_POINT ( 'NONE',  ( 8.290806648384990041, -33.63722727088462250, -2.499999999999998668 ) ) ;
#9472=ORIENTED_EDGE ( 'NONE', *, *, #11089, .T. ) ;
#9473=CARTESIAN_POINT ( 'NONE',  ( 37.21105169095337573, -2.744044523102963318, 6.000898145687354912 ) ) ;
#9478=CARTESIAN_POINT ( 'NONE',  ( 86.59338513520690128, -0.7688615754554688486, -5.609335628161745468 ) ) ;
#9482=CARTESIAN_POINT ( 'NONE',  ( -80.16840965959801224, -6.651026884041253417, -3.846849152753851087 ) ) ;
#9483=EDGE_CURVE ( 'NONE', #34557, #28485, #23039, .T. ) ;
#9485=DIRECTION ( 'NONE',  ( 0.000000000000000000, 0.000000000000000000, 1.000000000000000000 ) ) ;
#9491=CARTESIAN_POINT ( 'NONE',  ( 22.89740935448892500, 4.239003498654196456, 3.174338064556351924 ) ) ;
#9497=ORIENTED_EDGE ( 'NONE', *, *, #20088, .T. ) ;
#9500=CARTESIAN_POINT ( 'NONE',  ( 14.64821644803149425, 12.77550546983412438, -2.492606463805589811 ) ) ;
#9503=CARTESIAN_POINT ( 'NONE',  ( 19.21949373037735853, 7.325913195097914610, -3.173010411643660600 ) ) ;
#9512=DIRECTION ( 'NONE',  ( -0.9880385148181951571, 0.000000000000000000, -0.1542073060391599970 ) ) ;
#9513=CARTESIAN_POINT ( 'NONE',  ( 27.87470673840761037, 2.608020033772324275, -0.5247038454205935620 ) ) ;
#9521=CARTESIAN_POINT ( 'NONE',  ( 34.78019789095738901, -3.716936043298515457, -5.478546665663536430 ) ) ;
#9524=CARTESIAN_POINT ( 'NONE',  ( 14.74700808699402899, -4.436407246566614226, -2.508025288350517634 ) ) ;
#9525=DIRECTION ( 'NONE',  ( 0.000000000000000000, 1.000000000000000000, 0.000000000000000000 ) ) ;
#9543=CARTESIAN_POINT ( 'NONE',  ( 22.02762008288383200, 3.976027453218988317, 4.186289093362514535 ) ) ;
#9548=CARTESIAN_POINT ( 'NONE',  ( 21.98934069226735133, 5.611891575985531233, 3.092273232226271595 ) ) ;
#9549=DIRECTION ( 'NONE',  ( 0.9982280052159038242, 0.000000000000000000, 0.05950503846463438273 ) ) ;
#9553=CARTESIAN_POINT ( 'NONE',  ( 22.71567147354432237, 0.3624905230350064511, 6.349376209889807221 ) ) ;
#9557=ORIENTED_EDGE ( 'NONE', *, *, #39077, .F. ) ;
#9564=CARTESIAN_POINT ( 'NONE',  ( 21.85643539959776049, -3.145688729744653411, 12.47482453294728266 ) ) ;
#9567=CARTESIAN_POINT ( 'NONE',  ( -75.35262966362313364, 8.291683080040980869, 9.005052742938818966 ) ) ;
#9568=CARTESIAN_POINT ( 'NONE',  ( 36.07971702944216474, -3.672696443019492829, 5.688510560309873121 ) ) ;
#9573=CARTESIAN_POINT ( 'NONE',  ( 36.68636550425712528, -1.913427295981317888, -5.802400637960247742 ) ) ;
#9576=CARTESIAN_POINT ( 'NONE',  ( 22.37810747204872897, 5.219580669678665963, 3.555984268806748894 ) ) ;
#9578=CARTESIAN_POINT ( 'NONE',  ( -7.890026461918810519, -29.56993018339340651, 6.000000000000000000 ) ) ;
#9583=CARTESIAN_POINT ( 'NONE',  ( 24.35854945548016914, 1.282877579546743307, -4.712861751322592774 ) ) ;
#9584=CARTESIAN_POINT ( 'NONE',  ( 31.38981853733673688, -3.758192538165083807, -4.681675008679978767 ) ) ;
#9586=EDGE_LOOP ( 'NONE', ( #21719, #25247 ) ) ;
#9588=CARTESIAN_POINT ( 'NONE',  ( 29.13956619203430520, 0.4692469261591867280, 4.754332065975193977 ) ) ;
#9590=VECTOR ( 'NONE', #18599, 1000.000000000000000 ) ;
#9591=CARTESIAN_POINT ( 'NONE',  ( 85.73014479007146349, 1.298542115207370173, 5.666065989068760800 ) ) ;
#9593=CARTESIAN_POINT ( 'NONE',  ( 21.67220405017981122, 6.675115239655725397, 3.070808856021292499 ) ) ;
#9595=CARTESIAN_POINT ( 'NONE',  ( 24.60366954196197042, 2.981655850978834899, 3.555329962009686540 ) ) ;
#9599=VERTEX_POINT ( 'NONE', #13692 ) ;
#9602=ORIENTED_EDGE ( 'NONE', *, *, #15605, .F. ) ;
#9613=CARTESIAN_POINT ( 'NONE',  ( 24.05436622899220822, 3.340017053445958783, -3.241057297173068452 ) ) ;
#9619=CARTESIAN_POINT ( 'NONE',  ( -79.08083519856748467, -5.497992658161905410, -5.845328771210035690 ) ) ;
#9622=CARTESIAN_POINT ( 'NONE',  ( 87.51701825761838904, -2.015745416966476800, -3.511549023785576651 ) ) ;
#9626=DIRECTION ( 'NONE',  ( -2.699830798738917390E-13, 1.000000000000000000, 0.000000000000000000 ) ) ;
#9628=AXIS2_PLACEMENT_3D ( 'NONE', #24300, #3482, #11725 ) ;
#9634=CARTESIAN_POINT ( 'NONE',  ( 85.58015388280458069, 1.007655178167426335, 5.787227695588894605 ) ) ;
#9637=CARTESIAN_POINT ( 'NONE',  ( 36.14155268336735816, -3.142484588683069902, 5.847161401630891042 ) ) ;
#9638=CARTESIAN_POINT ( 'NONE',  ( 87.09859342968812257, 0.5244505078549105415, -5.068689133590885909 ) ) ;
#9641=CARTESIAN_POINT ( 'NONE',  ( 14.75078054601031674, -5.140699092989589047, 2.499999999999999556 ) ) ;
#9647=CARTESIAN_POINT ( 'NONE',  ( -80.55887061931086635, -6.632148677064343190, 2.726002644713694245 ) ) ;
#9651=CARTESIAN_POINT ( 'NONE',  ( 36.06236019073843835, -3.149134278961357225, 5.834801497878530085 ) ) ;
#9653=CARTESIAN_POINT ( 'NONE',  ( 24.64370639163859522, 1.605171026338595430, 4.497401421240313724 ) ) ;
#9654=CARTESIAN_POINT ( 'NONE',  ( 37.20488407139969667, -2.771826426831375034, 5.999999980036296421 ) ) ;
#9665=CARTESIAN_POINT ( 'NONE',  ( 24.13014922190525624, 2.944621410230606529, -3.777319215821884235 ) ) ;
#9667=EDGE_CURVE ( 'NONE', #9413, #19825, #38040, .T. ) ;
#9669=CARTESIAN_POINT ( 'NONE',  ( 21.85643539959774273, 9.172641120068929510, -1.679843024921975347 ) ) ;
#9670=EDGE_CURVE ( 'NONE', #33153, #28854, #21346, .T. ) ;
#9674=CARTESIAN_POINT ( 'NONE',  ( 87.15505355144220800, 0.4610318193416703680, -5.246243280819175681 ) ) ;
#9677=CARTESIAN_POINT ( 'NONE',  ( 14.67325355196695646, 12.62073864643243226, 2.499999999998588240 ) ) ;
#9678=CARTESIAN_POINT ( 'NONE',  ( 21.52542566397378820, -2.894605234475977618, 3.543787706140388849 ) ) ;
#9681=CARTESIAN_POINT ( 'NONE',  ( 36.44671748466953431, -2.355057832951331420, -5.894789749312875138 ) ) ;
#9683=CARTESIAN_POINT ( 'NONE',  ( 21.81726414084884169, 5.354314201170920384, 3.565644528639963617 ) ) ;
#9692=CARTESIAN_POINT ( 'NONE',  ( 30.68797926878130866, -2.925629016318143538, 4.995999375113326479 ) ) ;
#9694=CARTESIAN_POINT ( 'NONE',  ( 34.14220566676094393, -3.846217302993689469, 5.236774695382229616 ) ) ;
#9699=ORIENTED_EDGE ( 'NONE', *, *, #23579, .F. ) ;
#9701=CARTESIAN_POINT ( 'NONE',  ( -76.19356073596259193, 10.47839387954511814, -8.503801285675736565 ) ) ;
#9706=CARTESIAN_POINT ( 'NONE',  ( 22.90651681474014012, 4.202743079833220818, 3.210710377858703168 ) ) ;
#9714=CARTESIAN_POINT ( 'NONE',  ( 16.54063652338793133, 10.02979042668312992, -2.737642957281533729 ) ) ;
#9717=VECTOR ( 'NONE', #29031, 1000.000000000000000 ) ;
#9719=VECTOR ( 'NONE', #34543, 1000.000000000000000 ) ;
#9723=FACE_OUTER_BOUND ( 'NONE', #9086, .T. ) ;
#9724=CARTESIAN_POINT ( 'NONE',  ( 19.55994146243534715, 8.628030923317455247, 2.499999999993585575 ) ) ;
#9725=CARTESIAN_POINT ( 'NONE',  ( 27.31903677934867147, 0.4900422023718347675, -5.740875207198388175 ) ) ;
#9735=CARTESIAN_POINT ( 'NONE',  ( 35.56295975436646017, -1.640838707923856443, -5.744612369613007807 ) ) ;
#9742=CARTESIAN_POINT ( 'NONE',  ( -81.63024932266884548, 10.48199852196216497, 2.292792362136173434 ) ) ;
#9746=ORIENTED_EDGE ( 'NONE', *, *, #9334, .T. ) ;
#9752=LINE ( 'NONE', #13240, #36429 ) ;
#9753=CARTESIAN_POINT ( 'NONE',  ( 22.84784676164604278, 3.199131945760815832, 4.124430016485445272 ) ) ;
#9757=CARTESIAN_POINT ( 'NONE',  ( 24.06683628570359446, 3.348910172779726135, 3.206004284675357141 ) ) ;
#9764=CARTESIAN_POINT ( 'NONE',  ( 21.83335788848096115, 0.3052388310511004454, 8.127432559144740054 ) ) ;
#9770=CARTESIAN_POINT ( 'NONE',  ( 22.73811350958456501, -4.924115162416450531, 6.814090253401713149 ) ) ;
#9773=CARTESIAN_POINT ( 'NONE',  ( -73.51040120057371041, 5.657262173908669034, 9.719076197244223891 ) ) ;
#9775=ORIENTED_EDGE ( 'NONE', *, *, #34337, .T. ) ;
#9780=CARTESIAN_POINT ( 'NONE',  ( 33.44745999691134131, -3.711946420718001516, -5.220912322284510410 ) ) ;
#9781=CARTESIAN_POINT ( 'NONE',  ( 35.22195622051280139, -1.045642381572828628, -5.409226251924048157 ) ) ;
#9787=DIRECTION ( 'NONE',  ( 0.000000000000000000, -0.000000000000000000, -1.000000000000000000 ) ) ;
#9788=CARTESIAN_POINT ( 'NONE',  ( 22.81751159329827772, 0.7919312097182544807, -5.980481906966360839 ) ) ;
#9789=CARTESIAN_POINT ( 'NONE',  ( 32.00007467492793012, -3.767639907337460237, -4.802642618328528457 ) ) ;
#9792=ORIENTED_EDGE ( 'NONE', *, *, #4389, .F. ) ;
#9793=ORIENTED_EDGE ( 'NONE', *, *, #17136, .F. ) ;
#9796=CARTESIAN_POINT ( 'NONE',  ( 84.55403409623259847, 2.802886334004389024, 2.719422554281196280 ) ) ;
#9798=CARTESIAN_POINT ( 'NONE',  ( 24.49724481738078197, 2.968026975615160268, 3.636704260287059398 ) ) ;
#9801=CARTESIAN_POINT ( 'NONE',  ( 25.01091298175105848, 3.329590532566609529, -1.936828115965013142 ) ) ;
#9807=CARTESIAN_POINT ( 'NONE',  ( -70.92837670882107659, -45.61702805680359063, 10.00000000000000888 ) ) ;
#9819=CARTESIAN_POINT ( 'NONE',  ( 21.85643539959776760, 8.744094842958308078, -10.51782716378651550 ) ) ;
#9820=CARTESIAN_POINT ( 'NONE',  ( 24.71484882724550758, 3.003952457561420708, -3.426556331288557189 ) ) ;
#9822=CARTESIAN_POINT ( 'NONE',  ( -2.697268050091675118E-17, 3.729367930467589076, 6.000000000000000000 ) ) ;
#9826=CARTESIAN_POINT ( 'NONE',  ( -80.34590231409514161, -5.681217598735836205, -3.387305046538306552 ) ) ;
#9827=EDGE_CURVE ( 'NONE', #5466, #22987, #5152, .T. ) ;
#9833=ORIENTED_EDGE ( 'NONE', *, *, #11414, .T. ) ;
#9835=CARTESIAN_POINT ( 'NONE',  ( 20.26402972545001191, -7.228810192355688002, -2.500000000000000000 ) ) ;
#9837=B_SPLINE_CURVE_WITH_KNOTS ( 'NONE', 3,
 ( #4465, #32269, #16783, #38412, #10210, #26283, #22792, #38817, #35361, #10609, #7133, #19693, #13909, #26079, #1379, #1181, #32665, #21114, #30590, #1773, #14922, #40040, #5463, #30166, #21317, #36547, #33891 ),
 .UNSPECIFIED., .F., .F.,
 ( 4, 1, 2, 2, 1, 1, 1, 1, 1, 2, 2, 1, 1, 1, 1, 2, 2, 1, 4 ),
 ( 0.000000000000000000, 0.2324235260548973003, 0.2469499964333282671, 0.2614764668117592894, 0.2905294075686204458, 0.3486352890823428141, 0.4648470521097886055, 0.4938999928666482075, 0.4975316104612538815, 0.4993474192585585780, 0.5011632280558633301, 0.5084264632450831156, 0.5229529336235230197, 0.5810588151372841903, 0.6972705781648077528, 0.7263235189216886711, 0.7553764596785694785, 0.8134823411923304270, 0.9296941042198524352 ),
 .UNSPECIFIED. ) ;
#9839=FACE_OUTER_BOUND ( 'NONE', #31241, .T. ) ;
#9842=CARTESIAN_POINT ( 'NONE',  ( 30.51504204651931929, -0.1407231940035871265, 4.969008339076835590 ) ) ;
#9844=CARTESIAN_POINT ( 'NONE',  ( 87.61456772748933020, -0.05511631305283664489, -4.124113870075747812 ) ) ;
#9849=CARTESIAN_POINT ( 'NONE',  ( -70.44490529243154242, -45.69367636896786422, 9.988720588804540057 ) ) ;
#9854=CARTESIAN_POINT ( 'NONE',  ( -74.62920569612701627, -4.460155050320008918, 9.295740457114378685 ) ) ;
#9861=CARTESIAN_POINT ( 'NONE',  ( 23.51444095708766824, 1.310649503969850915, 5.121933516958420363 ) ) ;
#9872=CARTESIAN_POINT ( 'NONE',  ( 23.42095263414284290, 3.374540284680194624, -3.661182053110778600 ) ) ;
#9876=CARTESIAN_POINT ( 'NONE',  ( 21.85643539959776760, 7.145415623174192987, -7.905327125498018859 ) ) ;
#9879=CARTESIAN_POINT ( 'NONE',  ( 86.00054146471580907, 0.2529338399765344580, 5.999804812770356932 ) ) ;
#9881=CARTESIAN_POINT ( 'NONE',  ( 87.43313723349395161, -0.009410480739497543642, 5.495402557179364322 ) ) ;
#9884=CARTESIAN_POINT ( 'NONE',  ( 14.82998033694128459, -4.532293462924823935, 2.514727759383232897 ) ) ;
#9885=CARTESIAN_POINT ( 'NONE',  ( 36.42070800990175172, -3.114118155843566438, -5.890730341733725339 ) ) ;
#9888=CARTESIAN_POINT ( 'NONE',  ( 30.57577539112692477, -3.618309187433789376, -4.738484246135796774 ) ) ;
#9892=CARTESIAN_POINT ( 'NONE',  ( 28.18787290715265215, -3.182640706483542470, 4.605797312080136763 ) ) ;
#9895=CARTESIAN_POINT ( 'NONE',  ( 20.91846109042669610, 4.580160148488255700, 2.658159626579862156 ) ) ;
#9896=CARTESIAN_POINT ( 'NONE',  ( -2.697268050091675118E-17, 3.729367930467589076, 6.000000000000000000 ) ) ;
#9903=DIRECTION ( 'NONE',  ( -1.000000000000000000, 0.000000000000000000, 0.000000000000000000 ) ) ;
#9908=CARTESIAN_POINT ( 'NONE',  ( 21.86792300497991803, 5.743675277279487901, 3.228481761958482021 ) ) ;
#9917=CARTESIAN_POINT ( 'NONE',  ( 17.01838609035475613, 9.182891198947618960, -2.862528759259550970 ) ) ;
#9926=CARTESIAN_POINT ( 'NONE',  ( 15.78341758396470418, 8.012724437683271361, 3.484800230006450228 ) ) ;
#9927=CARTESIAN_POINT ( 'NONE',  ( 29.24730582455742578, -0.4004845594861357605, -5.905559009470326970 ) ) ;
#9934=CARTESIAN_POINT ( 'NONE',  ( 35.34375719191214671, -3.571401254346052045, -5.666764866774185450 ) ) ;
#9938=CARTESIAN_POINT ( 'NONE',  ( 21.88224095673515635, -13.29272450212527446, -2.499999999999999556 ) ) ;
#9939=CARTESIAN_POINT ( 'NONE',  ( 22.00316676826400908, -11.76202948577872753, 2.500000000000000000 ) ) ;
#9940=LINE ( 'NONE', #3405, #5186 ) ;
#9943=ORIENTED_EDGE ( 'NONE', *, *, #35263, .T. ) ;
#9949=CARTESIAN_POINT ( 'NONE',  ( 30.67349724481533002, -3.593355625737403525, 4.777428303402127874 ) ) ;
#9950=CARTESIAN_POINT ( 'NONE',  ( 24.00583079004835341, 2.820796528902969502, 3.912411818918270168 ) ) ;
#9951=CARTESIAN_POINT ( 'NONE',  ( 8.290806648384990041, -35.94265729135299381, 6.000000000000000000 ) ) ;
#9955=CARTESIAN_POINT ( 'NONE',  ( 21.83036068403676921, 5.963027752284762784, 3.135844384568250653 ) ) ;
#9964=CARTESIAN_POINT ( 'NONE',  ( 22.04975653352279963, 0.2919591322827700397, 7.506304445313716656 ) ) ;
#9968=CARTESIAN_POINT ( 'NONE',  ( 33.45716606812183613, -3.829385970599605393, -5.093809925484540813 ) ) ;
#9972=CARTESIAN_POINT ( 'NONE',  ( 24.13449073166137637, 1.731319574254092997, -6.231442870084249464 ) ) ;
#9974=VERTEX_POINT ( 'NONE', #32793 ) ;
#9975=CARTESIAN_POINT ( 'NONE',  ( -75.33383759686411452, -3.421339376598665716, 9.017346126309083942 ) ) ;
#9980=CARTESIAN_POINT ( 'NONE',  ( 32.02031732332363845, -3.752465789452563261, -4.808771302114207558 ) ) ;
#9981=CARTESIAN_POINT ( 'NONE',  ( 36.71895965078132917, -3.458220008152968372, -5.860798406330455457 ) ) ;
#9983=CARTESIAN_POINT ( 'NONE',  ( 17.44269447096448644, 8.925452895480308513, 2.905853932266882378 ) ) ;
#9988=CARTESIAN_POINT ( 'NONE',  ( 25.21793605145752792, 1.560386695300661319, -4.376291279302483517 ) ) ;
#9990=CARTESIAN_POINT ( 'NONE',  ( 29.65754893815654825, 1.153748204478383999, -4.260714825772614844 ) ) ;
#9991=CARTESIAN_POINT ( 'NONE',  ( 15.70794464876099816, 12.77956130087500952, -2.500000000000005329 ) ) ;
#9995=CARTESIAN_POINT ( 'NONE',  ( 84.91553621511910421, 2.364970790127210787, 4.120477167815592701 ) ) ;
#9997=CARTESIAN_POINT ( 'NONE',  ( 26.60586539650099169, 1.632482450356405268, 4.331819419614522104 ) ) ;
#10010=CARTESIAN_POINT ( 'NONE',  ( 28.37767182338955507, -4.101067068145935579, 4.014301156824140016 ) ) ;
#10012=CARTESIAN_POINT ( 'NONE',  ( 21.85643539959777826, -13.51165962708896728, -8.254727072381385256 ) ) ;
#10013=CARTESIAN_POINT ( 'NONE',  ( 23.73324195583390761, 3.546141233244914925, -3.227706410081386146 ) ) ;
#10017=VERTEX_POINT ( 'NONE', #38537 ) ;
#10020=CARTESIAN_POINT ( 'NONE',  ( -73.51024996325405425, -0.7972945005789436879, -9.719117299233273499 ) ) ;
#10022=DIRECTION ( 'NONE',  ( 1.000000000000000000, 0.000000000000000000, 0.000000000000000000 ) ) ;
#10024=CARTESIAN_POINT ( 'NONE',  ( 86.09116122586011954, 0.08319669091220074919, -6.006182420748226392 ) ) ;
#10027=CARTESIAN_POINT ( 'NONE',  ( 86.43572624768425783, -0.5192074800720990480, -5.777013305174518720 ) ) ;
#10028=CARTESIAN_POINT ( 'NONE',  ( 33.62470413278058601, -1.226591137072588600, 5.454346315099659392 ) ) ;
#10037=CARTESIAN_POINT ( 'NONE',  ( 36.42090402691821538, -3.114971261605032904, 5.890760934929827997 ) ) ;
#10042=CARTESIAN_POINT ( 'NONE',  ( 86.68816865751659861, 0.9854590918928021193, 5.166709667929270999 ) ) ;
#10047=VECTOR ( 'NONE', #32448, 1000.000000000000000 ) ;
#10051=CARTESIAN_POINT ( 'NONE',  ( -73.09553771626850960, -2.532785756717299108, 9.765145150773129501 ) ) ;
#10056=CARTESIAN_POINT ( 'NONE',  ( 23.90473187725620363, 2.109340586275191942, 4.420426059884545289 ) ) ;
#10061=DIRECTION ( 'NONE',  ( 0.9594800004753906153, 0.2817767355331954326, 0.000000000000000000 ) ) ;
#10064=CARTESIAN_POINT ( 'NONE',  ( 23.44360806831497257, 3.234883382834601750, -3.775111565067499342 ) ) ;
#10065=ORIENTED_EDGE ( 'NONE', *, *, #23203, .F. ) ;
#10068=CARTESIAN_POINT ( 'NONE',  ( 21.85643539959777826, -4.710037025930063237, 11.93878138912534226 ) ) ;
#10069=CARTESIAN_POINT ( 'NONE',  ( 21.85970433026863802, 3.598116536247010444, 3.919871293596266515 ) ) ;
#10073=CARTESIAN_POINT ( 'NONE',  ( 87.79537149936930973, -0.4305974645707495441, -5.064761461465907999 ) ) ;
#10077=CARTESIAN_POINT ( 'NONE',  ( 28.89675923326203488, -2.947373090957444042, 4.716436167749639807 ) ) ;
#10078=CARTESIAN_POINT ( 'NONE',  ( 35.95071194461377928, -2.121207001979848794, 5.817376088847740156 ) ) ;
#10080=CARTESIAN_POINT ( 'NONE',  ( 35.33511053670775937, -3.171501256377859512, -5.721296600767692198 ) ) ;
#10082=CARTESIAN_POINT ( 'NONE',  ( 84.23367565633908782, 2.854638525470858834, 2.083157151739415180 ) ) ;
#10085=CARTESIAN_POINT ( 'NONE',  ( -72.84815947045233031, 2.429809908889422498, 10.96147798754374669 ) ) ;
#10091=CARTESIAN_POINT ( 'NONE',  ( 32.00410610819579915, -3.635846591686252793, 4.956023177179895711 ) ) ;
#10094=CARTESIAN_POINT ( 'NONE',  ( 27.81484381033608599, 1.842735594674395516, 3.911111060978480936 ) ) ;
#10109=CARTESIAN_POINT ( 'NONE',  ( 16.29644454726526348, 9.829709983188696043, -2.749852321238235753 ) ) ;
#10112=EDGE_CURVE ( 'NONE', #218, #28242, #6627, .T. ) ;
#10113=LINE ( 'NONE', #3975, #448 ) ;
#10117=CARTESIAN_POINT ( 'NONE',  ( 29.97903609306309747, -3.796949753938318128, 3.982659670407546759 ) ) ;
#10126=CARTESIAN_POINT ( 'NONE',  ( 36.34374669389929835, -1.915861758104068224, -5.836669621121017393 ) ) ;
#10131=CARTESIAN_POINT ( 'NONE',  ( -76.12810195176366790, 8.940663570071636812, 9.995849007841474787 ) ) ;
#10133=PLANE ( 'NONE',  #10330 ) ;
#10142=CARTESIAN_POINT ( 'NONE',  ( 22.40981647624643713, 3.721157939412742532, 4.045705223971617137 ) ) ;
#10147=CARTESIAN_POINT ( 'NONE',  ( 23.75168596251202402, 3.571076225440265262, 3.154308973096512148 ) ) ;
#10150=CARTESIAN_POINT ( 'NONE',  ( 20.51517429375766355, -3.043394856432828366, 3.333276972429214613 ) ) ;
#10155=CARTESIAN_POINT ( 'NONE',  ( 22.63505186344747244, 0.3020627423357405417, 6.468267501412062082 ) ) ;
#10160=CARTESIAN_POINT ( 'NONE',  ( 8.290806648384990041, 0.000000000000000000, -6.000000000000000000 ) ) ;
#10163=CARTESIAN_POINT ( 'NONE',  ( 25.11223377877777807, -2.893972711065841086, 5.714375009671201155 ) ) ;
#10166=CARTESIAN_POINT ( 'NONE',  ( -79.93950600478302704, -5.593546482839650835, 6.495256196073648347 ) ) ;
#10167=CARTESIAN_POINT ( 'NONE',  ( 22.60277623034728478, 0.2789645760982217282, -6.515020334618169429 ) ) ;
#10173=CARTESIAN_POINT ( 'NONE',  ( -58.92473026143643722, -52.43948302755219260, -2.500000000000000000 ) ) ;
#10174=CARTESIAN_POINT ( 'NONE',  ( 33.68478720806815829, -3.838055986494960159, -5.140077084911478522 ) ) ;
#10176=VECTOR ( 'NONE', #33033, 1000.000000000000000 ) ;
#10178=CARTESIAN_POINT ( 'NONE',  ( 17.18926217949810109, 9.340092606904171646, 2.827706503231969037 ) ) ;
#10186=CARTESIAN_POINT ( 'NONE',  ( 22.50793842622461582, 0.7792813105832565590, -6.394562644212967939 ) ) ;
#10187=CARTESIAN_POINT ( 'NONE',  ( 35.22275699169255603, -1.056573163075043453, -5.416485502172596611 ) ) ;
#10189=DIRECTION ( 'NONE',  ( -0.000000000000000000, -1.000000000000000000, -0.000000000000000000 ) ) ;
#10194=CARTESIAN_POINT ( 'NONE',  ( 88.33724419093491065, -2.316998127210522007, 1.237639510709749091 ) ) ;
#10201=( NAMED_UNIT ( * ) PLANE_ANGLE_UNIT ( ) SI_UNIT ( $, .RADIAN. ) );
#10202=CIRCLE ( 'NONE', #10835, 7.744449365083023729 ) ;
#10210=CARTESIAN_POINT ( 'NONE',  ( 25.83360062294675075, 1.871733103193846448, 4.238356183839651514 ) ) ;
#10214=CARTESIAN_POINT ( 'NONE',  ( 21.85643539959776049, -15.24219007203948983, -1.854490019360333086 ) ) ;
#10216=CARTESIAN_POINT ( 'NONE',  ( 22.39823815405979701, 4.874039138771919077, -3.101746399076472205 ) ) ;
#10222=CARTESIAN_POINT ( 'NONE',  ( -73.23924125533064000, -0.08275262721004308930, -9.788968532873301598 ) ) ;
#10224=DIRECTION ( 'NONE',  ( -0.000000000000000000, 1.000000000000000000, -0.000000000000000000 ) ) ;
#10226=CARTESIAN_POINT ( 'NONE',  ( 85.17103880321602105, 1.638380925414154587, -5.247232096711407223 ) ) ;
#10232=AXIS2_PLACEMENT_3D ( 'NONE', #5193, #36890, #27815 ) ;
#10240=CARTESIAN_POINT ( 'NONE',  ( 33.62807682128043751, -1.230511385543872294, 5.454872704708900066 ) ) ;
#10241=VECTOR ( 'NONE', #21878, 1000.000000000000114 ) ;
#10243=CARTESIAN_POINT ( 'NONE',  ( 86.36291470068610465, 1.350799773688788674, 4.987004148466622766 ) ) ;
#10248=ORIENTED_EDGE ( 'NONE', *, *, #17117, .F. ) ;
#10255=CARTESIAN_POINT ( 'NONE',  ( 21.83945981511907064, 2.416022838233994552, 5.659870449405054238 ) ) ;
#10262=CARTESIAN_POINT ( 'NONE',  ( 85.76750662938394498, 2.019590379147275794, 3.841493691465702298 ) ) ;
#10265=CARTESIAN_POINT ( 'NONE',  ( 23.41724364834474414, 3.428523892220677993, -3.609970445808396544 ) ) ;
#10266=ORIENTED_EDGE ( 'NONE', *, *, #40329, .T. ) ;
#10271=CARTESIAN_POINT ( 'NONE',  ( 21.85643539959779957, 3.623429283794106670, 13.13803316603621241 ) ) ;
#10272=CARTESIAN_POINT ( 'NONE',  ( 20.24823138111575105, 11.68787526792862153, 3.842642712662352800 ) ) ;
#10276=CARTESIAN_POINT ( 'NONE',  ( 84.82990711808488982, 3.023024660489734394, 1.086629044751433293 ) ) ;
#10278=B_SPLINE_CURVE_WITH_KNOTS ( 'NONE', 3,
 ( #15185, #15392, #39899, #28153, #12087, #5729, #40707, #36811, #18267, #14767, #30652, #24875, #40491, #37213, #25083, #30859 ),
 .UNSPECIFIED., .F., .F.,
 ( 4, 2, 2, 2, 2, 2, 2, 4 ),
 ( 0.000000000000000000, 0.0006740595217997351124, 0.001348119043599470225, 0.002696238087198940449, 0.004044357130798413059, 0.005392476174397886970, 0.008088714261596836527, 0.01078495234879578782 ),
 .UNSPECIFIED. ) ;
#10280=CARTESIAN_POINT ( 'NONE',  ( 14.65850939258177554, -5.614383887714384791, 2.494212926738383906 ) ) ;
#10281=CARTESIAN_POINT ( 'NONE',  ( 37.01706860164229340, -2.756673952631257141, 5.983806835110248024 ) ) ;
#10282=CARTESIAN_POINT ( 'NONE',  ( -17.69482985384421880, -29.56993018339339940, 2.500000000000000000 ) ) ;
#10284=CARTESIAN_POINT ( 'NONE',  ( 22.92126275026679494, 2.653310250737696663, -3.783815423649973031 ) ) ;
#10287=CARTESIAN_POINT ( 'NONE',  ( 85.48109816848365483, 1.178641903994587903, 5.687362864452985889 ) ) ;
#10290=CARTESIAN_POINT ( 'NONE',  ( 29.62473861780153683, -3.849278697187920706, 4.318228108797867115 ) ) ;
#10293=CARTESIAN_POINT ( 'NONE',  ( 23.38512868750360596, 3.559325214671839266, 3.095447384079575315 ) ) ;
#10297=CARTESIAN_POINT ( 'NONE',  ( 87.60931828755812489, -2.129004962406701562, 3.117860766101097525 ) ) ;
#10299=ORIENTED_EDGE ( 'NONE', *, *, #27668, .F. ) ;
#10302=ORIENTED_EDGE ( 'NONE', *, *, #36302, .F. ) ;
#10306=VERTEX_POINT ( 'NONE', #9470 ) ;
#10320=CARTESIAN_POINT ( 'NONE',  ( 22.01541346579904967, 4.834729283906541220, -3.642368534677343117 ) ) ;
#10325=CARTESIAN_POINT ( 'NONE',  ( 26.92542807167190944, 1.449366069832211279, 5.022290288739529984 ) ) ;
#10329=CARTESIAN_POINT ( 'NONE',  ( 32.03973861597579287, -5.079083921188654926, 0.4704245571143086391 ) ) ;
#10330=AXIS2_PLACEMENT_3D ( 'NONE', #32194, #3994, #3595 ) ;
#10336=CARTESIAN_POINT ( 'NONE',  ( 36.73503357909203260, -2.304591497473642558, -5.935222444422922905 ) ) ;
#10346=CARTESIAN_POINT ( 'NONE',  ( 37.02980894656261057, -2.495571335640368371, 5.974001483408611257 ) ) ;
#10354=CARTESIAN_POINT ( 'NONE',  ( 23.23474455812838713, 3.274026224173547828, 3.847451402220932959 ) ) ;
#10357=VECTOR ( 'NONE', #11983, 1000.000000000000000 ) ;
#10358=VECTOR ( 'NONE', #35201, 1000.000000000000114 ) ;
#10361=CARTESIAN_POINT ( 'NONE',  ( 22.61528281558029008, 4.620618817536152889, 3.048381724597784892 ) ) ;
#10367=CARTESIAN_POINT ( 'NONE',  ( 21.79691714197424091, 0.2351871378864240913, 8.326263741760431714 ) ) ;
#10377=CARTESIAN_POINT ( 'NONE',  ( 25.36335546794393281, -3.584835346285432767, 4.690180580146940059 ) ) ;
#10379=CARTESIAN_POINT ( 'NONE',  ( -78.59183336369314077, -5.357290617477898031, 6.436894183391851598 ) ) ;
#10380=DIRECTION ( 'NONE',  ( -0.000000000000000000, -0.000000000000000000, -1.000000000000000000 ) ) ;
#10382=CARTESIAN_POINT ( 'NONE',  ( 22.43263433131228268, 5.122865301372990565, 2.446692766515739859 ) ) ;
#10384=CARTESIAN_POINT ( 'NONE',  ( 35.36788826667455510, -3.790803511439575946, -5.512024906129279422 ) ) ;
#10393=CARTESIAN_POINT ( 'NONE',  ( 26.10580188794843792, 1.913936627547451641, -4.230755467540477710 ) ) ;
#10394=CARTESIAN_POINT ( 'NONE',  ( 30.05259702970372260, 1.006150772074058564, -4.336635385246468744 ) ) ;
#10395=CARTESIAN_POINT ( 'NONE',  ( 16.64247417353310254, 12.36459659714428483, -2.500000000000000888 ) ) ;
#10400=CARTESIAN_POINT ( 'NONE',  ( 86.09116122586011954, 0.08319669091220074919, -6.006182420748226392 ) ) ;
#10402=CARTESIAN_POINT ( 'NONE',  ( 27.43879754216082389, 0.9604377377020558715, 4.488885984917203587 ) ) ;
#10413=CARTESIAN_POINT ( 'NONE',  ( 33.78306522148626101, -4.833110834643807863, 3.502350965566474628 ) ) ;
#10417=DIRECTION ( 'NONE',  ( -7.826543628040252284E-17, 1.000000000000000000, 0.000000000000000000 ) ) ;
#10421=CARTESIAN_POINT ( 'NONE',  ( 33.81163260347297239, -4.968337719301128885, -3.151236393681405623 ) ) ;
#10427=CARTESIAN_POINT ( 'NONE',  ( -72.95788378915689520, 3.814940674406429810, -10.95087388501848125 ) ) ;
#10429=CARTESIAN_POINT ( 'NONE',  ( -72.84815947045233031, 2.429809908903243443, 12.50000000000000000 ) ) ;
#10432=CARTESIAN_POINT ( 'NONE',  ( 86.14505873727070195, -0.01797735283943463491, 5.995667628870159582 ) ) ;
#10433=DIRECTION ( 'NONE',  ( 0.000000000000000000, 1.000000000000000000, 0.000000000000000000 ) ) ;
#10435=B_SPLINE_CURVE_WITH_KNOTS ( 'NONE', 3,
 ( #24056, #36624, #30456, #28169, #31684, #6968, #38048, #23527, #13144, #21098, #32491, #5446 ),
 .UNSPECIFIED., .F., .F.,
 ( 4, 2, 2, 2, 2, 4 ),
 ( 0.004696307191636101344, 0.005283442520392493159, 0.005870577849148884975, 0.006164145513527088255, 0.006457713177905292402, 0.007044848506661660799 ),
 .UNSPECIFIED. ) ;
#10439=CARTESIAN_POINT ( 'NONE',  ( 36.14162845619620157, -3.143484948803114243, 5.847173227813405205 ) ) ;
#10441=CARTESIAN_POINT ( 'NONE',  ( 87.56526962053540331, 0.0002576605070852033049, 4.866394609412610706 ) ) ;
#10445=CARTESIAN_POINT ( 'NONE',  ( 88.16566304253608166, -0.6741327274749846499, -2.283436234569833800 ) ) ;
#10450=ORIENTED_EDGE ( 'NONE', *, *, #32226, .T. ) ;
#10451=ORIENTED_EDGE ( 'NONE', *, *, #4600, .F. ) ;
#10454=CARTESIAN_POINT ( 'NONE',  ( 24.68943462063005967, 2.063637610377018206, 4.241669502777529743 ) ) ;
#10461=B_SPLINE_CURVE_WITH_KNOTS ( 'NONE', 3,
 ( #38976, #10582, #7100, #7297, #19663, #38787, #4432, #16750, #29332, #1151, #13685, #35721, #23944, #14882, #17761, #30553, #33237, #30967, #37120, #21492, #8290, #14474 ),
 .UNSPECIFIED., .F., .F.,
 ( 4, 2, 2, 2, 2, 2, 2, 2, 2, 2, 4 ),
 ( 0.000000000000000000, 0.2499999999999973910, 0.3749999999999961142, 0.4999999999999947820, 0.5624999999999912292, 0.5937499999999934497, 0.6249999999999956701, 0.6874999999999942268, 0.7187499999999961142, 0.7499999999999980016, 1.000000000000000000 ),
 .UNSPECIFIED. ) ;
#10466=CARTESIAN_POINT ( 'NONE',  ( 24.53703648633796774, 2.972983101647284521, -3.608924253653490233 ) ) ;
#10467=VERTEX_POINT ( 'NONE', #17059 ) ;
#10468=CARTESIAN_POINT ( 'NONE',  ( -71.43161014973536282, 0.09092285538556041380, 5.980075040747969695 ) ) ;
#10469=ORIENTED_EDGE ( 'NONE', *, *, #32509, .F. ) ;
#10471=CARTESIAN_POINT ( 'NONE',  ( 21.85643539959776760, -1.193669045901033066, -12.68912657263372346 ) ) ;
#10472=CARTESIAN_POINT ( 'NONE',  ( 21.46948114135319230, 9.243557392228170855, -3.873122283670241917 ) ) ;
#10475=CARTESIAN_POINT ( 'NONE',  ( 87.14484084030976874, 0.3304612005822565313, -5.669005978848654870 ) ) ;
#10476=CARTESIAN_POINT ( 'NONE',  ( 16.74878488105810348, 0.9046941363780687251, 4.803740791053210835 ) ) ;
#10481=CARTESIAN_POINT ( 'NONE',  ( 14.59423631969371193, -5.048651580101616965, -2.484181559264142081 ) ) ;
#10482=CARTESIAN_POINT ( 'NONE',  ( 37.04352256721959691, -2.892790444795046323, -5.987935616230180891 ) ) ;
#10484=CARTESIAN_POINT ( 'NONE',  ( 84.12549522848908623, 2.987061070915658867, -0.8566216743701494662 ) ) ;
#10488=CARTESIAN_POINT ( 'NONE',  ( 28.70277213621809409, -3.561666039817526386, 4.654175941992544807 ) ) ;
#10490=EDGE_LOOP ( 'NONE', ( #25919, #10949, #14956, #21678 ) ) ;
#10491=CARTESIAN_POINT ( 'NONE',  ( 37.17617793620765809, -2.565058875548333894, 5.981048444294359001 ) ) ;
#10492=CARTESIAN_POINT ( 'NONE',  ( -4.224659823956008253, -51.67615071827237472, -2.500000000000000000 ) ) ;
#10494=CARTESIAN_POINT ( 'NONE',  ( 86.93061992748306466, -1.256218166249259749, 5.071404822462298512 ) ) ;
#10504=CARTESIAN_POINT ( 'NONE',  ( 23.64899080490409489, 3.263760929269430289, 3.660893560480292575 ) ) ;
#10513=FACE_OUTER_BOUND ( 'NONE', #20478, .T. ) ;
#10518=CARTESIAN_POINT ( 'NONE',  ( 23.94313517838655869, 2.810339304371657132, -3.943303330136482820 ) ) ;
#10521=B_SPLINE_CURVE_WITH_KNOTS ( 'NONE', 3,
 ( #12291, #370, #24653, #31050, #5925, #9200, #28144, #21780, #18666, #3074, #32668, #3675, #19499, #34965, #32463, #31857, #29365, #32072, #10421, #1382, #575, #20091, #4469, #10612, #22997, #22595, #38415, #6740, #23188, #28967, #35562, #4261, #35757 ),
 .UNSPECIFIED., .F., .F.,
 ( 4, 2, 2, 2, 2, 2, 2, 2, 2, 2, 2, 1, 2, 2, 1, 1, 2, 4 ),
 ( 0.4585963849156251548, 0.4882313195419025753, 0.5030487868550412855, 0.5178662541681799958, 0.5771361234207347257, 0.6067710580470121462, 0.6215885253601507454, 0.6364059926732894557, 0.6956758619258440746, 0.7253107965521212730, 0.7401282638652599832, 0.7475369975218293384, 0.7493891809359716216, 0.7503152726430426522, 0.7512413643501137939, 0.7549457311783988045, 0.8142156004309570871, 0.9327553389360742075 ),
 .UNSPECIFIED. ) ;
#10523=CARTESIAN_POINT ( 'NONE',  ( 30.73735125564872916, -2.095387222228427770, 5.934458408524426076 ) ) ;
#10529=CARTESIAN_POINT ( 'NONE',  ( 34.76593155650069633, -3.465238236085922185, -5.619570445338033515 ) ) ;
#10535=CARTESIAN_POINT ( 'NONE',  ( 21.88744680497111261, -13.17188653508849150, -2.500000000000000888 ) ) ;
#10537=CARTESIAN_POINT ( 'NONE',  ( 30.19003827612802482, -2.952522945788203845, 4.918283640461378781 ) ) ;
#10538=VERTEX_POINT ( 'NONE', #29637 ) ;
#10539=CARTESIAN_POINT ( 'NONE',  ( 36.92447304359136240, -2.367222292930631689, 5.951667485741300112 ) ) ;
#10546=CARTESIAN_POINT ( 'NONE',  ( 30.76799283776897198, -3.322052511316047951, 4.963599853823706276 ) ) ;
#10547=CARTESIAN_POINT ( 'NONE',  ( 85.09607640761747405, 1.741501683616388130, -5.098621195172435172 ) ) ;
#10553=CARTESIAN_POINT ( 'NONE',  ( 22.61513645261399219, 4.622024906660042731, 3.046565464745161655 ) ) ;
#10563=CARTESIAN_POINT ( 'NONE',  ( 21.73476950717714118, 0.2476036213341410441, 9.023233531077035963 ) ) ;
#10567=DIRECTION ( 'NONE',  ( -0.9980241895169804645, 0.000000000000000000, 0.06283086135788849835 ) ) ;
#10572=CARTESIAN_POINT ( 'NONE',  ( 25.32326662574907772, -3.445015843796760624, -4.932833089913290614 ) ) ;
#10574=ORIENTED_EDGE ( 'NONE', *, *, #32833, .F. ) ;
#10575=CARTESIAN_POINT ( 'NONE',  ( -76.43910119853934759, -5.761394667964060190, 8.352738067394287924 ) ) ;
#10579=VERTEX_POINT ( 'NONE', #23653 ) ;
#10581=CARTESIAN_POINT ( 'NONE',  ( 25.73398621336427539, 2.637371603049242896, -3.518938631727759336 ) ) ;
#10582=CARTESIAN_POINT ( 'NONE',  ( 30.24787234978726858, -2.991825711127265919, -4.927310046378262420 ) ) ;
#10593=EDGE_CURVE ( 'NONE', #2020, #4342, #3409, .T. ) ;
#10594=CARTESIAN_POINT ( 'NONE',  ( 87.24982552262115121, -1.326261458569501839, 4.881571762780114732 ) ) ;
#10595=CIRCLE ( 'NONE', #1422, 7.744449365083023729 ) ;
#10598=CARTESIAN_POINT ( 'NONE',  ( -80.67082329696982868, 10.50842065708840067, -5.186806082895198955 ) ) ;
#10602=DIRECTION ( 'NONE',  ( 0.000000000000000000, 0.000000000000000000, 1.000000000000000000 ) ) ;
#10606=CARTESIAN_POINT ( 'NONE',  ( 33.89725028478159174, -5.465908938576614418, 0.4877600842561391481 ) ) ;
#10609=CARTESIAN_POINT ( 'NONE',  ( 24.38340127123625578, 2.573202976557773525, 4.012017501801370400 ) ) ;
#10610=CARTESIAN_POINT ( 'NONE',  ( 20.34585743190884344, 6.625446340279268043, -3.270942662530205602 ) ) ;
#10612=CARTESIAN_POINT ( 'NONE',  ( 33.78877019722047947, -4.859422714393206277, -3.437826128937246484 ) ) ;
#10613=CARTESIAN_POINT ( 'NONE',  ( -70.92837670882201451, -21.78299143689573469, 6.000000000001379341 ) ) ;
#10619=CARTESIAN_POINT ( 'NONE',  ( -75.92415766659136978, -3.925048772356933835, -10.09882139952678948 ) ) ;
#10620=LINE ( 'NONE', #10429, #8988 ) ;
#10627=EDGE_CURVE ( 'NONE', #3011, #5958, #18640, .T. ) ;
#10631=CARTESIAN_POINT ( 'NONE',  ( 22.01541346579904967, 4.834729283906541220, -3.642368534677343117 ) ) ;
#10636=CARTESIAN_POINT ( 'NONE',  ( 35.33522264782425282, -3.171501239445705167, 5.721314098418827321 ) ) ;
#10639=CARTESIAN_POINT ( 'NONE',  ( 84.84279093542515682, 3.008464274580536113, -1.251974654204536908 ) ) ;
#10645=CARTESIAN_POINT ( 'NONE',  ( -80.30224715670834712, 11.50583414542592742, -3.508222272703448663 ) ) ;
#10647=ORIENTED_EDGE ( 'NONE', *, *, #34625, .F. ) ;
#10653=CARTESIAN_POINT ( 'NONE',  ( 24.35217137059073522, 1.294611633738677270, 4.709786998218760345 ) ) ;
#10656=DIRECTION ( 'NONE',  ( 1.000000000000000000, 1.776143608908745286E-15, 0.000000000000000000 ) ) ;
#10662=CARTESIAN_POINT ( 'NONE',  ( 21.81164502259897731, 5.201711882885422078, -3.655446855725318134 ) ) ;
#10666=CARTESIAN_POINT ( 'NONE',  ( 22.36058758039612471, 3.933412737179332375, -7.046732538784932665 ) ) ;
#10667=CARTESIAN_POINT ( 'NONE',  ( 21.88165365390326400, 4.350072964282386323, 2.563907282946755012E-12 ) ) ;
#10668=CARTESIAN_POINT ( 'NONE',  ( 16.08591480223022074, 7.879342699536265648, 3.484773800359155960 ) ) ;
#10671=CARTESIAN_POINT ( 'NONE',  ( 86.69901843299427924, 0.4902165918510832388, 5.965927736749048194 ) ) ;
#10675=CARTESIAN_POINT ( 'NONE',  ( -81.60021392995659539, -5.622709797487786432, 2.348518091125527008 ) ) ;
#10677=CARTESIAN_POINT ( 'NONE',  ( -70.92837670882107659, 13.87661300689599742, 10.00000000000000533 ) ) ;
#10678=CARTESIAN_POINT ( 'NONE',  ( 18.20696997742687984, -2.825060525577835602, -3.048036020847092242 ) ) ;
#10679=CARTESIAN_POINT ( 'NONE',  ( 27.40537536757053161, 0.9587627913666219026, -4.483669646254042185 ) ) ;
#10681=CARTESIAN_POINT ( 'NONE',  ( 84.47786603692917140, 2.553026049322892455, -3.367302602819985058 ) ) ;
#10682=CARTESIAN_POINT ( 'NONE',  ( 28.66920249112477848, -4.024975064351027143, -4.110187144531254333 ) ) ;
#10685=ADVANCED_FACE ( 'NONE', ( #11364 ), #36909, .T. ) ;
#10690=ORIENTED_EDGE ( 'NONE', *, *, #38245, .T. ) ;
#10691=CARTESIAN_POINT ( 'NONE',  ( 33.11281012697673276, -0.1525902709989853945, 4.944059908066099851 ) ) ;
#10692=CARTESIAN_POINT ( 'NONE',  ( 16.45184370577523225, -3.221501287979960715, 2.774106118266566945 ) ) ;
#10693=CARTESIAN_POINT ( 'NONE',  ( -69.42837670882107659, -47.11702805680359063, 38.00000000000000711 ) ) ;
#10694=CARTESIAN_POINT ( 'NONE',  ( 86.19214148621283300, -0.1009238796382747189, 5.955419684790980384 ) ) ;
#10701=CARTESIAN_POINT ( 'NONE',  ( 23.17633557675668143, 3.725374598916875168, 3.475392858078595104 ) ) ;
#10707=DIRECTION ( 'NONE',  ( -0.000000000000000000, 1.000000000000000000, -0.000000000000000000 ) ) ;
#10710=CARTESIAN_POINT ( 'NONE',  ( 22.50620321255335554, 2.285223840635106640, -5.090854016693098671 ) ) ;
#10713=CARTESIAN_POINT ( 'NONE',  ( 25.62569289649984583, 1.971242808189318296, -4.205907154860246244 ) ) ;
#10718=CARTESIAN_POINT ( 'NONE',  ( 29.97449823033972649, -1.245471885678776980, 6.039028575696650414 ) ) ;
#10720=CARTESIAN_POINT ( 'NONE',  ( 25.51679268433478853, -4.687544639108172539, 0.4528783670679029094 ) ) ;
#10725=CARTESIAN_POINT ( 'NONE',  ( 36.92999076337549269, -2.615982695873473762, -5.970216232463218198 ) ) ;
#10730=ADVANCED_FACE ( 'NONE', ( #17953 ), #20849, .F. ) ;
#10734=CARTESIAN_POINT ( 'NONE',  ( 20.76538735788932399, 4.421521651906416217, 3.217090461606771701 ) ) ;
#10735=B_SPLINE_CURVE_WITH_KNOTS ( 'NONE', 3,
 ( #27052, #39186, #32838, #39597, #39814, #11381, #20868, #5229, #23946, #4630, #11582, #33032, #17764, #13885 ),
 .UNSPECIFIED., .F., .F.,
 ( 4, 2, 2, 2, 2, 2, 4 ),
 ( 1.390486644391990834E-17, 0.0002943548652378657647, 0.0005887097304757176516, 0.0008830645957135694300, 0.001177419460951421425, 0.001766129191427110454, 0.002354838921902799483 ),
 .UNSPECIFIED. ) ;
#10739=VERTEX_POINT ( 'NONE', #10613 ) ;
#10747=CARTESIAN_POINT ( 'NONE',  ( 21.71285251252540505, 6.321249563836915719, 3.195723793048483863 ) ) ;
#10751=AXIS2_PLACEMENT_3D ( 'NONE', #22341, #35104, #13450 ) ;
#10755=CARTESIAN_POINT ( 'NONE',  ( 21.97782326148428211, 0.2280598603087039544, 7.713529440660342296 ) ) ;
#10759=AXIS2_PLACEMENT_3D ( 'NONE', #19376, #14137, #26713 ) ;
#10760=DIRECTION ( 'NONE',  ( -0.06282940500769126912, -0.006808616672654400036, -0.9980010564149641716 ) ) ;
#10766=CARTESIAN_POINT ( 'NONE',  ( 30.07020345058763766, -4.232275913155626235, -2.900971327107725983 ) ) ;
#10769=CARTESIAN_POINT ( 'NONE',  ( -73.70040385515898151, -1.203501491044927763, 10.84085080396863532 ) ) ;
#10770=CARTESIAN_POINT ( 'NONE',  ( 22.29883823987281843, 0.2632337822729923227, -7.099254618854787147 ) ) ;
#10773=ORIENTED_EDGE ( 'NONE', *, *, #2122, .F. ) ;
#10774=CARTESIAN_POINT ( 'NONE',  ( 23.38445862666371511, 3.558655165361555905, -3.098096260192995111 ) ) ;
#10778=DIRECTION ( 'NONE',  ( 1.000000000000000000, 0.000000000000000000, 0.000000000000000000 ) ) ;
#10789=CARTESIAN_POINT ( 'NONE',  ( 86.54029261786013194, -0.3196574014320466284, 5.877194713501632251 ) ) ;
#10791=ORIENTED_EDGE ( 'NONE', *, *, #11089, .F. ) ;
#10792=CARTESIAN_POINT ( 'NONE',  ( -73.56175482597444670, 5.777891328422431805, -10.86681767987946934 ) ) ;
#10796=CARTESIAN_POINT ( 'NONE',  ( 25.27016851667936237, -3.231043682594727073, 4.010790585719321122 ) ) ;
#10805=AXIS2_PLACEMENT_3D ( 'NONE', #34778, #38426, #32086 ) ;
#10810=ADVANCED_FACE ( 'NONE', ( #9723 ), #18160, .F. ) ;
#10811=CARTESIAN_POINT ( 'NONE',  ( 21.85643539959774273, -6.795129563591141064, 12.90182208710982259 ) ) ;
#10816=CIRCLE ( 'NONE', #33210, 6.000000000000002665 ) ;
#10817=CARTESIAN_POINT ( 'NONE',  ( 14.62198803971679872, -4.616044494662263631, 2.500000000000223377 ) ) ;
#10818=CARTESIAN_POINT ( 'NONE',  ( -72.84060385100936230, 2.621073588131995979, -10.96223601709252193 ) ) ;
#10833=CARTESIAN_POINT ( 'NONE',  ( 36.63346434955200692, -3.080208230909283085, 5.923936114067666736 ) ) ;
#10835=AXIS2_PLACEMENT_3D ( 'NONE', #30661, #10881, #17254 ) ;
#10838=CARTESIAN_POINT ( 'NONE',  ( 85.57721755140556752, 2.175474006149249018, 4.430974418963669059 ) ) ;
#10845=DIRECTION ( 'NONE',  ( 0.000000000000000000, 1.000000000000000000, 0.000000000000000000 ) ) ;
#10852=CARTESIAN_POINT ( 'NONE',  ( 23.99396089256777387, 1.018594166801584100, 4.989981842188739414 ) ) ;
#10858=ADVANCED_FACE ( 'NONE', ( #18999 ), #5827, .F. ) ;
#10860=CARTESIAN_POINT ( 'NONE',  ( 23.99288918444596419, 3.298330898318068360, -3.389965429840589461 ) ) ;
#10861=VERTEX_POINT ( 'NONE', #15078 ) ;
#10864=ORIENTED_EDGE ( 'NONE', *, *, #25124, .T. ) ;
#10866=CARTESIAN_POINT ( 'NONE',  ( 22.77977322753350720, -5.661609348961630594, -5.678499401198807917 ) ) ;
#10868=AXIS2_PLACEMENT_3D ( 'NONE', #33768, #15210, #2072 ) ;
#10869=CARTESIAN_POINT ( 'NONE',  ( 16.91049418450527853, 9.757949552745497357, 2.499999999999927169 ) ) ;
#10872=CARTESIAN_POINT ( 'NONE',  ( 85.55911739799610416, 1.969564878966352905, 4.951173091362058187 ) ) ;
#10880=CARTESIAN_POINT ( 'NONE',  ( 34.13636567165694657, -3.129955875004838628, -5.534203472820675707 ) ) ;
#10881=DIRECTION ( 'NONE',  ( 0.000000000000000000, -0.000000000000000000, -1.000000000000000000 ) ) ;
#10882=CARTESIAN_POINT ( 'NONE',  ( 84.29260032154424209, 2.783174668905456617, -2.501150759418095504 ) ) ;
#10883=CARTESIAN_POINT ( 'NONE',  ( 30.23789859557072646, -3.686283672430305636, -4.621445095038371420 ) ) ;
#10890=CARTESIAN_POINT ( 'NONE',  ( 29.48876346201022614, 1.220278706431014104, 4.220659031012087503 ) ) ;
#10896=CIRCLE ( 'NONE', #10232, 10.00000000000000888 ) ;
#10899=CARTESIAN_POINT ( 'NONE',  ( -69.92837670882107659, -0.7829914368874778541, 38.00000000000000711 ) ) ;
#10901=CARTESIAN_POINT ( 'NONE',  ( 21.87278005295212324, 2.930088050433418800, 3.925081081565170660 ) ) ;
#10904=CARTESIAN_POINT ( 'NONE',  ( 23.69208156265775145, 3.471075682706086685, 3.392352389993136264 ) ) ;
#10911=CARTESIAN_POINT ( 'NONE',  ( 14.77222818450456643, -4.461908109758233820, -2.511961494517393145 ) ) ;
#10914=CARTESIAN_POINT ( 'NONE',  ( 22.24968006774034990, 3.032303245382528711, -4.686988268442751071 ) ) ;
#10919=CARTESIAN_POINT ( 'NONE',  ( 24.23747724132151760, 2.648570161240320964, -3.989242527747176137 ) ) ;
#10923=CARTESIAN_POINT ( 'NONE',  ( 85.70831578087668845, 2.086076349557777654, 3.711011680213312403 ) ) ;
#10924=CARTESIAN_POINT ( 'NONE',  ( 31.80158048871438581, -1.669318041804891850, 6.009059823207920203 ) ) ;
#10927=CARTESIAN_POINT ( 'NONE',  ( -81.77946201182784591, -5.605489059854700251, -1.058732183306707153 ) ) ;
#10931=CARTESIAN_POINT ( 'NONE',  ( 36.64788811273031399, -3.154273958936592237, -5.926187291151666869 ) ) ;
#10938=CARTESIAN_POINT ( 'NONE',  ( 21.48247406815364613, 3.876925869359153509, 3.508130194431774207 ) ) ;
#10949=ORIENTED_EDGE ( 'NONE', *, *, #39961, .T. ) ;
#10950=CARTESIAN_POINT ( 'NONE',  ( 21.99629294673994551, 5.575760840298564780, 3.113047709983713940 ) ) ;
#10954=ORIENTED_EDGE ( 'NONE', *, *, #16571, .T. ) ;
#10956=CARTESIAN_POINT ( 'NONE',  ( 25.40497407019471865, 0.6693547542586180121, 4.599869742869072908 ) ) ;
#10958=CIRCLE ( 'NONE', #27396, 21.28220113893567245 ) ;
#10961=VECTOR ( 'NONE', #20192, 1000.000000000000000 ) ;
#10965=ADVANCED_FACE ( 'NONE', ( #31973 ), #20073, .T. ) ;
#10968=CARTESIAN_POINT ( 'NONE',  ( 28.08579234408868786, -0.7886013899455160958, -6.074239229908586779 ) ) ;
#10970=ORIENTED_EDGE ( 'NONE', *, *, #25915, .T. ) ;
#10972=CARTESIAN_POINT ( 'NONE',  ( 24.74154467618137332, 0.6006174455902917320, -4.777991240237089876 ) ) ;
#10976=CARTESIAN_POINT ( 'NONE',  ( 37.10393103747592392, -3.125961714947245174, -5.976270759528274468 ) ) ;
#10977=DIRECTION ( 'NONE',  ( 1.000000000000000000, 0.000000000000000000, 0.000000000000000000 ) ) ;
#10990=CARTESIAN_POINT ( 'NONE',  ( 84.23599009083828548, 2.852497016463987567, -2.111805961397795084 ) ) ;
#10993=DIRECTION ( 'NONE',  ( 0.000000000000000000, -0.000000000000000000, 1.000000000000000000 ) ) ;
#10996=ORIENTED_EDGE ( 'NONE', *, *, #27148, .T. ) ;
#10998=CARTESIAN_POINT ( 'NONE',  ( 14.38908530706053490, 8.635444686654100366, -3.482730190673553938 ) ) ;
#11004=DIRECTION ( 'NONE',  ( 0.000000000000000000, 0.000000000000000000, 1.000000000000000000 ) ) ;
#11006=CARTESIAN_POINT ( 'NONE',  ( 21.85643539959775694, 5.081979399238238493, 12.23420521612613143 ) ) ;
#11012=CARTESIAN_POINT ( 'NONE',  ( 14.75848712228891912, -5.150036851632115109, 2.500000000037279957 ) ) ;
#11013=CARTESIAN_POINT ( 'NONE',  ( -79.28524469389549267, 10.39485579098267287, -5.506563355727433162 ) ) ;
#11015=CARTESIAN_POINT ( 'NONE',  ( 36.49377363026633248, -3.561668432020718367, -5.795624143399630945 ) ) ;
#11023=CARTESIAN_POINT ( 'NONE',  ( 87.46698719228061236, 0.1106531486882382370, 4.398961038131239398 ) ) ;
#11027=CARTESIAN_POINT ( 'NONE',  ( 21.25657249720342890, 3.328711648262387079, 3.524000248973877980 ) ) ;
#11031=CARTESIAN_POINT ( 'NONE',  ( 86.06476644049696745, 1.615394338423677079, -5.255309406831162988 ) ) ;
#11033=CARTESIAN_POINT ( 'NONE',  ( 28.38493088217029836, 0.6184565668324991661, -4.636552974946980932 ) ) ;
#11035=LINE ( 'NONE', #19527, #32045 ) ;
#11038=CARTESIAN_POINT ( 'NONE',  ( -76.03073930765792454, 10.38232506267625688, -8.602311807112798192 ) ) ;
#11049=CARTESIAN_POINT ( 'NONE',  ( 21.92288564526636563, 0.6275057185515289238, 7.506979565206076899 ) ) ;
#11056=CARTESIAN_POINT ( 'NONE',  ( 19.45444762555048968, 11.13896630658038056, 2.499999999999995115 ) ) ;
#11060=CARTESIAN_POINT ( 'NONE',  ( 23.40982567674854309, 3.536491107301646064, -3.507547231203631988 ) ) ;
#11064=CARTESIAN_POINT ( 'NONE',  ( 21.85643539959776760, 7.937350203533870996, 6.559150378249414715 ) ) ;
#11065=CARTESIAN_POINT ( 'NONE',  ( 17.82514609008682172, 11.84176510169323748, 2.499999999999998668 ) ) ;
#11068=CARTESIAN_POINT ( 'NONE',  ( 84.32156544206206661, 3.079100735703119707, -0.4907544566128131391 ) ) ;
#11071=DIRECTION ( 'NONE',  ( -1.000000000000000000, 0.000000000000000000, 0.000000000000000000 ) ) ;
#11074=CARTESIAN_POINT ( 'NONE',  ( 21.50914624065722691, -2.894264267616096120, -3.541302231922554000 ) ) ;
#11075=CARTESIAN_POINT ( 'NONE',  ( 37.04510231533804898, -2.801254996599130020, -5.988182174130333379 ) ) ;
#11077=CARTESIAN_POINT ( 'NONE',  ( 22.34798716198837454, 0.2922943786608916961, -6.997897115895016285 ) ) ;
#11082=CARTESIAN_POINT ( 'NONE',  ( 32.42603576456313164, -3.007759285847489750, -5.267265126335289871 ) ) ;
#11084=VERTEX_POINT ( 'NONE', #17201 ) ;
#11085=ORIENTED_EDGE ( 'NONE', *, *, #250, .F. ) ;
#11086=CARTESIAN_POINT ( 'NONE',  ( 30.88361545799471486, 0.6996882436838504082, 4.491048756100919803 ) ) ;
#11089=EDGE_CURVE ( 'NONE', #18492, #3377, #7941, .T. ) ;
#11101=CARTESIAN_POINT ( 'NONE',  ( 22.46827172332250200, 4.617652435747735318, 3.274651054683074491 ) ) ;
#11105=CARTESIAN_POINT ( 'NONE',  ( 14.61802081865033642, -4.461995682952384357, -2.500000000000000000 ) ) ;
#11108=CARTESIAN_POINT ( 'NONE',  ( 24.89046942861130063, -2.711312442094912623, -4.091157751249474117 ) ) ;
#11109=CARTESIAN_POINT ( 'NONE',  ( 20.71918928157063178, 6.165415561970744918, -3.398715681700897662 ) ) ;
#11111=CARTESIAN_POINT ( 'NONE',  ( 21.84929449939717117, 2.757990278203812817, -5.323232446221868308 ) ) ;
#11117=CARTESIAN_POINT ( 'NONE',  ( 27.43879703630890887, 0.9604363013853572939, -4.488885905966782275 ) ) ;
#11121=CARTESIAN_POINT ( 'NONE',  ( 85.09836244081553502, 2.771204891246429547, 1.045684100250478643 ) ) ;
#11122=CARTESIAN_POINT ( 'NONE',  ( 31.86155337613836380, -4.142523116122148963, 4.178567150506776962 ) ) ;
#11124=CARTESIAN_POINT ( 'NONE',  ( -80.78031099096216394, -5.651013701725611682, -4.946895140558772219 ) ) ;
#11126=CARTESIAN_POINT ( 'NONE',  ( 14.79476812666557350, -5.587083218280035624, 2.503656380302125228 ) ) ;
#11128=CARTESIAN_POINT ( 'NONE',  ( 34.76872341006280465, -3.305568305793640693, -5.632898191526192200 ) ) ;
#11132=VECTOR ( 'NONE', #17442, 1000.000000000000000 ) ;
#11136=CARTESIAN_POINT ( 'NONE',  ( 33.67412422684426332, -3.719468122262790999, 5.264089307504189463 ) ) ;
#11140=FACE_OUTER_BOUND ( 'NONE', #21635, .T. ) ;
#11150=CARTESIAN_POINT ( 'NONE',  ( 21.83153479609358882, 5.955861309579818297, 3.139072512424320838 ) ) ;
#11151=DIRECTION ( 'NONE',  ( 0.000000000000000000, 0.000000000000000000, -1.000000000000000000 ) ) ;
#11156=CARTESIAN_POINT ( 'NONE',  ( 26.76119839104307729, 0.8702342918438391584, 4.383274761122565089 ) ) ;
#11157=CARTESIAN_POINT ( 'NONE',  ( 14.68539485748044626, -4.702058589831320745, -2.500000000000172307 ) ) ;
#11160=VERTEX_POINT ( 'NONE', #39636 ) ;
#11164=CARTESIAN_POINT ( 'NONE',  ( 63.05383694556373797, -7.271989087314214117, -6.000000000000000000 ) ) ;
#11165=CARTESIAN_POINT ( 'NONE',  ( 30.06379901557190237, -4.186058752285889639, 3.090730270791094636 ) ) ;
#11169=CARTESIAN_POINT ( 'NONE',  ( 27.43552295442261268, 0.9748355693916180842, -4.488373114136018138 ) ) ;
#11175=CARTESIAN_POINT ( 'NONE',  ( 27.81554284938481203, 1.843609864746671212, -3.908850080722512388 ) ) ;
#11179=DIRECTION ( 'NONE',  ( -0.000000000000000000, 0.000000000000000000, 1.000000000000000000 ) ) ;
#11189=CARTESIAN_POINT ( 'NONE',  ( 86.70396871743868417, -0.5679530053852996918, -5.718564545587779158 ) ) ;
#11200=CIRCLE ( 'NONE', #17758, 10.00000000000000533 ) ;
#11203=CARTESIAN_POINT ( 'NONE',  ( 17.60335279841272182, 11.93951228567222600, -2.500000000000012434 ) ) ;
#11210=CARTESIAN_POINT ( 'NONE',  ( 21.85643539959777826, -5.315239383820637542, 13.63683724657638052 ) ) ;
#11211=CARTESIAN_POINT ( 'NONE',  ( -79.02304780370427295, 11.44793877116905101, 5.885444661546937795 ) ) ;
#11213=CARTESIAN_POINT ( 'NONE',  ( 14.72131129160176322, -5.032869250705308772, 2.500000000000122569 ) ) ;
#11214=CARTESIAN_POINT ( 'NONE',  ( -79.95507389475284299, 10.45503264499227214, -6.471215697590134930 ) ) ;
#11216=CARTESIAN_POINT ( 'NONE',  ( 36.87241546289296679, -2.085184201125469539, -5.863287844626394296 ) ) ;
#11224=AXIS2_PLACEMENT_3D ( 'NONE', #30762, #17963, #8494 ) ;
#11225=CARTESIAN_POINT ( 'NONE',  ( 87.61513118388886312, -0.05574921402413471339, 4.133600037482800360 ) ) ;
#11229=CARTESIAN_POINT ( 'NONE',  ( 36.90765050460312580, -3.026038577865985513, 5.966729494780605769 ) ) ;
#11232=CARTESIAN_POINT ( 'NONE',  ( 87.01296019436635731, 0.4868102506410553754, -5.723292304581113044 ) ) ;
#11235=CARTESIAN_POINT ( 'NONE',  ( 33.62515361724260998, -1.226752319248198164, -5.454416468020780506 ) ) ;
#11246=CARTESIAN_POINT ( 'NONE',  ( 23.56014592707593280, 1.105608511620937984, 5.220594937748640696 ) ) ;
#11256=CARTESIAN_POINT ( 'NONE',  ( 23.15910336873031738, 3.906749609004425139, -3.275810519260066389 ) ) ;
#11259=CARTESIAN_POINT ( 'NONE',  ( 21.85643539959778181, 8.766930670454163632, 4.215001190429523703 ) ) ;
#11261=CARTESIAN_POINT ( 'NONE',  ( 21.88097534389255472, 3.372061099796740180, -3.393279653742926172 ) ) ;
#11265=CARTESIAN_POINT ( 'NONE',  ( 85.43170627155664931, 2.122511629702291902, -4.702826977918449280 ) ) ;
#11272=CARTESIAN_POINT ( 'NONE',  ( 19.69748393801550534, -3.013861005515011904, -3.228077426689117235 ) ) ;
#11273=CARTESIAN_POINT ( 'NONE',  ( 36.89660107519480903, -3.000806692559368383, -5.965004964089976269 ) ) ;
#11274=CARTESIAN_POINT ( 'NONE',  ( 14.69558838330753581, -65.19654454972992141, -2.500000000000000444 ) ) ;
#11275=CIRCLE ( 'NONE', #21834, 21.28220113893567245 ) ;
#11276=CARTESIAN_POINT ( 'NONE',  ( 24.64884766327626053, 0.7497537406995623543, -4.794175230417015321 ) ) ;
#11279=CARTESIAN_POINT ( 'NONE',  ( 20.42173045687939137, 3.659900802137024733, 3.393702957850269541 ) ) ;
#11280=CARTESIAN_POINT ( 'NONE',  ( 30.19238557334687911, -2.952639005720375742, -4.918649992961978690 ) ) ;
#11284=CARTESIAN_POINT ( 'NONE',  ( 27.81753993201519393, 1.846270399565714371, 3.902048507340946326 ) ) ;
#11294=CARTESIAN_POINT ( 'NONE',  ( 14.75726152236038935, -4.580480956772500889, 2.509421305520750600 ) ) ;
#11297=CARTESIAN_POINT ( 'NONE',  ( 22.52624294278324157, 4.322728351962980220, 3.478153892842317241 ) ) ;
#11303=CARTESIAN_POINT ( 'NONE',  ( 26.16692636534402538, -2.761581989583650198, -4.290379727454292080 ) ) ;
#11307=CARTESIAN_POINT ( 'NONE',  ( 22.04746162069255533, 2.900181437439750542, -4.981729368850734474 ) ) ;
#11312=DIRECTION ( 'NONE',  ( 1.000000000000000000, 0.000000000000000000, 0.000000000000000000 ) ) ;
#11315=CARTESIAN_POINT ( 'NONE',  ( 86.40868413783579172, 1.299389369533768379, 4.865112849554557251 ) ) ;
#11317=CARTESIAN_POINT ( 'NONE',  ( 31.44014676667174157, -3.103618331322294921, 5.406754918213918515 ) ) ;
#11325=CARTESIAN_POINT ( 'NONE',  ( 36.68769143235972763, -2.387623739369580722, -5.932399561826603218 ) ) ;
#11328=FACE_BOUND ( 'NONE', #27312, .T. ) ;
#11331=ADVANCED_FACE ( 'NONE', ( #19055 ), #22364, .T. ) ;
#11333=CARTESIAN_POINT ( 'NONE',  ( 27.74721017235163600, 1.752453911456003599, 4.134717658254572825 ) ) ;
#11337=CARTESIAN_POINT ( 'NONE',  ( -62.92837670882106238, -23.80776546975053520, 6.000000000000000000 ) ) ;
#11339=PLANE ( 'NONE',  #30523 ) ;
#11341=CARTESIAN_POINT ( 'NONE',  ( 85.67826002946482333, 0.8418862626009593342, -5.872190610739490779 ) ) ;
#11342=LINE ( 'NONE', #34595, #35371 ) ;
#11347=CARTESIAN_POINT ( 'NONE',  ( 21.83642765803570995, 5.927067409592997826, 3.151569157035945867 ) ) ;
#11354=CARTESIAN_POINT ( 'NONE',  ( 21.73387441235908923, 0.2123480426500482521, 9.115313740638288920 ) ) ;
#11361=CARTESIAN_POINT ( 'NONE',  ( 36.31056033868917154, -3.612627279154186244, -5.748865049962640583 ) ) ;
#11364=FACE_OUTER_BOUND ( 'NONE', #27578, .T. ) ;
#11365=CARTESIAN_POINT ( 'NONE',  ( 14.69558838330753936, -3.003688195628454238, 6.000000000000001776 ) ) ;
#11366=CARTESIAN_POINT ( 'NONE',  ( 28.10280119166142399, -0.8120181649793116740, 6.074162340139093175 ) ) ;
#11371=CARTESIAN_POINT ( 'NONE',  ( 21.97527673563478956, 0.2261748271463902005, -7.720852451735783717 ) ) ;
#11378=CARTESIAN_POINT ( 'NONE',  ( 35.21965174470370386, -1.049964233957617177, -5.413429237120623405 ) ) ;
#11381=CARTESIAN_POINT ( 'NONE',  ( -71.59512852109486403, -48.46428640673855170, 5.963535602158745341 ) ) ;
#11390=LINE ( 'NONE', #1971, #19962 ) ;
#11400=EDGE_CURVE ( 'NONE', #4251, #36906, #15958, .T. ) ;
#11401=ORIENTED_EDGE ( 'NONE', *, *, #6381, .T. ) ;
#11403=CARTESIAN_POINT ( 'NONE',  ( 17.73032643950705989, 9.401816356539047348, -2.499999999999722888 ) ) ;
#11410=CARTESIAN_POINT ( 'NONE',  ( 18.59223163685811997, 13.14295818854019871, 2.500000000000000444 ) ) ;
#11411=CARTESIAN_POINT ( 'NONE',  ( 21.85643539959779957, 4.362886173974390935, 14.46802226367788791 ) ) ;
#11412=VERTEX_POINT ( 'NONE', #38580 ) ;
#11413=CARTESIAN_POINT ( 'NONE',  ( -79.95320165109795596, 10.45477653335570878, 6.473989127779994135 ) ) ;
#11414=EDGE_CURVE ( 'NONE', #24169, #27368, #16320, .T. ) ;
#11415=CARTESIAN_POINT ( 'NONE',  ( 14.77222419049203594, -4.492314308407749479, 2.511960871155140218 ) ) ;
#11419=CARTESIAN_POINT ( 'NONE',  ( -80.20725398478467127, 11.50953281160756347, -3.750582765600833923 ) ) ;
#11433=CARTESIAN_POINT ( 'NONE',  ( 36.42662174935294672, -3.159887864482101794, 5.891653323799407538 ) ) ;
#11435=CARTESIAN_POINT ( 'NONE',  ( 87.69705646362149309, -0.3167607505441215610, 5.204154330927820205 ) ) ;
#11436=CARTESIAN_POINT ( 'NONE',  ( 32.92332271219583362, -2.910100397871670186, 5.759571882993297365 ) ) ;
#11449=CARTESIAN_POINT ( 'NONE',  ( 22.73568268706182849, 0.4048558432997723111, 6.305629274227928960 ) ) ;
#11452=VECTOR ( 'NONE', #21846, 1000.000000000000000 ) ;
#11459=CARTESIAN_POINT ( 'NONE',  ( 24.03489882237598252, 3.326192361758713467, -3.293071421972179724 ) ) ;
#11463=CARTESIAN_POINT ( 'NONE',  ( 22.80949115205394406, -6.484386712482024251, -3.653976874014524867 ) ) ;
#11464=CARTESIAN_POINT ( 'NONE',  ( 21.87484035781776726, 3.535422555137202494, -3.391095861098737174 ) ) ;
#11469=CARTESIAN_POINT ( 'NONE',  ( 84.96877181165257298, 2.299433286287765554, -4.273906790846864645 ) ) ;
#11478=CARTESIAN_POINT ( 'NONE',  ( 17.05638849885697894, -3.260855927369440188, -2.842766561921666213 ) ) ;
#11480=LINE ( 'NONE', #36819, #20080 ) ;
#11482=CARTESIAN_POINT ( 'NONE',  ( 24.59788967097932044, 0.8378664169005234363, -4.794031594194660961 ) ) ;
#11484=ORIENTED_EDGE ( 'NONE', *, *, #36133, .F. ) ;
#11485=CARTESIAN_POINT ( 'NONE',  ( 35.45221327798894606, -1.918015286137918052, 5.739573315685131405 ) ) ;
#11487=CARTESIAN_POINT ( 'NONE',  ( 31.86443645673159963, -2.967394441500424751, -5.179613972017589774 ) ) ;
#11491=CARTESIAN_POINT ( 'NONE',  ( 33.11469321899686236, -0.1493061854001800637, 4.939395549459463908 ) ) ;
#11492=CARTESIAN_POINT ( 'NONE',  ( 24.89998026755250393, -2.711650026429365479, 4.092642147686758491 ) ) ;
#11500=CARTESIAN_POINT ( 'NONE',  ( 14.74756118481574774, -5.100620622190623621, 2.500104659008372643 ) ) ;
#11502=CARTESIAN_POINT ( 'NONE',  ( -62.92837670882106238, -52.49535338866468948, -6.000000000000000000 ) ) ;
#11504=CARTESIAN_POINT ( 'NONE',  ( 23.20559657321298275, 3.453218578186380672, 3.711049198623960432 ) ) ;
#11514=CARTESIAN_POINT ( 'NONE',  ( 24.13946561501993671, 2.647771132776644887, -4.002951860888451563 ) ) ;
#11516=PLANE ( 'NONE',  #7657 ) ;
#11522=CARTESIAN_POINT ( 'NONE',  ( 87.74221684178165503, -0.1984978568185522818, 3.841619981418926244 ) ) ;
#11528=CARTESIAN_POINT ( 'NONE',  ( 36.64077810573005678, -3.117975142819385148, -5.925077602603106897 ) ) ;
#11531=DIRECTION ( 'NONE',  ( -1.385724075720358314E-16, 1.000000000000000000, 0.000000000000000000 ) ) ;
#11534=ORIENTED_EDGE ( 'NONE', *, *, #40244, .T. ) ;
#11535=CARTESIAN_POINT ( 'NONE',  ( 34.57549087153120837, -0.8971447047965824817, 5.398446312640987621 ) ) ;
#11549=CARTESIAN_POINT ( 'NONE',  ( 23.73921823260045372, 3.555442417871877314, 3.202292173715798107 ) ) ;
#11556=CARTESIAN_POINT ( 'NONE',  ( 23.05624328173124482, 0.3494845576275186216, 5.956316157212953044 ) ) ;
#11557=CARTESIAN_POINT ( 'NONE',  ( 14.78182191374954080, -5.169433146903486431, -2.499999999999999556 ) ) ;
#11566=CARTESIAN_POINT ( 'NONE',  ( 26.73479038929921359, 2.133517298515754668, 4.055905576634827092 ) ) ;
#11568=CARTESIAN_POINT ( 'NONE',  ( -70.92837670882107659, -0.7829914368874778541, 38.00000000000000711 ) ) ;
#11571=CARTESIAN_POINT ( 'NONE',  ( -80.58722291995898956, -6.629895795999400931, 2.621518543355748854 ) ) ;
#11572=CARTESIAN_POINT ( 'NONE',  ( 26.05452957851533924, 0.7951218899326391032, -4.421888884741046688 ) ) ;
#11577=CARTESIAN_POINT ( 'NONE',  ( -72.42837670882110501, -47.31541682994506459, 9.886859966642605357 ) ) ;
#11578=CARTESIAN_POINT ( 'NONE',  ( 36.87014114482988703, -2.088717756108750212, -5.864854126680631552 ) ) ;
#11580=CARTESIAN_POINT ( 'NONE',  ( 37.19747295490952155, -2.841588721108153415, -5.999818660317219887 ) ) ;
#11582=CARTESIAN_POINT ( 'NONE',  ( -72.23889801321112714, -47.87246752859122978, 5.855634630472075663 ) ) ;
#11586=EDGE_CURVE ( 'NONE', #22597, #9007, #40490, .T. ) ;
#11587=CARTESIAN_POINT ( 'NONE',  ( 14.75256470577902057, -4.610397949049963806, -2.508547837535054725 ) ) ;
#11588=CARTESIAN_POINT ( 'NONE',  ( 22.77766753872744232, 1.958428159634223231, -5.124684968651379791 ) ) ;
#11600=VECTOR ( 'NONE', #35764, 1000.000000000000000 ) ;
#11606=ORIENTED_EDGE ( 'NONE', *, *, #32006, .F. ) ;
#11608=CARTESIAN_POINT ( 'NONE',  ( 15.80745346850759603, 8.002139515150915372, -3.484773916741293220 ) ) ;
#11612=LINE ( 'NONE', #8535, #28125 ) ;
#11613=CARTESIAN_POINT ( 'NONE',  ( 21.85643539959781023, -11.34362525346678474, 8.214566034197922306 ) ) ;
#11615=CARTESIAN_POINT ( 'NONE',  ( -79.67174074027452946, 11.50491621841984546, 4.869819349584945556 ) ) ;
#11616=CARTESIAN_POINT ( 'NONE',  ( 14.68780169807769376, -4.611715951047749229, 2.499999999999924505 ) ) ;
#11618=CARTESIAN_POINT ( 'NONE',  ( -75.58662980897157979, 8.514659871459404172, -8.885563836102193136 ) ) ;
#11623=CARTESIAN_POINT ( 'NONE',  ( 14.66778827922366268, 13.14255605609920963, 2.495661121409653127 ) ) ;
#11625=CARTESIAN_POINT ( 'NONE',  ( -77.92837670882107659, 2.429809908903242555, -12.50000000000000000 ) ) ;
#11635=CARTESIAN_POINT ( 'NONE',  ( 27.40853967452441609, 0.9677969527344274514, 4.484163512883236891 ) ) ;
#11638=CARTESIAN_POINT ( 'NONE',  ( 85.22136629666657370, 2.371628277241609517, -4.205523829021379001 ) ) ;
#11639=EDGE_CURVE ( 'NONE', #36975, #18458, #18382, .T. ) ;
#11640=DIRECTION ( 'NONE',  ( 0.000000000000000000, -1.000000000000000000, 0.000000000000000000 ) ) ;
#11644=CARTESIAN_POINT ( 'NONE',  ( -70.12941265528974100, -21.39831437159005390, 5.947290612307118529 ) ) ;
#11651=LINE ( 'NONE', #8772, #27302 ) ;
#11654=CARTESIAN_POINT ( 'NONE',  ( 24.11448298858268657, 0.5898710210986063407, 5.089296224101761190 ) ) ;
#11656=VERTEX_POINT ( 'NONE', #6046 ) ;
#11665=CARTESIAN_POINT ( 'NONE',  ( 23.14273095532835001, 4.006691610855233066, -3.147203323943627229 ) ) ;
#11668=CARTESIAN_POINT ( 'NONE',  ( 24.99455384622441301, -2.608472216378299180, -6.027016329390949778 ) ) ;
#11670=DIRECTION ( 'NONE',  ( -0.000000000000000000, 1.000000000000000000, -0.000000000000000000 ) ) ;
#11672=CARTESIAN_POINT ( 'NONE',  ( 86.04767080185138184, 0.5164224212623146348, 6.001289606117265585 ) ) ;
#11677=CARTESIAN_POINT ( 'NONE',  ( 33.97225482870646118, -3.752748478265877541, -5.291075728257928823 ) ) ;
#11685=CARTESIAN_POINT ( 'NONE',  ( 86.31823139319517679, 1.400990185460310844, -4.784756222713710372 ) ) ;
#11689=CARTESIAN_POINT ( 'NONE',  ( 37.17692586084726969, -2.564445794282764979, 5.980943416423468939 ) ) ;
#11690=CARTESIAN_POINT ( 'NONE',  ( 17.97890173384453760, -2.875347590309559553, 3.012440455584755039 ) ) ;
#11703=CARTESIAN_POINT ( 'NONE',  ( 14.76534721654833504, -5.157638883270574404, 2.500001661686563015 ) ) ;
#11705=CARTESIAN_POINT ( 'NONE',  ( 24.54080388820417014, 2.535510198792493508, 4.001279714722917547 ) ) ;
#11710=ORIENTED_EDGE ( 'NONE', *, *, #19677, .F. ) ;
#11712=CARTESIAN_POINT ( 'NONE',  ( 16.54345625214024196, -3.183194016283426908, -2.788404471784634797 ) ) ;
#11713=CARTESIAN_POINT ( 'NONE',  ( -70.92837670882107659, -56.35932253828835314, -6.000000000000002665 ) ) ;
#11716=CARTESIAN_POINT ( 'NONE',  ( 22.64042881234975724, 3.244544948583774513, -4.225217879000846999 ) ) ;
#11719=CARTESIAN_POINT ( 'NONE',  ( 21.85643539959777470, -5.967561930184303698, -15.30482168765389694 ) ) ;
#11724=CARTESIAN_POINT ( 'NONE',  ( 86.69860591627480062, 0.9737354674733970095, 5.003702464200671329 ) ) ;
#11725=DIRECTION ( 'NONE',  ( -0.7877517966954343809, 0.6159927814537400348, 0.000000000000000000 ) ) ;
#11728=DIRECTION ( 'NONE',  ( -0.000000000000000000, 1.000000000000000000, -0.000000000000000000 ) ) ;
#11730=CARTESIAN_POINT ( 'NONE',  ( 36.91148996621163292, -2.638676746795284078, -5.967328735622324132 ) ) ;
#11734=CARTESIAN_POINT ( 'NONE',  ( -70.26294730757642526, -45.76915084690816826, 5.963676894908396697 ) ) ;
#11736=CARTESIAN_POINT ( 'NONE',  ( 36.49301456553985190, -3.557456006871358323, 5.797608776528274888 ) ) ;
#11740=CARTESIAN_POINT ( 'NONE',  ( -12.99139449055068241, -10.90558813203967148, -6.000000000000000000 ) ) ;
#11743=CARTESIAN_POINT ( 'NONE',  ( -72.11798225935933715, 5.092045952281377907, -9.929846635402185484 ) ) ;
#11747=B_SPLINE_CURVE_WITH_KNOTS ( 'NONE', 3,
 ( #3248, #24619, #21955, #15966, #27905, #37988, #338, #18851, #12878, #31424, #3040, #15558, #21547, #6302, #9584, #12471, #15767, #37173, #9789, #25442, #28323, #139, #12670, #25245 ),
 .UNSPECIFIED., .F., .F.,
 ( 4, 2, 2, 2, 1, 1, 2, 2, 2, 2, 2, 2, 4 ),
 ( 0.000000000000000000, 0.2499999999999828471, 0.3749999999999742428, 0.4374999999999711342, 0.4687499999999695799, 0.4843749999999687472, 0.4921874999999684142, 0.4999999999999680256, 0.6249999999999711342, 0.6874999999999725775, 0.7187499999999753530, 0.7499999999999780176, 1.000000000000000000 ),
 .UNSPECIFIED. ) ;
#11752=CARTESIAN_POINT ( 'NONE',  ( 22.88444072573192400, 4.292063183685437266, 3.118239780378390780 ) ) ;
#11758=CARTESIAN_POINT ( 'NONE',  ( 26.06763236307823561, 0.7305744058604376479, 4.422384865831292977 ) ) ;
#11767=CARTESIAN_POINT ( 'NONE',  ( 32.32438508616473882, -2.203219671913323019, -5.968588774572396893 ) ) ;
#11768=EDGE_CURVE ( 'NONE', #1778, #17373, #16799, .T. ) ;
#11769=CARTESIAN_POINT ( 'NONE',  ( 14.61802081865031688, -4.584994529579697442, -2.500000000000000444 ) ) ;
#11772=CARTESIAN_POINT ( 'NONE',  ( 26.70586447420738807, 0.9595633775789119690, -4.381173435910611147 ) ) ;
#11779=CARTESIAN_POINT ( 'NONE',  ( 35.67318982790884974, -1.412481467646560462, -5.626421653071801643 ) ) ;
#11783=PRODUCT ( 'Heavy Cast Steel Frame Chassis', 'Heavy Cast Steel Frame Chassis', '', ( #27070 ) ) ;
#11785=CARTESIAN_POINT ( 'NONE',  ( -72.84815947045233031, 2.429809908889422498, 10.96147798754374669 ) ) ;
#11802=CARTESIAN_POINT ( 'NONE',  ( 21.98862019667479828, 5.618512022731773747, 3.087214410704674172 ) ) ;
#11805=CARTESIAN_POINT ( 'NONE',  ( 22.14748389186037159, -3.079134181252381808, 3.566341549651656617 ) ) ;
#11809=CARTESIAN_POINT ( 'NONE',  ( 16.92333532088173698, 7.515569096285618755, -3.484773916740906863 ) ) ;
#11813=DIRECTION ( 'NONE',  ( 0.000000000000000000, -0.000000000000000000, -1.000000000000000000 ) ) ;
#11817=CARTESIAN_POINT ( 'NONE',  ( 21.85643539959776760, -1.193669045901033066, -12.68912657263372346 ) ) ;
#11819=CARTESIAN_POINT ( 'NONE',  ( -79.06493839038353144, 10.34607662704177145, 5.825634118554894769 ) ) ;
#11820=DIRECTION ( 'NONE',  ( -0.000000000000000000, -0.000000000000000000, -1.000000000000000000 ) ) ;
#11822=CARTESIAN_POINT ( 'NONE',  ( -73.26201557575831202, 7.663664970033887691, -9.727200596108295017 ) ) ;
#11827=CARTESIAN_POINT ( 'NONE',  ( 15.02955287353362124, 11.88006370660428246, 2.552123235661551526 ) ) ;
#11831=EDGE_CURVE ( 'NONE', #4684, #4341, #38385, .T. ) ;
#11838=CARTESIAN_POINT ( 'NONE',  ( 24.67315655365684890, 2.664633189631731458, -3.911906493327204526 ) ) ;
#11843=CARTESIAN_POINT ( 'NONE',  ( 20.42597344558877026, 3.670373271656663938, 3.394365178855436760 ) ) ;
#11846=CARTESIAN_POINT ( 'NONE',  ( 85.98118993947397826, 1.447477879098551856, 5.565446759936045318 ) ) ;
#11849=CARTESIAN_POINT ( 'NONE',  ( -71.05898624497616822, -21.78299143688729700, 5.999999999999970690 ) ) ;
#11866=PLANE ( 'NONE',  #36757 ) ;
#11868=CARTESIAN_POINT ( 'NONE',  ( 23.72560648584031640, 3.533562144730845844, -3.260337319806162704 ) ) ;
#11872=CARTESIAN_POINT ( 'NONE',  ( 25.20438522764541744, -3.119311913904994515, 5.422531462276817038 ) ) ;
#11873=EDGE_CURVE ( 'NONE', #40686, #21186, #38710, .T. ) ;
#11874=AXIS2_PLACEMENT_3D ( 'NONE', #12203, #21692, #25180 ) ;
#11878=CARTESIAN_POINT ( 'NONE',  ( 88.01214243333713227, -2.271333487497714465, 2.136702053253976885 ) ) ;
#11881=CARTESIAN_POINT ( 'NONE',  ( 25.91700580362422812, 2.564115597501617216, -3.561092020512977907 ) ) ;
#11882=CARTESIAN_POINT ( 'NONE',  ( -72.42837670882109080, -47.01774489676372326, 9.886859966642603581 ) ) ;
#11883=EDGE_CURVE ( 'NONE', #4342, #24169, #949, .T. ) ;
#11886=CARTESIAN_POINT ( 'NONE',  ( 15.23668652445202021, -3.872406382219718335, -2.583925503793695899 ) ) ;
#11888=CARTESIAN_POINT ( 'NONE',  ( -5.316495087772350026, -32.84709638682603838, -6.000000000000001776 ) ) ;
#11890=CARTESIAN_POINT ( 'NONE',  ( 36.63303770807473825, -3.078030482662974077, 5.923869526346774883 ) ) ;
#11896=CARTESIAN_POINT ( 'NONE',  ( 32.06975058867338646, 0.2538586514417362494, 4.725460599369140091 ) ) ;
#11897=CARTESIAN_POINT ( 'NONE',  ( 30.19003827612802482, -2.952522945788203845, 4.918283640461378781 ) ) ;
#11909=CARTESIAN_POINT ( 'NONE',  ( 22.26456873610839438, 2.506020883773357966, 5.102889090039424147 ) ) ;
#11910=CARTESIAN_POINT ( 'NONE',  ( 21.44604159357209383, 7.932351888401207418, -2.756240841243536188 ) ) ;
#11918=CARTESIAN_POINT ( 'NONE',  ( 86.16949904519324832, 1.568053417999200505, -4.594337618669723788 ) ) ;
#11919=CARTESIAN_POINT ( 'NONE',  ( -58.92473026143653669, 13.37661300689600274, 2.500000000000000000 ) ) ;
#11922=CARTESIAN_POINT ( 'NONE',  ( 24.44644773797692494, 2.805227876606543713, -3.838340539723811062 ) ) ;
#11923=VERTEX_POINT ( 'NONE', #16561 ) ;
#11924=CARTESIAN_POINT ( 'NONE',  ( 21.85643539959774273, 11.87467848218428834, -0.9583437110454642305 ) ) ;
#11930=CARTESIAN_POINT ( 'NONE',  ( 86.67773139875836819, 0.9971827163122055637, 5.329716871657868005 ) ) ;
#11933=CARTESIAN_POINT ( 'NONE',  ( -80.91065676098010329, -6.597313057213482601, -0.5950503846463383040 ) ) ;
#11937=VECTOR ( 'NONE', #33533, 1000.000000000000000 ) ;
#11939=CARTESIAN_POINT ( 'NONE',  ( 36.98002556809775854, -2.957261013591625520, -5.978025373836474365 ) ) ;
#11944=CARTESIAN_POINT ( 'NONE',  ( -70.73213213501304608, -45.61702805680359063, 6.000000000000001776 ) ) ;
#11945=ORIENTED_EDGE ( 'NONE', *, *, #27413, .T. ) ;
#11946=CARTESIAN_POINT ( 'NONE',  ( 35.70145850010435140, -1.358481403853448732, 5.583794832904679595 ) ) ;
#11951=CARTESIAN_POINT ( 'NONE',  ( -7.890026461918812295, -6.626103207857777159E-16, 6.000000000000000000 ) ) ;
#11955=CARTESIAN_POINT ( 'NONE',  ( 0.000000000000000000, 13.37661300689600097, 6.000000000000000000 ) ) ;
#11958=CARTESIAN_POINT ( 'NONE',  ( 22.21046374329029405, 5.169589464359284570, 3.137441446710924620 ) ) ;
#11960=CARTESIAN_POINT ( 'NONE',  ( -4.266520354791871306, -48.67644278316300444, 6.000000000000000000 ) ) ;
#11972=CARTESIAN_POINT ( 'NONE',  ( -17.69482985384421880, -29.56993018339339940, 6.000000000000000000 ) ) ;
#11973=ORIENTED_EDGE ( 'NONE', *, *, #3214, .F. ) ;
#11978=CARTESIAN_POINT ( 'NONE',  ( 29.24730582455742578, -0.4004845594861357605, -5.905559009470326970 ) ) ;
#11979=CARTESIAN_POINT ( 'NONE',  ( 14.70571656306172237, -5.036098275607509223, -2.499999999999940492 ) ) ;
#11983=DIRECTION ( 'NONE',  ( 0.000000000000000000, 0.000000000000000000, -1.000000000000000000 ) ) ;
#11986=EDGE_CURVE ( 'NONE', #17221, #10017, #17817, .T. ) ;
#11988=CARTESIAN_POINT ( 'NONE',  ( 37.13786913975418713, -2.596535722758734011, -5.986194934020763192 ) ) ;
#11996=CARTESIAN_POINT ( 'NONE',  ( 21.42317272044189735, 8.032848918686916306, 2.736807373248377750 ) ) ;
#11997=CARTESIAN_POINT ( 'NONE',  ( 23.80152365654308610, 2.314069967681273710, -4.322128912501145948 ) ) ;
#12002=VECTOR ( 'NONE', #38758, 1000.000000000000000 ) ;
#12007=DIRECTION ( 'NONE',  ( 1.000000000000000000, 0.000000000000000000, 0.000000000000000000 ) ) ;
#12013=CARTESIAN_POINT ( 'NONE',  ( 22.18530337611392511, 5.286255035602901664, 3.058813682531833500 ) ) ;
#12015=CARTESIAN_POINT ( 'NONE',  ( 22.14520323347436204, -3.079061112527371247, 3.566016265539754482 ) ) ;
#12022=DIRECTION ( 'NONE',  ( -0.000000000000000000, 0.000000000000000000, 1.000000000000000000 ) ) ;
#12024=CARTESIAN_POINT ( 'NONE',  ( 21.85643539959777470, 6.775053487808889940, 8.548204544396675431 ) ) ;
#12026=CARTESIAN_POINT ( 'NONE',  ( -78.25131871557718455, 11.30516684399499816, 6.821579343738465084 ) ) ;
#12031=EDGE_CURVE ( 'NONE', #5730, #18458, #5850, .T. ) ;
#12032=CARTESIAN_POINT ( 'NONE',  ( 28.28109443870617312, -3.657712271061086540, -4.586391589056719731 ) ) ;
#12033=CARTESIAN_POINT ( 'NONE',  ( 32.06979358023967563, 0.2538423115740326419, -4.725469285452410517 ) ) ;
#12035=CARTESIAN_POINT ( 'NONE',  ( 15.64340809456564152, 11.14027857853738013, 2.614319631236162511 ) ) ;
#12040=CARTESIAN_POINT ( 'NONE',  ( 18.45497827215059772, 13.28099812781043276, -2.500000000000000000 ) ) ;
#12041=CARTESIAN_POINT ( 'NONE',  ( 36.94473691932590498, -2.175944540167862762, -5.891203402125550603 ) ) ;
#12042=CARTESIAN_POINT ( 'NONE',  ( 24.47644591641656220, 2.965209954150327842, -3.650517593455100407 ) ) ;
#12045=CARTESIAN_POINT ( 'NONE',  ( 35.33694189094937599, -3.445746785322538308, 5.711001300648953283 ) ) ;
#12049=CARTESIAN_POINT ( 'NONE',  ( 84.83925925549863223, 2.817044135119172399, -2.844581780382558378 ) ) ;
#12050=CARTESIAN_POINT ( 'NONE',  ( -71.72841970756384455, -21.39719814140381615, 5.947160319466099132 ) ) ;
#12051=CARTESIAN_POINT ( 'NONE',  ( 34.16812880522524409, -3.144588050804470125, -5.539160878010015665 ) ) ;
#12053=ORIENTED_EDGE ( 'NONE', *, *, #28783, .T. ) ;
#12074=CARTESIAN_POINT ( 'NONE',  ( 24.52423802077814585, -6.127131655257791465, 2.764126198674226931 ) ) ;
#12077=CARTESIAN_POINT ( 'NONE',  ( 24.34606147761258654, 3.138786336531333099, -3.389104778623087455 ) ) ;
#12081=CARTESIAN_POINT ( 'NONE',  ( 24.03893326528611141, 2.664202206450044130, -5.290213626918107259 ) ) ;
#12082=CARTESIAN_POINT ( 'NONE',  ( 20.30405589181014747, 6.129815107149093834, 3.484773800364461938 ) ) ;
#12086=CARTESIAN_POINT ( 'NONE',  ( 86.42019152727894493, 0.2271775462534226520, 6.017476335466618309 ) ) ;
#12087=CARTESIAN_POINT ( 'NONE',  ( 15.06184329234986663, 12.12621205208998987, 2.536020854430098836 ) ) ;
#12096=EDGE_LOOP ( 'NONE', ( #15293, #24510, #10450, #29370, #15732, #20483, #38020, #7661, #34594, #15314, #28070, #18705, #36792, #26521, #26071, #9746, #21794, #20028 ) ) ;
#12097=CARTESIAN_POINT ( 'NONE',  ( 37.04568408393004830, -2.800967617106917551, 5.988272973189237902 ) ) ;
#12099=CARTESIAN_POINT ( 'NONE',  ( 85.94962389285764459, 1.815027625006768730, -4.252598035848374813 ) ) ;
#12102=CARTESIAN_POINT ( 'NONE',  ( 36.87190381947284123, -2.085833083560729051, 5.863581891243574873 ) ) ;
#12103=CARTESIAN_POINT ( 'NONE',  ( 23.67457366230596705, -2.672207667981083112, 3.901387810367294762 ) ) ;
#12104=CARTESIAN_POINT ( 'NONE',  ( 21.39126609848262817, -3.058903647210607701, -3.458430474917000286 ) ) ;
#12107=AXIS2_PLACEMENT_3D ( 'NONE', #39596, #21284, #2366 ) ;
#12116=CARTESIAN_POINT ( 'NONE',  ( 22.91664155360341937, 2.744262553797580217, 4.428644351404614987 ) ) ;
#12117=CARTESIAN_POINT ( 'NONE',  ( 31.38403718649578877, 0.5068638959182734105, 4.596961181239236360 ) ) ;
#12119=EDGE_CURVE ( 'NONE', #39349, #38890, #21443, .T. ) ;
#12126=CYLINDRICAL_SURFACE ( 'NONE', #805, 8.080217238368755162 ) ;
#12130=CARTESIAN_POINT ( 'NONE',  ( 22.85242861330229047, 3.166249937094171685, -4.146800157721144409 ) ) ;
#12134=CARTESIAN_POINT ( 'NONE',  ( 21.85643539959772497, -14.97654459006671068, 3.851724272136834326 ) ) ;
#12140=CARTESIAN_POINT ( 'NONE',  ( 88.43294427370824451, -0.9743556922601576131, -2.623293804462837553 ) ) ;
#12145=CARTESIAN_POINT ( 'NONE',  ( 18.25296777573797513, -2.941843506369077321, 3.053268232905335555 ) ) ;
#12146=CARTESIAN_POINT ( 'NONE',  ( 25.01091293555841233, 3.329590545877085805, 1.936828124349011526 ) ) ;
#12147=CARTESIAN_POINT ( 'NONE',  ( 37.04431342567128382, -2.893185755689349214, -5.988059048818550778 ) ) ;
#12152=B_SPLINE_CURVE_WITH_KNOTS ( 'NONE', 3,
 ( #36516, #30550, #14879, #15297, #2362, #2771, #39382, #1954, #23745, #17759, #30346, #2152, #11577, #5634 ),
 .UNSPECIFIED., .F., .F.,
 ( 4, 2, 2, 2, 2, 2, 4 ),
 ( 0.007044848506661660799, 0.007338175092571547382, 0.007631501678481433099, 0.007924828264391319682, 0.008218154850301206266, 0.008804808022120993310, 0.009391461193940780355 ),
 .UNSPECIFIED. ) ;
#12156=CARTESIAN_POINT ( 'NONE',  ( 27.78114228934722618, 1.798550533532914830, 4.024392981447666884 ) ) ;
#12158=ORIENTED_EDGE ( 'NONE', *, *, #25933, .T. ) ;
#12163=VERTEX_POINT ( 'NONE', #14624 ) ;
#12165=CARTESIAN_POINT ( 'NONE',  ( 88.35472856589244373, -0.8865000968999163788, -0.8281635480601134969 ) ) ;
#12167=CARTESIAN_POINT ( 'NONE',  ( -71.85905498853752249, 3.863100500280893357, -9.956904411795710175 ) ) ;
#12172=LINE ( 'NONE', #12583, #21223 ) ;
#12174=CARTESIAN_POINT ( 'NONE',  ( 23.14578216353262263, 3.986807833658514877, 3.175358570212865938 ) ) ;
#12178=EDGE_CURVE ( 'NONE', #16241, #8875, #22236, .T. ) ;
#12188=ORIENTED_EDGE ( 'NONE', *, *, #9670, .F. ) ;
#12190=ORIENTED_EDGE ( 'NONE', *, *, #25306, .T. ) ;
#12193=CARTESIAN_POINT ( 'NONE',  ( -70.92837670882107659, -47.11702805680359063, 38.00000000000000711 ) ) ;
#12195=CARTESIAN_POINT ( 'NONE',  ( 28.53445731760455573, 0.6922391713037714389, -5.301755952056612209 ) ) ;
#12199=CARTESIAN_POINT ( 'NONE',  ( 24.12590274031893856, 0.5209382751000486422, -5.092299414582193151 ) ) ;
#12203=CARTESIAN_POINT ( 'NONE',  ( -4.444218661349752963, -35.94265729135299381, 2.500000000000000000 ) ) ;
#12206=CARTESIAN_POINT ( 'NONE',  ( 36.10477245413083836, -1.582022789005378849, -5.680924181711803911 ) ) ;
#12216=CARTESIAN_POINT ( 'NONE',  ( 25.04641388788620304, 2.159341827801565028, -4.144791871881564838 ) ) ;
#12228=CARTESIAN_POINT ( 'NONE',  ( 22.38229058954441797, 4.940558714326160228, 3.046107694943288813 ) ) ;
#12229=EDGE_CURVE ( 'NONE', #30583, #16084, #8181, .T. ) ;
#12242=CARTESIAN_POINT ( 'NONE',  ( 21.85643539959776760, 7.937350203533870996, 6.559150378249414715 ) ) ;
#12244=CARTESIAN_POINT ( 'NONE',  ( -75.05519143552835715, 9.687648905246064146, 9.110330305801273454 ) ) ;
#12245=CARTESIAN_POINT ( 'NONE',  ( 36.65806048341712398, -3.481436136677176219, 5.844384006794087760 ) ) ;
#12247=ORIENTED_EDGE ( 'NONE', *, *, #5099, .F. ) ;
#12249=CARTESIAN_POINT ( 'NONE',  ( 30.69560960875148581, -3.339038624481136974, -4.972551620578038012 ) ) ;
#12250=CARTESIAN_POINT ( 'NONE',  ( 32.07043626334714759, 0.2549077454616246463, -4.723733316502016777 ) ) ;
#12252=CARTESIAN_POINT ( 'NONE',  ( 15.42605057732512819, 10.99993330764380950, 2.614006291671366444 ) ) ;
#12254=CARTESIAN_POINT ( 'NONE',  ( 29.66582406763757618, -3.796006116354329052, 4.435324138597246169 ) ) ;
#12257=CARTESIAN_POINT ( 'NONE',  ( 22.66896291849731071, 0.3171684538786420648, -6.422044740241496186 ) ) ;
#12258=CARTESIAN_POINT ( 'NONE',  ( 36.82054380567017660, -2.045509829724917683, -5.849054631016336714 ) ) ;
#12259=CARTESIAN_POINT ( 'NONE',  ( 26.12442444200497249, 1.901572713601228148, -4.234468824312982882 ) ) ;
#12264=CARTESIAN_POINT ( 'NONE',  ( 36.91763012405728972, -3.049005243583072566, 5.968287055754437631 ) ) ;
#12268=CARTESIAN_POINT ( 'NONE',  ( 86.36811837411410409, 0.9377611381114191458, -5.884791073222536362 ) ) ;
#12269=CARTESIAN_POINT ( 'NONE',  ( 33.14263624204154723, -3.231821542972313388, 5.586707398679605419 ) ) ;
#12270=CARTESIAN_POINT ( 'NONE',  ( 21.71197053136906163, 6.328941705067348877, 3.193005318136709736 ) ) ;
#12272=CARTESIAN_POINT ( 'NONE',  ( 24.50294889293943257, 2.766753032866218653, 3.859934611448354591 ) ) ;
#12273=DIRECTION ( 'NONE',  ( 0.000000000000000000, -0.000000000000000000, -1.000000000000000000 ) ) ;
#12277=ADVANCED_FACE ( 'NONE', ( #7902 ), #23558, .F. ) ;
#12278=ORIENTED_EDGE ( 'NONE', *, *, #34628, .F. ) ;
#12291=CARTESIAN_POINT ( 'NONE',  ( 33.89725028478159174, -5.465908938576614418, 0.4877600842561391481 ) ) ;
#12292=AXIS2_PLACEMENT_3D ( 'NONE', #34002, #8643, #6342 ) ;
#12293=CARTESIAN_POINT ( 'NONE',  ( 24.64255241942672114, 2.987807242327306767, -3.517570117124183771 ) ) ;
#12297=CARTESIAN_POINT ( 'NONE',  ( 25.36335546794393281, -3.584835346285432767, 4.690180580146940059 ) ) ;
#12298=CARTESIAN_POINT ( 'NONE',  ( -80.88559923893718917, -5.699916044423376960, -1.011431130875308337 ) ) ;
#12301=CARTESIAN_POINT ( 'NONE',  ( 86.54108089765607303, -0.3148381559440514010, -5.858094985366312457 ) ) ;
#12307=FACE_BOUND ( 'NONE', #9229, .T. ) ;
#12308=CARTESIAN_POINT ( 'NONE',  ( 14.98150154961487068, -6.080694961501129647, -2.528993159681567793 ) ) ;
#12313=CARTESIAN_POINT ( 'NONE',  ( 36.63332213572625307, -3.079482314827179934, 5.923913918160702785 ) ) ;
#12314=EDGE_CURVE ( 'NONE', #27368, #7875, #4627, .T. ) ;
#12315=CARTESIAN_POINT ( 'NONE',  ( 87.00024757794628272, 0.6349172363070331171, 4.931108601852515427 ) ) ;
#12319=CARTESIAN_POINT ( 'NONE',  ( 22.17363360563139452, -2.652663328054713165, 3.667129814150781097 ) ) ;
#12320=CARTESIAN_POINT ( 'NONE',  ( -69.79768788248055955, -46.12641766718275704, 9.936119964364207746 ) ) ;
#12321=AXIS2_PLACEMENT_3D ( 'NONE', #32425, #19456, #32029 ) ;
#12323=VECTOR ( 'NONE', #8667, 1000.000000000000000 ) ;
#12324=ORIENTED_EDGE ( 'NONE', *, *, #24891, .T. ) ;
#12325=CARTESIAN_POINT ( 'NONE',  ( 27.29202159548859896, -4.463074182346106866, -3.652272488581413512 ) ) ;
#12333=CARTESIAN_POINT ( 'NONE',  ( 22.89135895909411644, 2.899355188632806613, 4.326634353261504806 ) ) ;
#12334=CARTESIAN_POINT ( 'NONE',  ( 33.57045594063073679, -0.3384725396225634619, 5.045718172883097097 ) ) ;
#12340=CARTESIAN_POINT ( 'NONE',  ( 86.03410341386039306, 1.720136217376576848, -4.402104626801674137 ) ) ;
#12345=CARTESIAN_POINT ( 'NONE',  ( 23.05884816843563456, 3.162798540487469001, -4.037182842946084982 ) ) ;
#12346=ORIENTED_EDGE ( 'NONE', *, *, #12696, .T. ) ;
#12349=CARTESIAN_POINT ( 'NONE',  ( 21.85643539959774984, 9.043776176932434296, -7.298091200098202336 ) ) ;
#12354=CARTESIAN_POINT ( 'NONE',  ( 85.61973765214487742, 2.185571507920985646, -3.964146163151171187 ) ) ;
#12359=CARTESIAN_POINT ( 'NONE',  ( 19.71439828684868445, -2.982188169833531521, 3.242426474250064583 ) ) ;
#12361=CARTESIAN_POINT ( 'NONE',  ( 20.48006656716360041, 3.803899341377876109, -3.402807718724278452 ) ) ;
#12365=EDGE_CURVE ( 'NONE', #9599, #2897, #10461, .T. ) ;
#12373=CARTESIAN_POINT ( 'NONE',  ( 33.94504222670371973, -0.4898145577208962709, 5.123711933742746361 ) ) ;
#12379=CARTESIAN_POINT ( 'NONE',  ( 88.35188732102578513, -0.8833086758121115878, 0.5115122137427119409 ) ) ;
#12380=CARTESIAN_POINT ( 'NONE',  ( -73.10036559450711025, 7.400480790150822941, -9.764070703836081222 ) ) ;
#12386=CARTESIAN_POINT ( 'NONE',  ( 23.73355850457707206, 3.546588217239842411, 3.226370594130565816 ) ) ;
#12391=ORIENTED_EDGE ( 'NONE', *, *, #7991, .F. ) ;
#12396=CARTESIAN_POINT ( 'NONE',  ( 18.58232099604030552, 8.030589776515261846, -3.022115281584475621 ) ) ;
#12405=CARTESIAN_POINT ( 'NONE',  ( 14.69558838330753581, -65.19654454972992141, 2.500000000000000444 ) ) ;
#12406=CARTESIAN_POINT ( 'NONE',  ( 30.73735125564872916, -2.095387222228427770, 5.934458408524426076 ) ) ;
#12409=CARTESIAN_POINT ( 'NONE',  ( 24.72159449605993231, 0.6340518189776346292, -4.784391175910871929 ) ) ;
#12412=CARTESIAN_POINT ( 'NONE',  ( -7.890026461918810519, -29.56993018339340651, 6.000000000000000000 ) ) ;
#12413=DIRECTION ( 'NONE',  ( 1.000000000000000000, 0.000000000000000000, 0.000000000000000000 ) ) ;
#12414=EDGE_CURVE ( 'NONE', #40359, #5482, #26844, .T. ) ;
#12415=CARTESIAN_POINT ( 'NONE',  ( 33.91388920362712867, -0.5462387119675344849, -5.194274413794256695 ) ) ;
#12417=CARTESIAN_POINT ( 'NONE',  ( 32.21384408659537968, -3.775819508426534465, 4.843400441209068319 ) ) ;
#12420=CARTESIAN_POINT ( 'NONE',  ( 8.290806648384990041, -33.63722727088462250, 2.499999999999998668 ) ) ;
#12424=AXIS2_PLACEMENT_3D ( 'NONE', #21032, #17920, #2107 ) ;
#12426=CARTESIAN_POINT ( 'NONE',  ( -80.92837670882107659, 2.429809908903242555, -12.50000000000000000 ) ) ;
#12438=CARTESIAN_POINT ( 'NONE',  ( 24.41077649390761550, 3.166270396914395935, 3.259050073679078618 ) ) ;
#12443=CARTESIAN_POINT ( 'NONE',  ( 22.07198986276520714, 0.3265494727465731439, 7.434200068064451550 ) ) ;
#12451=CARTESIAN_POINT ( 'NONE',  ( 21.85643539959775694, 1.480681348264278219, 12.33944218828100325 ) ) ;
#12454=CARTESIAN_POINT ( 'NONE',  ( -72.84051408678523387, 2.240445720093386051, 10.96224446246069206 ) ) ;
#12455=CARTESIAN_POINT ( 'NONE',  ( 36.72314012181375631, -3.448745041943457323, 5.863009582911698381 ) ) ;
#12457=DIRECTION ( 'NONE',  ( 0.000000000000000000, 0.000000000000000000, 1.000000000000000000 ) ) ;
#12458=CARTESIAN_POINT ( 'NONE',  ( -80.90861860399087391, 11.45717611192839591, 0.6283086135788882309 ) ) ;
#12460=CARTESIAN_POINT ( 'NONE',  ( 4.200390093233091093, -29.56993018339339940, -6.000000000000000000 ) ) ;
#12461=CARTESIAN_POINT ( 'NONE',  ( 36.44575679768344401, -1.731622218426172921, -5.730272923922282935 ) ) ;
#12463=CARTESIAN_POINT ( 'NONE',  ( 22.07127107929524357, 4.795919128869573278, 3.651153666268970532 ) ) ;
#12470=CARTESIAN_POINT ( 'NONE',  ( 23.61265236088880215, 0.4553577143438285457, -5.501100469002734528 ) ) ;
#12471=CARTESIAN_POINT ( 'NONE',  ( 31.69270225732497082, -3.760796806013388505, -4.741932875280792103 ) ) ;
#12473=CARTESIAN_POINT ( 'NONE',  ( 24.36839190658592358, 2.936743033212012577, -3.728160028041425988 ) ) ;
#12476=CARTESIAN_POINT ( 'NONE',  ( 33.67582729204764291, -3.265305600472629077, 5.462325320484106683 ) ) ;
#12480=CARTESIAN_POINT ( 'NONE',  ( 88.08925887309592895, -2.022426073114577338, 2.982665067064442788 ) ) ;
#12482=CARTESIAN_POINT ( 'NONE',  ( 35.96707384839896093, -3.154842221623805454, -5.819929759647552991 ) ) ;
#12484=VERTEX_POINT ( 'NONE', #2569 ) ;
#12485=CARTESIAN_POINT ( 'NONE',  ( 25.64725611152496398, 2.152986409533134804, 4.135202000189527993 ) ) ;
#12496=VERTEX_POINT ( 'NONE', #38134 ) ;
#12501=CARTESIAN_POINT ( 'NONE',  ( 21.71676751225188795, 6.286869429030311984, -3.207926565813705277 ) ) ;
#12504=CARTESIAN_POINT ( 'NONE',  ( -76.99182769667817183, -4.628834071841179565, -9.484053338739713013 ) ) ;
#12507=CARTESIAN_POINT ( 'NONE',  ( 85.98972789526511917, 0.6168376674493800671, -5.987237289632960646 ) ) ;
#12511=CARTESIAN_POINT ( 'NONE',  ( 22.07069217792962590, 4.357467706526993112, -1.544973507881162167 ) ) ;
#12513=AXIS2_PLACEMENT_3D ( 'NONE', #21231, #23893, #26996 ) ;
#12518=CARTESIAN_POINT ( 'NONE',  ( 27.40535003225689792, 0.9587719845282556275, 4.483665692065598840 ) ) ;
#12520=CARTESIAN_POINT ( 'NONE',  ( 86.92636418897033934, 0.7179065655219835085, -4.964803926638174048 ) ) ;
#12525=CARTESIAN_POINT ( 'NONE',  ( 14.77277131670251364, 13.03059887336277356, -2.498940285545853346 ) ) ;
#12526=ORIENTED_EDGE ( 'NONE', *, *, #23701, .F. ) ;
#12528=CARTESIAN_POINT ( 'NONE',  ( 27.53908758452205419, -4.370590091868444382, -3.734973139623710026 ) ) ;
#12530=CARTESIAN_POINT ( 'NONE',  ( -79.80088323097261593, 11.50896648099637432, 4.631886560738033509 ) ) ;
#12532=EDGE_LOOP ( 'NONE', ( #20558, #31342 ) ) ;
#12534=CARTESIAN_POINT ( 'NONE',  ( 35.93061354739079150, -3.156855339584533127, 5.814239247879517514 ) ) ;
#12535=ORIENTED_EDGE ( 'NONE', *, *, #22799, .F. ) ;
#12537=CARTESIAN_POINT ( 'NONE',  ( 23.58159892518875012, 2.786089680335510188, 4.075354304694349672 ) ) ;
#12538=CARTESIAN_POINT ( 'NONE',  ( 36.01495275453719813, -1.469146332022411405, 5.615055713102431234 ) ) ;
#12544=CARTESIAN_POINT ( 'NONE',  ( 86.51911666896515385, 1.175346309125120836, -4.933042343133747565 ) ) ;
#12545=DIRECTION ( 'NONE',  ( 1.000000000000000000, 0.000000000000000000, 0.000000000000000000 ) ) ;
#12549=CARTESIAN_POINT ( 'NONE',  ( 22.22094290343520839, 3.703924387003111995, -4.206398560386165109 ) ) ;
#12551=CARTESIAN_POINT ( 'NONE',  ( 21.85643539959779602, 6.788858854521340191, -12.70575755685024610 ) ) ;
#12553=VERTEX_POINT ( 'NONE', #25184 ) ;
#12556=CARTESIAN_POINT ( 'NONE',  ( 87.18644375116411993, 0.4257728571452945587, -5.011944538332810062 ) ) ;
#12558=VECTOR ( 'NONE', #5693, 1000.000000000000114 ) ;
#12559=CARTESIAN_POINT ( 'NONE',  ( 14.77222812468949620, 12.33286846116140190, 2.511961485181804843 ) ) ;
#12560=CARTESIAN_POINT ( 'NONE',  ( 14.82260051658036559, -5.954777973940915459, 2.519088763667999498 ) ) ;
#12562=CARTESIAN_POINT ( 'NONE',  ( 35.33511103386211971, -3.172769356962385601, -5.721296678360661581 ) ) ;
#12570=VERTEX_POINT ( 'NONE', #22315 ) ;
#12572=CARTESIAN_POINT ( 'NONE',  ( 36.44417780280348040, -1.734285983370489781, 5.731955937638065990 ) ) ;
#12575=CARTESIAN_POINT ( 'NONE',  ( 87.73256103596717992, -2.278636154477776454, -2.442743118526013557 ) ) ;
#12576=ADVANCED_FACE ( 'NONE', ( #34683 ), #6458, .F. ) ;
#12577=EDGE_LOOP ( 'NONE', ( #35836, #25705, #32115, #7112, #28957 ) ) ;
#12581=EDGE_LOOP ( 'NONE', ( #18524, #8807 ) ) ;
#12583=CARTESIAN_POINT ( 'NONE',  ( -58.92473026143653669, 13.37661300689600274, 2.500000000000000000 ) ) ;
#12584=ORIENTED_EDGE ( 'NONE', *, *, #22230, .T. ) ;
#12585=CARTESIAN_POINT ( 'NONE',  ( 22.62710517823844114, 4.569975501755447311, 3.100331212370438294 ) ) ;
#12591=CARTESIAN_POINT ( 'NONE',  ( -71.91909284412787429, -45.98648324524150865, 5.918062715858019018 ) ) ;
#12593=CARTESIAN_POINT ( 'NONE',  ( 18.30399930829332789, 7.732246112693302642, -3.063179794592037375 ) ) ;
#12607=CARTESIAN_POINT ( 'NONE',  ( 28.57954844588206811, 0.5947805351201630453, 5.396286122280502084 ) ) ;
#12616=CARTESIAN_POINT ( 'NONE',  ( 34.60566713630616675, -0.8402458443559904788, -5.339578216116290577 ) ) ;
#12623=CARTESIAN_POINT ( 'NONE',  ( 21.88052003412104440, -13.33610013990758247, 2.500000000000000444 ) ) ;
#12632=CARTESIAN_POINT ( 'NONE',  ( 22.42221550662346630, 3.548445137936078186, 4.163436039515404197 ) ) ;
#12635=CIRCLE ( 'NONE', #22535, 21.28220113893567245 ) ;
#12638=CARTESIAN_POINT ( 'NONE',  ( 21.71101792114980000, 6.337217689991505587, 3.190087676312844955 ) ) ;
#12639=CARTESIAN_POINT ( 'NONE',  ( 17.98299319363433924, -3.166408508134356925, 2.970447345965724573 ) ) ;
#12644=CARTESIAN_POINT ( 'NONE',  ( 21.80387297355334653, 0.2465413692211569363, 8.289364210318115767 ) ) ;
#12651=CARTESIAN_POINT ( 'NONE',  ( 21.85643539959781023, -9.626920734992143736, 7.250399157909895642 ) ) ;
#12654=CARTESIAN_POINT ( 'NONE',  ( -73.13416264966082281, 4.597384000621623557, 10.93019976426635154 ) ) ;
#12660=CARTESIAN_POINT ( 'NONE',  ( 20.92045457785759410, 4.581795454354830710, -2.649697436696578645 ) ) ;
#12663=CARTESIAN_POINT ( 'NONE',  ( 17.61160109935129370, 8.414362448292965979, 2.955114308372669196 ) ) ;
#12665=CARTESIAN_POINT ( 'NONE',  ( 30.11812385294796002, -3.708574960581302982, 4.582163967512324021 ) ) ;
#12668=CARTESIAN_POINT ( 'NONE',  ( -80.92837670882107659, 2.429809908903242555, -12.50000000000000000 ) ) ;
#12669=CARTESIAN_POINT ( 'NONE',  ( 23.59088344076351973, 0.9244265036794051538, -5.301842884707729020 ) ) ;
#12670=CARTESIAN_POINT ( 'NONE',  ( 33.05009345505028051, -3.812300322207410996, -5.013107131247908299 ) ) ;
#12671=CARTESIAN_POINT ( 'NONE',  ( 24.94694396431675187, 2.517674699171826624, -3.979827897743033471 ) ) ;
#12674=CARTESIAN_POINT ( 'NONE',  ( 20.48007155163331205, 3.803897258032066908, 3.402808496671325678 ) ) ;
#12677=CARTESIAN_POINT ( 'NONE',  ( 85.11033487576473533, 2.122656363318763173, 4.626068480629312418 ) ) ;
#12678=FACE_OUTER_BOUND ( 'NONE', #33567, .T. ) ;
#12681=CARTESIAN_POINT ( 'NONE',  ( 26.50466346464379086, 1.691181880056894737, 4.311557507100089559 ) ) ;
#12693=CARTESIAN_POINT ( 'NONE',  ( -70.92837670882107659, -37.87473357531881391, 0.000000000000000000 ) ) ;
#12694=VERTEX_POINT ( 'NONE', #38327 ) ;
#12696=EDGE_CURVE ( 'NONE', #24696, #16350, #22715, .T. ) ;
#12702=CARTESIAN_POINT ( 'NONE',  ( 21.99292708584655998, 5.590793479290228518, -3.105521760628916272 ) ) ;
#12712=CARTESIAN_POINT ( 'NONE',  ( 87.82658540711466344, -2.392274210255118216, -1.851534029869310816 ) ) ;
#12719=DIRECTION ( 'NONE',  ( 0.000000000000000000, 0.000000000000000000, -1.000000000000000000 ) ) ;
#12723=CARTESIAN_POINT ( 'NONE',  ( 36.42079407071754815, -3.114107480780474280, 5.890743773605413125 ) ) ;
#12724=CARTESIAN_POINT ( 'NONE',  ( 87.54465900634191655, 0.02340848060778613626, -4.593250482506632260 ) ) ;
#12732=CARTESIAN_POINT ( 'NONE',  ( -71.83276077574569740, 0.9916882426457708233, 9.959148848844533219 ) ) ;
#12738=CARTESIAN_POINT ( 'NONE',  ( 22.04424169242247089, 2.368281942274926166, 5.447058248131960490 ) ) ;
#12739=CARTESIAN_POINT ( 'NONE',  ( 31.10600218134772987, 0.6115860487915156796, 4.541982612545634623 ) ) ;
#12747=CARTESIAN_POINT ( 'NONE',  ( 85.65652580503477509, 2.144249308523916042, -3.546142381197787241 ) ) ;
#12751=CARTESIAN_POINT ( 'NONE',  ( 24.36246139054879833, 2.879672585629011738, -3.789350523822255568 ) ) ;
#12753=CARTESIAN_POINT ( 'NONE',  ( 21.85643539959779957, -10.54057479330554159, -5.012605957032298498 ) ) ;
#12757=CARTESIAN_POINT ( 'NONE',  ( 87.85599567641696694, -0.3262996441500809475, -4.386575958041428080 ) ) ;
#12758=ORIENTED_EDGE ( 'NONE', *, *, #26497, .F. ) ;
#12759=CARTESIAN_POINT ( 'NONE',  ( 10.58508780786439374, 19.59913305159139441, 2.500000000000000000 ) ) ;
#12760=CARTESIAN_POINT ( 'NONE',  ( 33.94050681485320098, -3.428830454661854432, 5.491199649958280027 ) ) ;
#12763=CARTESIAN_POINT ( 'NONE',  ( 36.91076444475422136, -2.639566709576531611, -5.967215500452092591 ) ) ;
#12775=CARTESIAN_POINT ( 'NONE',  ( 37.00880725212909539, -2.250639250997623630, 5.913624440729033260 ) ) ;
#12779=CARTESIAN_POINT ( 'NONE',  ( 88.20160905653106909, -0.7145089964949031813, -2.080387601684223320 ) ) ;
#12786=CARTESIAN_POINT ( 'NONE',  ( 23.15296705429070556, 3.944850500700754825, 3.230105547710554248 ) ) ;
#12790=VECTOR ( 'NONE', #27444, 1000.000000000000000 ) ;
#12797=CARTESIAN_POINT ( 'NONE',  ( 14.71117645488784120, 12.53769967753948578, -2.502432895569043136 ) ) ;
#12800=EDGE_LOOP ( 'NONE', ( #36155, #4073 ) ) ;
#12807=CARTESIAN_POINT ( 'NONE',  ( 17.62552235143947854, 11.92971608769965997, 2.500000000000007550 ) ) ;
#12808=CARTESIAN_POINT ( 'NONE',  ( 29.95345716813442749, -1.222334143750352764, -6.038643835265099291 ) ) ;
#12810=CARTESIAN_POINT ( 'NONE',  ( 19.23685618013880472, -6.968822543817719151, 2.500000000000000444 ) ) ;
#12815=CARTESIAN_POINT ( 'NONE',  ( 36.84678844362374406, -3.231065898219810162, -5.943761196008794379 ) ) ;
#12818=CARTESIAN_POINT ( 'NONE',  ( 23.83223587884036831, -2.668011125867791211, -3.925994812332605388 ) ) ;
#12829=CARTESIAN_POINT ( 'NONE',  ( -70.92837670882107659, -65.19654454972992141, -6.000000000000002665 ) ) ;
#12836=CARTESIAN_POINT ( 'NONE',  ( 21.85231751869008932, 4.115031571714823144, 4.273325978632851907 ) ) ;
#12841=CARTESIAN_POINT ( 'NONE',  ( 23.14138885347819041, 4.047734147674228566, 3.078156626778878469 ) ) ;
#12848=CARTESIAN_POINT ( 'NONE',  ( 27.28763074894343887, 1.166087062639404870, 4.463145202650028232 ) ) ;
#12855=( BOUNDED_SURFACE ( )  B_SPLINE_SURFACE ( 3, 2, ( 
 ( #25679, #31664, #3680 ),
 ( #37814, #12298, #25282 ),
 ( #21992, #31261, #2865 ),
 ( #12913, #3479, #34973 ),
 ( #6550, #24871, #31461 ),
 ( #21786, #9826, #582 ),
 ( #34772, #28570, #377 ),
 ( #22206, #13121, #37410 ),
 ( #16005, #15388, #173 ),
 ( #34364, #9619, #15806 ),
 ( #34570, #9002, #21582 ),
 ( #27943, #31054, #25480 ),
 ( #38025, #9206, #6747 ),
 ( #34164, #6344, #19298 ),
 ( #28775, #40486, #31869 ),
 ( #6134, #5930, #18674 ),
 ( #18893, #3077, #15597 ),
 ( #28149, #40703, #12504 ),
 ( #25079, #37609, #28360 ),
 ( #20287, #32279, #1579 ),
 ( #23194, #32871, #35766 ),
 ( #23393, #4269, #10619 ),
 ( #29373, #26489, #14110 ),
 ( #16792, #1193, #13730 ),
 ( #29571, #32470, #3885 ),
 ( #32672, #7539, #26293 ),
 ( #35959, #1387, #778 ),
 ( #16401, #38223, #4661 ),
 ( #4079, #7740, #13309 ),
 ( #28975, #35171, #25882 ),
 ( #16592, #10020, #38421 ),
 ( #20095, #10222, #6944 ),
 ( #38629, #19506, #17197 ),
 ( #38825, #4473, #29764 ),
 ( #22805, #32081, #16994 ),
 ( #13918, #35375, #39014 ),
 ( #7143, #19704, #10818 ),
 ( #29175, #22603, #984 ),
 ( #13520, #26091, #10427 ),
 ( #23003, #35570, #7339 ),
 ( #19898, #8742, #27087 ),
 ( #36158, #40048, #21326 ),
 ( #2614, #5262, #30173 ),
 ( #33071, #21122, #27285 ),
 ( #11822, #33494, #39850 ),
 ( #17803, #14930, #30809 ),
 ( #30388, #2193, #14711 ),
 ( #18012, #20908, #4856 ),
 ( #33690, #11618, #24197 ),
 ( #24406, #30600, #29970 ),
 ( #36756, #8542, #23594 ),
 ( #20697, #36962, #1784 ),
 ( #17388, #7937, #14312 ),
 ( #5061, #5469, #33901 ),
 ( #20489, #5675, #2409 ),
 ( #8126, #27498, #26882 ),
 ( #39424, #23983, #17594 ),
 ( #18217, #26689, #11214 ),
 ( #39223, #11013, #23780 ),
 ( #36359, #33280, #1995 ),
 ( #8333, #14513, #39634 ),
 ( #11419, #36554, #3238 ),
 ( #34113, #127, #15754 ),
 ( #18839, #2814, #25029 ),
 ( #25431, #15548, #25234 ),
 ( #22360, #37765, #34926 ),
 ( #15954, #31009, #40245 ),
 ( #12458, #6086, #18421 ) ),
 .UNSPECIFIED., .F., .F., .T. ) 
 B_SPLINE_SURFACE_WITH_KNOTS ( ( 4, 2, 2, 2, 2, 2, 2, 2, 2, 2, 2, 2, 2, 2, 2, 2, 2, 2, 2, 2, 2, 2, 2, 2, 2, 2, 2, 2, 2, 2, 2, 2, 2, 4 ),
 ( 3, 3 ),
 ( 0.04252856423674911124, 0.04385758186914752443, 0.04518659950154593069, 0.04651561713394433695, 0.04784463476634275014, 0.05050267003113956960, 0.05116717884733877619, 0.05183168766353797585, 0.05316070529593638905, 0.05382521411213559565, 0.05448972292833480224, 0.05581874056073320850, 0.05648324937693241510, 0.05714775819313161476, 0.05847677582553002795, 0.05980579345792844115, 0.06113481109032684740, 0.06246382872272525366, 0.06379284635512366686, 0.06512186398752208005, 0.06645088161992049325, 0.06777989925231889257, 0.06910891688471730576, 0.07043793451711571896, 0.07176695214951411828, 0.07309596978191253147, 0.07442498741431094467, 0.07575400504670935786, 0.07708302267910777106, 0.07841204031150618425, 0.07974105794390459745, 0.08107007557630301064, 0.08239909320870142384, 0.08505712847349823635 ),
 ( 0.000000000000000000, 1.000000000000000000 ),
 .UNSPECIFIED. ) 
 GEOMETRIC_REPRESENTATION_ITEM ( )  RATIONAL_B_SPLINE_SURFACE ( (
 ( 1.000000000000000000, 0.7442417417348949904, 1.000000000000000000),
 ( 1.000000000000000000, 0.7431783020712605659, 1.000000000000000000),
 ( 1.000000000000000000, 0.7409760979376766032, 1.000000000000000000),
 ( 1.000000000000000000, 0.7345856213530946865, 1.000000000000000000),
 ( 1.000000000000000000, 0.7304004294511651230, 1.000000000000000000),
 ( 1.000000000000000000, 0.7203431566566479427, 1.000000000000000000),
 ( 1.000000000000000000, 0.7144690456092649411, 1.000000000000000000),
 ( 1.000000000000000000, 0.7013913408706143882, 1.000000000000000000),
 ( 1.000000000000000000, 0.6941559842080995413, 1.000000000000000000),
 ( 1.000000000000000000, 0.6719163496680571335, 1.000000000000000000),
 ( 1.000000000000000000, 0.6561249043233500222, 1.000000000000000000),
 ( 1.000000000000000000, 0.6392825574178745418, 1.000000000000000000),
 ( 1.000000000000000000, 0.6360685153987252205, 1.000000000000000000),
 ( 1.000000000000000000, 0.6301773797663908772, 1.000000000000000000),
 ( 1.000000000000000000, 0.6274839287509237362, 1.000000000000000000),
 ( 1.000000000000000000, 0.6202923972654608153, 1.000000000000000000),
 ( 1.000000000000000000, 0.6166918370340956912, 1.000000000000000000),
 ( 1.000000000000000000, 0.6134846856060413023, 1.000000000000000000),
 ( 1.000000000000000000, 0.6127846890635409993, 1.000000000000000000),
 ( 1.000000000000000000, 0.6121417544835984215, 1.000000000000000000),
 ( 1.000000000000000000, 0.6121919490915220807, 1.000000000000000000),
 ( 1.000000000000000000, 0.6133751910668664431, 1.000000000000000000),
 ( 1.000000000000000000, 0.6155490712539813947, 1.000000000000000000),
 ( 1.000000000000000000, 0.6203878072413371303, 1.000000000000000000),
 ( 1.000000000000000000, 0.6222638419436984369, 1.000000000000000000),
 ( 1.000000000000000000, 0.6263429184244624359, 1.000000000000000000),
 ( 1.000000000000000000, 0.6285529934538920394, 1.000000000000000000),
 ( 1.000000000000000000, 0.6354958318040264675, 1.000000000000000000),
 ( 1.000000000000000000, 0.6405374649603885473, 1.000000000000000000),
 ( 1.000000000000000000, 0.6504850597404820967, 1.000000000000000000),
 ( 1.000000000000000000, 0.6552989879275363805, 1.000000000000000000),
 ( 1.000000000000000000, 0.6637694919636900615, 1.000000000000000000),
 ( 1.000000000000000000, 0.6674481112988286391, 1.000000000000000000),
 ( 1.000000000000000000, 0.6731606607313684876, 1.000000000000000000),
 ( 1.000000000000000000, 0.6751501093762943828, 1.000000000000000000),
 ( 1.000000000000000000, 0.6771367351906749654, 1.000000000000000000),
 ( 1.000000000000000000, 0.6771517807286357993, 1.000000000000000000),
 ( 1.000000000000000000, 0.6751929488707926197, 1.000000000000000000),
 ( 1.000000000000000000, 0.6731945361681611617, 1.000000000000000000),
 ( 1.000000000000000000, 0.6675581016157797754, 1.000000000000000000),
 ( 1.000000000000000000, 0.6639163920490709359, 1.000000000000000000),
 ( 1.000000000000000000, 0.6554729574460654851, 1.000000000000000000),
 ( 1.000000000000000000, 0.6506196326805566699, 1.000000000000000000),
 ( 1.000000000000000000, 0.6407412944952491918, 1.000000000000000000),
 ( 1.000000000000000000, 0.6357223030003761322, 1.000000000000000000),
 ( 1.000000000000000000, 0.6264724816114001227, 1.000000000000000000),
 ( 1.000000000000000000, 0.6222236727237925313, 1.000000000000000000),
 ( 1.000000000000000000, 0.6156853169344688181, 1.000000000000000000),
 ( 1.000000000000000000, 0.6134690707966352630, 1.000000000000000000),
 ( 1.000000000000000000, 0.6117931279243551401, 1.000000000000000000),
 ( 1.000000000000000000, 0.6123370218337945703, 1.000000000000000000),
 ( 1.000000000000000000, 0.6165118084860213843, 1.000000000000000000),
 ( 1.000000000000000000, 0.6200744837291712885, 1.000000000000000000),
 ( 1.000000000000000000, 0.6295916762275356460, 1.000000000000000000),
 ( 1.000000000000000000, 0.6355670384684388718, 1.000000000000000000),
 ( 1.000000000000000000, 0.6490362627856776090, 1.000000000000000000),
 ( 1.000000000000000000, 0.6564052266140359970, 1.000000000000000000),
 ( 1.000000000000000000, 0.6715002995394828700, 1.000000000000000000),
 ( 1.000000000000000000, 0.6792468330939857024, 1.000000000000000000),
 ( 1.000000000000000000, 0.6942451427572285949, 1.000000000000000000),
 ( 1.000000000000000000, 0.7013942707229733342, 1.000000000000000000),
 ( 1.000000000000000000, 0.7144494188210194219, 1.000000000000000000),
 ( 1.000000000000000000, 0.7203582787926783304, 1.000000000000000000),
 ( 1.000000000000000000, 0.7305132205854709682, 1.000000000000000000),
 ( 1.000000000000000000, 0.7347357360980601992, 1.000000000000000000),
 ( 1.000000000000000000, 0.7442195004274780867, 1.000000000000000000),
 ( 1.000000000000000000, 0.7464355310270405219, 1.000000000000000000),
 ( 1.000000000000000000, 0.7441515679388579496, 1.000000000000000000) ) ) 
 REPRESENTATION_ITEM ( '' )  SURFACE ( )  );
#12857=CARTESIAN_POINT ( 'NONE',  ( 25.51884215448320958, -4.718317418738882552, 0.4603789867971156413 ) ) ;
#12859=ORIENTED_EDGE ( 'NONE', *, *, #24489, .T. ) ;
#12860=CARTESIAN_POINT ( 'NONE',  ( -74.02829583808838265, 6.653335707795791087, 9.562392075533951541 ) ) ;
#12867=CARTESIAN_POINT ( 'NONE',  ( 28.18609449851297910, -3.183177124052247287, -4.605519748400973334 ) ) ;
#12868=CARTESIAN_POINT ( 'NONE',  ( 36.20103906056434795, -3.651302259472223533, -5.717550162322121210 ) ) ;
#12871=CARTESIAN_POINT ( 'NONE',  ( 19.96668899214778747, 6.747717534392478456, 3.285463770674537543 ) ) ;
#12873=CARTESIAN_POINT ( 'NONE',  ( 28.67087680535204797, -4.024283280459782119, 4.110896467804376009 ) ) ;
#12877=CARTESIAN_POINT ( 'NONE',  ( 22.48654264114678369, 0.6042035298600259008, -6.567991110914350728 ) ) ;
#12878=CARTESIAN_POINT ( 'NONE',  ( 30.85399364833475744, -3.769658692124774113, -4.573109180878241808 ) ) ;
#12880=ORIENTED_EDGE ( 'NONE', *, *, #6414, .T. ) ;
#12888=CARTESIAN_POINT ( 'NONE',  ( 87.06687503756165825, -0.7302844941506287935, -5.541598948305895611 ) ) ;
#12891=CARTESIAN_POINT ( 'NONE',  ( 24.67487267398843542, 2.663866308026491492, 3.912183617538783409 ) ) ;
#12892=CARTESIAN_POINT ( 'NONE',  ( 24.98423877875683985, 3.112984909006376810, -2.906875866008173936 ) ) ;
#12906=CARTESIAN_POINT ( 'NONE',  ( 23.14060042872244694, 4.027402677322106328, -3.115282196985579954 ) ) ;
#12907=ORIENTED_EDGE ( 'NONE', *, *, #31991, .F. ) ;
#12913=CARTESIAN_POINT ( 'NONE',  ( -80.68970021994135777, -6.620776169903922259, -2.209499440123503522 ) ) ;
#12915=FACE_OUTER_BOUND ( 'NONE', #7866, .T. ) ;
#12917=CARTESIAN_POINT ( 'NONE',  ( 86.53727031679849802, -0.6854317443871157378, -5.678301933988063155 ) ) ;
#12928=CARTESIAN_POINT ( 'NONE',  ( 33.13586453634747642, -3.753881462307791850, -5.125994689951091310 ) ) ;
#12932=CARTESIAN_POINT ( 'NONE',  ( 20.42279120405673609, 3.662518919516934535, 3.393868513101561124 ) ) ;
#12934=CARTESIAN_POINT ( 'NONE',  ( 86.21492201224262431, 1.517032185505227559, -5.007191195300914721 ) ) ;
#12937=CARTESIAN_POINT ( 'NONE',  ( -62.92837670882107659, -49.49506129533733656, 6.000000000000000000 ) ) ;
#12942=CARTESIAN_POINT ( 'NONE',  ( -80.29545004356899085, -6.646483628119856490, 3.526391997555196056 ) ) ;
#12950=CARTESIAN_POINT ( 'NONE',  ( 24.86342019672374448, 1.896585702110065164, 4.289962101907669023 ) ) ;
#12956=CARTESIAN_POINT ( 'NONE',  ( 86.24677872985614613, 1.481249208270744466, 4.702149241800761992 ) ) ;
#12960=CARTESIAN_POINT ( 'NONE',  ( 23.87989460547934684, 3.092228747732352456, -3.719817981150454145 ) ) ;
#12964=CARTESIAN_POINT ( 'NONE',  ( 21.85643539959776760, -12.33099359671888884, 6.023794913588264244 ) ) ;
#12965=CARTESIAN_POINT ( 'NONE',  ( 16.12938719712982660, 15.26369590459581360, 1.887449634883829663 ) ) ;
#12969=CARTESIAN_POINT ( 'NONE',  ( 86.60363381072151867, 0.9779648536402296699, 5.693185077828528229 ) ) ;
#12971=CARTESIAN_POINT ( 'NONE',  ( 14.71640407924273219, 12.89631605138042403, 2.500000000000011546 ) ) ;
#12972=CARTESIAN_POINT ( 'NONE',  ( 17.14784120125169409, -3.222914996324496517, 2.862138963676726711 ) ) ;
#12973=CARTESIAN_POINT ( 'NONE',  ( 34.33288252766027426, -1.486090089270978298, -5.564874680979682964 ) ) ;
#12977=CARTESIAN_POINT ( 'NONE',  ( 30.67406393699503298, -3.593393542108534344, -4.777508688867102116 ) ) ;
#12984=CARTESIAN_POINT ( 'NONE',  ( 28.44546091714163438, -4.072879259825384679, 4.061366448452340627 ) ) ;
#12987=CARTESIAN_POINT ( 'NONE',  ( 36.13125622736320253, -1.533072422867240325, 5.645132520243028473 ) ) ;
#12990=ORIENTED_EDGE ( 'NONE', *, *, #16842, .T. ) ;
#12991=CARTESIAN_POINT ( 'NONE',  ( -77.46169046775075628, 11.07004784189294000, -7.581925507970804112 ) ) ;
#13006=CARTESIAN_POINT ( 'NONE',  ( 14.89600225145155576, 12.34220076978314751, -2.524950096939041266 ) ) ;
#13010=VECTOR ( 'NONE', #24122, 1000.000000000000000 ) ;
#13017=CARTESIAN_POINT ( 'NONE',  ( 26.62075075102985267, 2.678422205045695392, 2.704210781993271695 ) ) ;
#13024=CARTESIAN_POINT ( 'NONE',  ( 27.58412137558927313, 1.448149839084869051, -4.473612028233096005 ) ) ;
#13030=CARTESIAN_POINT ( 'NONE',  ( 21.88434783170197662, -13.24225184460187776, -2.500000000000000000 ) ) ;
#13031=AXIS2_PLACEMENT_3D ( 'NONE', #28983, #40710, #34981 ) ;
#13035=VERTEX_POINT ( 'NONE', #28204 ) ;
#13041=CARTESIAN_POINT ( 'NONE',  ( 30.19003827612802482, -2.952522945788203845, 4.918283640461378781 ) ) ;
#13042=CARTESIAN_POINT ( 'NONE',  ( 22.22390872265649620, 3.654499484256482855, 4.238281575154772440 ) ) ;
#13048=CLOSED_SHELL ( 'NONE', ( #10965, #38238, #7578, #10810, #37190, #7160, #5316, #23753, #37043, #1937, #40677, #75, #34038, #12576, #13260, #17682, #16627, #10858, #6368, #27931, #36312, #11331, #22300, #31120, #5295, #23411, #34758, #25075, #17919, #13683, #1587, #33726, #36806, #546, #37827, #4250, #34103, #35707, #18586, #3292, #37761, #36628, #18216, #14921, #28692, #38063, #36501, #18351, #35730, #29753, #26600, #8924, #14969, #10730, #1120, #24682, #684, #16623, #1145, #12277, #28889, #8381, #31584, #36765, #19768, #6722, #10685, #6897, #13367, #32657, #2106, #20398, #7024, #1878, #36803, #37272, #30659, #15380, #3793, #15883, #4645, #16051, #23170, #4114, #32253, #21000, #19845, #5169, #21205, #4929, #15421, #2299, #29252, #14450, #28176, #25310, #3343, #1770, #16825, #32093, #5399, #6889, #31809, #21439, #39762, #22350, #7854, #35586, #2822, #34559, #6005, #32246, #30412, #33107 ) ) ;
#13053=CARTESIAN_POINT ( 'NONE',  ( 23.62521421733200810, 0.5032721505374657678, 5.478091647691247346 ) ) ;
#13059=CARTESIAN_POINT ( 'NONE',  ( -17.69482985384422236, -39.37473357531881391, -6.000000000000000000 ) ) ;
#13062=EDGE_LOOP ( 'NONE', ( #4154, #31398, #14602, #30656, #35550 ) ) ;
#13063=CARTESIAN_POINT ( 'NONE',  ( 22.80949115205394406, -6.484386712482024251, -3.653976874014524867 ) ) ;
#13066=CARTESIAN_POINT ( 'NONE',  ( -73.23935992792370087, 4.942735534762467964, 9.788940037685113893 ) ) ;
#13067=FACE_OUTER_BOUND ( 'NONE', #2748, .T. ) ;
#13073=CARTESIAN_POINT ( 'NONE',  ( 32.90368182600108327, -3.810879906198540112, -4.978789352745470964 ) ) ;
#13074=CARTESIAN_POINT ( 'NONE',  ( 37.10982994964820847, -2.403900326362613971, -5.951681757502289116 ) ) ;
#13076=CARTESIAN_POINT ( 'NONE',  ( 17.01637594748899218, 9.184973690624572029, 2.862215027849857929 ) ) ;
#13079=DIRECTION ( 'NONE',  ( 1.000000000000000000, -0.000000000000000000, 0.000000000000000000 ) ) ;
#13081=CARTESIAN_POINT ( 'NONE',  ( 25.66313521821469479, 1.726747700288609799, -4.270219735217844814 ) ) ;
#13082=CARTESIAN_POINT ( 'NONE',  ( 35.68902945888083167, -1.289468566711789554, -5.530809620460434672 ) ) ;
#13083=VECTOR ( 'NONE', #33164, 1000.000000000000000 ) ;
#13089=CARTESIAN_POINT ( 'NONE',  ( 85.94684271633954609, 0.9790069142357779031, 5.868308835085408681 ) ) ;
#13092=CARTESIAN_POINT ( 'NONE',  ( -76.84400769949562005, 9.411604022321832019, -9.587408972141622243 ) ) ;
#13094=CARTESIAN_POINT ( 'NONE',  ( -4.444218661349752963, -35.94265729135299381, 2.500000000000000000 ) ) ;
#13106=DIRECTION ( 'NONE',  ( 0.000000000000000000, -0.000000000000000000, -1.000000000000000000 ) ) ;
#13107=ORIENTED_EDGE ( 'NONE', *, *, #4123, .T. ) ;
#13114=CARTESIAN_POINT ( 'NONE',  ( 21.85643539959778892, 11.01376456104441104, -6.033145431426138572 ) ) ;
#13115=CARTESIAN_POINT ( 'NONE',  ( 21.72163592607151728, 6.243142354532070115, -3.223666675097538459 ) ) ;
#13121=CARTESIAN_POINT ( 'NONE',  ( -79.87442750853132623, -5.634526803139693563, -4.486596260177802442 ) ) ;
#13123=CARTESIAN_POINT ( 'NONE',  ( -80.92837670882107659, 2.429809908903242555, -12.50000000000000000 ) ) ;
#13125=CARTESIAN_POINT ( 'NONE',  ( 84.96089493372460311, 1.928984934743871449, -4.835719925821683418 ) ) ;
#13126=CARTESIAN_POINT ( 'NONE',  ( 25.01091293497539780, 3.329590547006094248, -1.936828119410943350 ) ) ;
#13131=CARTESIAN_POINT ( 'NONE',  ( -71.92837670882107659, -20.78299143688747819, 9.949874371066202983 ) ) ;
#13134=EDGE_CURVE ( 'NONE', #36097, #26946, #32146, .T. ) ;
#13136=CARTESIAN_POINT ( 'NONE',  ( 34.93030302952856658, -1.707825049874648560, 5.658116598965852617 ) ) ;
#13139=CARTESIAN_POINT ( 'NONE',  ( 88.07575545775937087, -0.5731442609823791390, 3.387043347726935050 ) ) ;
#13144=CARTESIAN_POINT ( 'NONE',  ( -70.26248529839136836, -48.46472069417173145, 9.978220256720669923 ) ) ;
#13149=CARTESIAN_POINT ( 'NONE',  ( -73.93807322288319028, -3.714211979007700393, 9.537397809311197960 ) ) ;
#13150=VERTEX_POINT ( 'NONE', #19362 ) ;
#13153=CARTESIAN_POINT ( 'NONE',  ( 23.39816613655191802, 1.771640793782062406, 4.881439243339824152 ) ) ;
#13161=CARTESIAN_POINT ( 'NONE',  ( 86.43327874156520352, 1.271763543294590848, 4.874929521669852051 ) ) ;
#13166=CARTESIAN_POINT ( 'NONE',  ( 21.85074289711433337, 4.166209864296642529, -4.242968198356735776 ) ) ;
#13170=CARTESIAN_POINT ( 'NONE',  ( 21.85643539959774273, -6.858222381794880640, 10.60035608423801357 ) ) ;
#13171=CARTESIAN_POINT ( 'NONE',  ( 21.85643539959777826, 3.765123657700753412, -3.918568846603332378 ) ) ;
#13174=CARTESIAN_POINT ( 'NONE',  ( 85.38594790374143884, 2.393190016811436394, 3.957880923259903927 ) ) ;
#13177=CARTESIAN_POINT ( 'NONE',  ( 16.21041041637272428, -3.304833269244274341, 2.736424614369139530 ) ) ;
#13179=CARTESIAN_POINT ( 'NONE',  ( 34.92983894306404125, -1.709246109001034020, -5.658044167049093964 ) ) ;
#13185=CARTESIAN_POINT ( 'NONE',  ( 28.20895372393743017, -3.294009627498124093, 4.609087483380881700 ) ) ;
#13188=CARTESIAN_POINT ( 'NONE',  ( 32.06717985418615768, 0.2495969218020720470, 4.732404502101774213 ) ) ;
#13195=FACE_BOUND ( 'NONE', #19852, .T. ) ;
#13196=ORIENTED_EDGE ( 'NONE', *, *, #6084, .F. ) ;
#13207=CARTESIAN_POINT ( 'NONE',  ( 15.57425752064463076, 11.08950951739397262, -2.625789524671749753 ) ) ;
#13215=CARTESIAN_POINT ( 'NONE',  ( 22.81629046404031413, 3.691080719936705279, -3.767431959620346937 ) ) ;
#13219=CARTESIAN_POINT ( 'NONE',  ( 14.51114108199450925, 10.82491523625665053, 2.499999999996797229 ) ) ;
#13220=CARTESIAN_POINT ( 'NONE',  ( 28.43092716748534343, -1.248584762127236569, 6.041969456467763955 ) ) ;
#13222=CARTESIAN_POINT ( 'NONE',  ( -70.79780587197991792, -21.78299143688773043, 10.00000000000003020 ) ) ;
#13225=DIRECTION ( 'NONE',  ( 1.000000000000000000, 0.000000000000000000, 0.000000000000000000 ) ) ;
#13227=CARTESIAN_POINT ( 'NONE',  ( 36.66469078098081980, -3.237339655608454603, -5.925250000093051028 ) ) ;
#13231=CARTESIAN_POINT ( 'NONE',  ( -81.32912492467333720, 10.50070982703512712, 3.457416654607596840 ) ) ;
#13232=CARTESIAN_POINT ( 'NONE',  ( 22.07803051241986836, -11.23212333282388009, -2.500000000000000444 ) ) ;
#13234=CARTESIAN_POINT ( 'NONE',  ( 31.76537530306199741, -2.962049296186602731, 5.164153083184395143 ) ) ;
#13240=CARTESIAN_POINT ( 'NONE',  ( -62.92837670882106238, -23.80776546975053520, 6.000000000000000000 ) ) ;
#13241=CARTESIAN_POINT ( 'NONE',  ( 22.20338448559262901, 4.015215451811328329, 3.998823550933331195 ) ) ;
#13244=LINE ( 'NONE', #1122, #12002 ) ;
#13247=CARTESIAN_POINT ( 'NONE',  ( 21.29078198983360792, -3.051855081372369938, 3.444149166357055591 ) ) ;
#13253=CARTESIAN_POINT ( 'NONE',  ( 23.60046373739841030, 0.4362303430042576147, 5.514821429153919041 ) ) ;
#13259=LINE ( 'NONE', #13868, #40495 ) ;
#13260=ADVANCED_FACE ( 'NONE', ( #5124 ), #24256, .F. ) ;
#13263=CARTESIAN_POINT ( 'NONE',  ( 25.28494853283190125, -3.333630280469910723, 5.108382079771137008 ) ) ;
#13266=CARTESIAN_POINT ( 'NONE',  ( -77.73005492033482255, -4.997448663934537905, 8.952513429815514456 ) ) ;
#13268=CARTESIAN_POINT ( 'NONE',  ( 21.66003001261448802, 6.756596355199507187, 2.827218952364252580 ) ) ;
#13269=CARTESIAN_POINT ( 'NONE',  ( 35.36801745506461003, -3.791884530138194265, -5.511195673735667988 ) ) ;
#13271=CARTESIAN_POINT ( 'NONE',  ( 21.38350792168483139, 5.477734254629577748, 3.543811591909045156 ) ) ;
#13276=CARTESIAN_POINT ( 'NONE',  ( 26.33495388482178257, 1.786803017097982504, -4.277245124679304844 ) ) ;
#13278=CARTESIAN_POINT ( 'NONE',  ( 33.68488252487933465, -0.3869890349111386740, -5.069973516189887341 ) ) ;
#13283=CARTESIAN_POINT ( 'NONE',  ( 86.57035376367728929, -0.007661497531101129840, -5.962853773335548446 ) ) ;
#13284=VERTEX_POINT ( 'NONE', #1640 ) ;
#13285=CARTESIAN_POINT ( 'NONE',  ( -73.12373367897625087, 4.565503759671822870, -10.93214365780120545 ) ) ;
#13288=DIRECTION ( 'NONE',  ( -5.570824187210003553E-14, 1.000000000000000000, -6.938893903907129770E-15 ) ) ;
#13289=ORIENTED_EDGE ( 'NONE', *, *, #6520, .T. ) ;
#13296=ORIENTED_EDGE ( 'NONE', *, *, #20671, .T. ) ;
#13302=CARTESIAN_POINT ( 'NONE',  ( 21.85643539959776049, -14.86125632165375343, -4.251346793879176467 ) ) ;
#13303=CARTESIAN_POINT ( 'NONE',  ( 22.00415366418653562, 5.540035186195420458, -3.131174203737818296 ) ) ;
#13309=CARTESIAN_POINT ( 'NONE',  ( -74.10404772851687483, -1.915033150869918099, -10.75253851325693688 ) ) ;
#13313=CARTESIAN_POINT ( 'NONE',  ( 87.52985346608603834, -1.683278932971326691, -4.201117388013917875 ) ) ;
#13316=CARTESIAN_POINT ( 'NONE',  ( 21.55641518153495184, 7.313212361982168730, -1.964796485855104358 ) ) ;
#13322=CARTESIAN_POINT ( 'NONE',  ( 36.97985918926679005, -2.956901537102269106, 5.977999406396011572 ) ) ;
#13326=CARTESIAN_POINT ( 'NONE',  ( 87.26180097699096905, 0.3411280444268214862, 4.951700522085849876 ) ) ;
#13331=EDGE_CURVE ( 'NONE', #36906, #5482, #10202, .T. ) ;
#13334=ORIENTED_EDGE ( 'NONE', *, *, #9670, .T. ) ;
#13335=EDGE_CURVE ( 'NONE', #31580, #28300, #11480, .T. ) ;
#13344=CARTESIAN_POINT ( 'NONE',  ( 25.13028398501089455, 2.418633085955766759, 4.024527564920112432 ) ) ;
#13349=EDGE_CURVE ( 'NONE', #25264, #15683, #23348, .T. ) ;
#13351=CARTESIAN_POINT ( 'NONE',  ( 85.36365109362724013, 2.473220085049208983, 2.424004168925880442 ) ) ;
#13355=CARTESIAN_POINT ( 'NONE',  ( 24.36792415750019458, 2.936288794802523139, -3.728798694104302758 ) ) ;
#13359=CARTESIAN_POINT ( 'NONE',  ( 21.85643539959774273, 10.54266624894746229, 1.842303177338921572 ) ) ;
#13360=CARTESIAN_POINT ( 'NONE',  ( 21.87484035784453695, 3.535422555123523658, 3.391095861108603504 ) ) ;
#13363=CARTESIAN_POINT ( 'NONE',  ( 87.94592890065770519, -0.6044765299818539717, 4.822713664802365408 ) ) ;
#13367=ADVANCED_FACE ( 'NONE', ( #30443 ), #2253, .F. ) ;
#13368=CARTESIAN_POINT ( 'NONE',  ( 15.06368528933364281, -4.031268556551167670, 2.557450424642690567 ) ) ;
#13369=CARTESIAN_POINT ( 'NONE',  ( 35.92872908462157966, -2.111607858196849818, 5.813945131888477391 ) ) ;
#13371=CARTESIAN_POINT ( 'NONE',  ( 34.13611374073711602, -3.134507220645912806, -5.534164152908742196 ) ) ;
#13373=CARTESIAN_POINT ( 'NONE',  ( 84.50896143996750709, 2.514019815156651294, -3.493124578469008146 ) ) ;
#13378=CARTESIAN_POINT ( 'NONE',  ( 32.89828394892415275, -3.753738769583905288, 5.047802179214622598 ) ) ;
#13380=ORIENTED_EDGE ( 'NONE', *, *, #16507, .T. ) ;
#13381=CARTESIAN_POINT ( 'NONE',  ( 37.18642854612528481, -2.963312751682652735, 6.000018072115591572 ) ) ;
#13385=CARTESIAN_POINT ( 'NONE',  ( 86.66947201173555015, -0.8835633689198520990, 5.500948792305413448 ) ) ;
#13391=CARTESIAN_POINT ( 'NONE',  ( 14.77315594796471743, 13.19392823276620419, 2.499999999999996891 ) ) ;
#13392=ORIENTED_EDGE ( 'NONE', *, *, #40273, .F. ) ;
#13397=CARTESIAN_POINT ( 'NONE',  ( 24.27615491347996723, 3.119136480584640658, 3.486480195292287032 ) ) ;
#13402=EDGE_CURVE ( 'NONE', #15998, #5350, #16120, .T. ) ;
#13410=CARTESIAN_POINT ( 'NONE',  ( 25.33160239074249986, 2.112310346557956908, -4.160007218831053954 ) ) ;
#13413=CARTESIAN_POINT ( 'NONE',  ( 27.88065694771982450, 2.580388505813413502, -1.055963728923108524 ) ) ;
#13415=DIRECTION ( 'NONE',  ( -0.000000000000000000, -0.000000000000000000, -1.000000000000000000 ) ) ;
#13420=CARTESIAN_POINT ( 'NONE',  ( 36.98988159880491366, -2.542881062934562841, -5.977438618132547177 ) ) ;
#13427=CARTESIAN_POINT ( 'NONE',  ( 21.88286327911765028, -13.27756337371481798, -2.499999999999999556 ) ) ;
#13428=CARTESIAN_POINT ( 'NONE',  ( 21.87963034546448071, -13.35931693332254788, 2.500000000000000444 ) ) ;
#13429=EDGE_CURVE ( 'NONE', #30233, #31898, #5000, .T. ) ;
#13431=CARTESIAN_POINT ( 'NONE',  ( 33.75536587385149545, -0.8752969169947810713, 5.454565398524055198 ) ) ;
#13441=CARTESIAN_POINT ( 'NONE',  ( 24.35459986608915628, 2.895258409799770227, 3.776052705250971364 ) ) ;
#13446=CARTESIAN_POINT ( 'NONE',  ( 21.82997413388621410, 5.965416049814977306, 3.134756262805778793 ) ) ;
#13450=DIRECTION ( 'NONE',  ( 0.000000000000000000, 0.000000000000000000, -1.000000000000000000 ) ) ;
#13454=CARTESIAN_POINT ( 'NONE',  ( 26.05429450752729892, 0.7955742409443752328, 4.421904258172623337 ) ) ;
#13462=CARTESIAN_POINT ( 'NONE',  ( 25.43482567069144906, -3.911874351919522041, 4.043259094187231284 ) ) ;
#13465=CARTESIAN_POINT ( 'NONE',  ( -79.86026552043743720, -5.632672876117126748, 4.514648094728398675 ) ) ;
#13466=CARTESIAN_POINT ( 'NONE',  ( 23.58040427942380290, 0.3886573651980784194, -5.537642973953215808 ) ) ;
#13472=CARTESIAN_POINT ( 'NONE',  ( 36.13290868086723862, -1.530173128070416055, -5.643002085621601438 ) ) ;
#13475=DIRECTION ( 'NONE',  ( 0.000000000000000000, -0.000000000000000000, -1.000000000000000000 ) ) ;
#13478=CARTESIAN_POINT ( 'NONE',  ( 30.43224445366828235, -3.649418619126846508, 4.685639825479781528 ) ) ;
#13482=CARTESIAN_POINT ( 'NONE',  ( 21.94609799796423744, 0.7904948903713955310, -7.266583015939693801 ) ) ;
#13483=CARTESIAN_POINT ( 'NONE',  ( 34.16050310316816052, -0.5835275994841344627, -5.173420616574753161 ) ) ;
#13484=CARTESIAN_POINT ( 'NONE',  ( 20.40287464304303100, 10.75613383955523616, -2.500000000000000000 ) ) ;
#13489=CARTESIAN_POINT ( 'NONE',  ( 84.34456690318765482, 2.887654542466673746, -2.101772343363317752 ) ) ;
#13493=CARTESIAN_POINT ( 'NONE',  ( -81.51664041560071894, 10.48936286263200834, -2.744537766835254189 ) ) ;
#13504=CARTESIAN_POINT ( 'NONE',  ( 37.13477802123105675, -2.471947244483942097, 5.963681894023967089 ) ) ;
#13512=CARTESIAN_POINT ( 'NONE',  ( 21.85643539959774273, 11.61750052538138256, -3.706567411524428479 ) ) ;
#13513=DIRECTION ( 'NONE',  ( 0.000000000000000000, 0.000000000000000000, -1.000000000000000000 ) ) ;
#13514=CARTESIAN_POINT ( 'NONE',  ( 24.40656851573213260, 3.164061221018514836, -3.268877201782123709 ) ) ;
#13517=ORIENTED_EDGE ( 'NONE', *, *, #26203, .T. ) ;
#13520=CARTESIAN_POINT ( 'NONE',  ( -71.87663712502020985, 3.986363140443492270, -9.955339895040744125 ) ) ;
#13521=CARTESIAN_POINT ( 'NONE',  ( 1.700390093233090871, -29.56993018339339940, 27.90461065042423527 ) ) ;
#13524=CARTESIAN_POINT ( 'NONE',  ( 84.33668400229728945, 2.728897857615574019, 2.746074863882507877 ) ) ;
#13526=FACE_OUTER_BOUND ( 'NONE', #19578, .T. ) ;
#13535=CARTESIAN_POINT ( 'NONE',  ( 33.62865206644069360, -1.228866384903354092, 5.454962485628514379 ) ) ;
#13538=CARTESIAN_POINT ( 'NONE',  ( 86.67773139875836819, 0.9971827163122055637, 5.329716871657868005 ) ) ;
#13546=VERTEX_POINT ( 'NONE', #28373 ) ;
#13547=CARTESIAN_POINT ( 'NONE',  ( -72.55849701049024247, 6.338670283186906396, 9.867990834847722326 ) ) ;
#13551=CARTESIAN_POINT ( 'NONE',  ( 22.01028799361013455, 1.448149096448989148, 6.405474035339984162 ) ) ;
#13553=VERTEX_POINT ( 'NONE', #11888 ) ;
#13562=EDGE_CURVE ( 'NONE', #12553, #9974, #21386, .T. ) ;
#13563=CARTESIAN_POINT ( 'NONE',  ( 21.85277127755108850, 4.059747631923805500, -4.311690313514618289 ) ) ;
#13565=FACE_OUTER_BOUND ( 'NONE', #31051, .T. ) ;
#13567=VERTEX_POINT ( 'NONE', #40305 ) ;
#13568=CARTESIAN_POINT ( 'NONE',  ( 21.85643539959774984, 7.798985686765059100, -6.733359799098007414 ) ) ;
#13569=CARTESIAN_POINT ( 'NONE',  ( 17.10505430642727021, 14.50076029600939620, -3.172244300427717878 ) ) ;
#13572=CARTESIAN_POINT ( 'NONE',  ( 87.33013056844055200, 0.1115698105147486796, -5.569409363020906056 ) ) ;
#13573=CARTESIAN_POINT ( 'NONE',  ( 26.00676459590870948, -2.423824083598640655, 4.803740791041811953 ) ) ;
#13574=ORIENTED_EDGE ( 'NONE', *, *, #9324, .F. ) ;
#13575=CARTESIAN_POINT ( 'NONE',  ( 26.28262498061524255, -2.815787221564533649, 4.308437294549054997 ) ) ;
#13578=CARTESIAN_POINT ( 'NONE',  ( 26.27644361979791299, -2.815469118397957438, -4.307472543696508005 ) ) ;
#13579=CARTESIAN_POINT ( 'NONE',  ( 36.14145924306839675, -3.142491748452399758, -5.847146818012371128 ) ) ;
#13583=ORIENTED_EDGE ( 'NONE', *, *, #23579, .T. ) ;
#13586=CARTESIAN_POINT ( 'NONE',  ( 32.88573892376593477, -3.567000722825174996, 5.242007489099518303 ) ) ;
#13590=CARTESIAN_POINT ( 'NONE',  ( 37.21201414827569209, -2.743731264475244735, 6.000895904599971686 ) ) ;
#13595=CARTESIAN_POINT ( 'NONE',  ( 87.74957675019172143, -2.299229798971626160, -2.336605637469935548 ) ) ;
#13603=CARTESIAN_POINT ( 'NONE',  ( 23.14817712711864672, 3.972822056005928193, 3.193607562712095227 ) ) ;
#13616=CARTESIAN_POINT ( 'NONE',  ( 25.78025694704896509, 1.897212611309158747, -4.230030613094124092 ) ) ;
#13619=CARTESIAN_POINT ( 'NONE',  ( 86.66388813748453401, 1.012732124415782531, -5.000054679117940104 ) ) ;
#13621=CARTESIAN_POINT ( 'NONE',  ( 28.77170544830297416, -1.679059579700503901, 5.945470488877720783 ) ) ;
#13629=CARTESIAN_POINT ( 'NONE',  ( -81.73797001107014637, -5.609980832826766850, -1.463193866445242186 ) ) ;
#13632=CARTESIAN_POINT ( 'NONE',  ( 37.02894987274358130, -3.025198956107289394, -5.984733352030005449 ) ) ;
#13637=CARTESIAN_POINT ( 'NONE',  ( 21.89416422391149553, -13.03218691091165482, -2.499999999999999556 ) ) ;
#13640=CARTESIAN_POINT ( 'NONE',  ( 30.66838910461938283, 0.2949634357040269994, 4.962894452049861904 ) ) ;
#13647=DIRECTION ( 'NONE',  ( -0.9616058754224561245, 0.2744342186262705430, 0.000000000000000000 ) ) ;
#13648=CARTESIAN_POINT ( 'NONE',  ( 30.88504653261737687, -3.473826543452005922, 4.907706032697572773 ) ) ;
#13651=CARTESIAN_POINT ( 'NONE',  ( 21.71182896267971074, 6.328908860361642574, -3.192117583127509928 ) ) ;
#13657=CARTESIAN_POINT ( 'NONE',  ( 22.38195073352680353, 4.938598426050218038, 3.049351103695999932 ) ) ;
#13658=DIRECTION ( 'NONE',  ( -1.000000000000000000, 0.000000000000000000, 0.000000000000000000 ) ) ;
#13663=CARTESIAN_POINT ( 'NONE',  ( 23.06111833571992165, 0.3526964807778580901, 5.951137662820944918 ) ) ;
#13674=CARTESIAN_POINT ( 'NONE',  ( 25.45397947482645762, -4.047761836529544688, -3.708248611797466232 ) ) ;
#13677=CARTESIAN_POINT ( 'NONE',  ( -74.01735817102475323, -1.775513542402386014, 9.566008380307465586 ) ) ;
#13678=CARTESIAN_POINT ( 'NONE',  ( 26.06763238852761333, 0.7305626207722594190, -4.422385087239707246 ) ) ;
#13683=ADVANCED_FACE ( 'NONE', ( #29187 ), #16218, .F. ) ;
#13684=CARTESIAN_POINT ( 'NONE',  ( 34.63719001687865529, -0.7818850938027223085, -5.275113761647806321 ) ) ;
#13685=CARTESIAN_POINT ( 'NONE',  ( 30.77571102275213732, -3.326538504857021294, -4.963279402896310089 ) ) ;
#13692=CARTESIAN_POINT ( 'NONE',  ( 30.19238557334687911, -2.952639005720375742, -4.918649992961978690 ) ) ;
#13698=CARTESIAN_POINT ( 'NONE',  ( 85.61743365444765175, 1.218782235343771836, 5.694237175320765232 ) ) ;
#13705=B_SPLINE_CURVE_WITH_KNOTS ( 'NONE', 3,
 ( #39858, #21131, #37375, #36972, #9171, #37172, #40254, #21336, #15347, #18632, #21743, #34325, #33908, #5685, #18228, #6096, #12040, #28113, #30817, #31218, #27700, #2623, #38381 ),
 .UNSPECIFIED., .F., .F.,
 ( 4, 1, 1, 1, 1, 1, 1, 2, 2, 1, 1, 1, 1, 1, 2, 2, 4 ),
 ( 0.000000000000000000, 0.1250000000000023870, 0.1875000000000044964, 0.2187500000000058842, 0.2343750000000065503, 0.2421875000000077993, 0.2460937500000071054, 0.2480468750000068001, 0.2500000000000064393, 0.3750000000000008882, 0.4374999999999990008, 0.4687499999999974465, 0.4843749999999963918, 0.4921874999999948375, 0.4960937499999947820, 0.4999999999999946709, 1.000000000000000000 ),
 .UNSPECIFIED. ) ;
#13709=EDGE_CURVE ( 'NONE', #13567, #23822, #27981, .T. ) ;
#13712=CARTESIAN_POINT ( 'NONE',  ( 13.68084587807537211, 8.951768997783636550, -3.481680170128817586 ) ) ;
#13720=CARTESIAN_POINT ( 'NONE',  ( 21.85643539959780313, 0.8081825263151607430, -15.79083533483346535 ) ) ;
#13730=CARTESIAN_POINT ( 'NONE',  ( -75.21192073048329974, -3.284165063629141290, -10.40382875421505204 ) ) ;
#13739=DIRECTION ( 'NONE',  ( 1.000000000000000000, 0.000000000000000000, 0.000000000000000000 ) ) ;
#13744=CARTESIAN_POINT ( 'NONE',  ( 27.40774226395753388, 0.9655407106828844954, 4.484039057678827156 ) ) ;
#13747=CARTESIAN_POINT ( 'NONE',  ( 84.92887162652053235, 2.911150016110632510, -2.020846097872043501 ) ) ;
#13754=CARTESIAN_POINT ( 'NONE',  ( 23.36034022128349363, -7.521608558640657805, -2.500000000000000444 ) ) ;
#13761=CARTESIAN_POINT ( 'NONE',  ( 25.02156159189623352, 1.129856609166535186, 4.599960578933319333 ) ) ;
#13768=CARTESIAN_POINT ( 'NONE',  ( 21.99199484643884617, 4.642299483723236087, -3.779662632850636861 ) ) ;
#13774=CARTESIAN_POINT ( 'NONE',  ( 23.93232801731964443, 3.995115622954060530, -2.300403959411237320 ) ) ;
#13775=CARTESIAN_POINT ( 'NONE',  ( 21.80570325383041208, 6.356989464231460829, -3.898355529981889500 ) ) ;
#13779=CARTESIAN_POINT ( 'NONE',  ( 84.97295377430323526, 2.662001904288300302, 3.416982328422734305 ) ) ;
#13783=CARTESIAN_POINT ( 'NONE',  ( 14.72357206727486556, -4.485203473217731052, 2.504367530671055331 ) ) ;
#13787=CARTESIAN_POINT ( 'NONE',  ( 34.92879589194200918, -1.712044492387412742, -5.657881373695215821 ) ) ;
#13789=CARTESIAN_POINT ( 'NONE',  ( 84.67345804563912282, 2.302372249231917412, 4.084305866287619047 ) ) ;
#13796=CARTESIAN_POINT ( 'NONE',  ( 35.73027522876729023, -1.304475999450107615, 5.538144598496089088 ) ) ;
#13797=CARTESIAN_POINT ( 'NONE',  ( 16.44412387426018185, -3.224078058481200770, 2.772901251853813420 ) ) ;
#13799=CARTESIAN_POINT ( 'NONE',  ( 14.77315594796849574, 13.19392823276453441, -2.500000000000005773 ) ) ;
#13800=CARTESIAN_POINT ( 'NONE',  ( 86.28440875934980170, -0.2633909481622456195, 5.902347234764444117 ) ) ;
#13802=EDGE_LOOP ( 'NONE', ( #29447, #20921, #28650, #13875, #7157, #40338 ) ) ;
#13809=CARTESIAN_POINT ( 'NONE',  ( 21.93898495623947298, 5.250604734135974283, 3.452261465700366738 ) ) ;
#13815=DIRECTION ( 'NONE',  ( -1.000000000000000000, 0.000000000000000000, 0.000000000000000000 ) ) ;
#13817=CARTESIAN_POINT ( 'NONE',  ( 24.73513624196588268, 2.629268958504959564, -3.929116450179705122 ) ) ;
#13827=CARTESIAN_POINT ( 'NONE',  ( 27.87470673840761037, 2.608020033772324275, -0.5247038454205935620 ) ) ;
#13829=CARTESIAN_POINT ( 'NONE',  ( -70.42535609528330554, -21.65703093012598401, 9.988066921647984486 ) ) ;
#13834=CARTESIAN_POINT ( 'NONE',  ( 37.06194287117967434, -2.795410267932249671, -5.990810550159801906 ) ) ;
#13842=CARTESIAN_POINT ( 'NONE',  ( 35.80552223569445403, -3.523224689456814662, 5.749495820074442598 ) ) ;
#13846=ORIENTED_EDGE ( 'NONE', *, *, #9414, .F. ) ;
#13849=CARTESIAN_POINT ( 'NONE',  ( 84.98208903537448577, 1.898203206837230983, -4.865140515105523811 ) ) ;
#13857=CARTESIAN_POINT ( 'NONE',  ( 21.83475994719001534, 5.936717745254647127, 3.147461123595437726 ) ) ;
#13864=CARTESIAN_POINT ( 'NONE',  ( 23.06597301177588477, 0.3557582928994350580, 5.946024084739200077 ) ) ;
#13868=CARTESIAN_POINT ( 'NONE',  ( -70.92837670882107659, -23.80776546975053520, 10.00000000000000888 ) ) ;
#13872=DIRECTION ( 'NONE',  ( -0.000000000000000000, -1.000000000000000000, -0.000000000000000000 ) ) ;
#13873=CARTESIAN_POINT ( 'NONE',  ( 29.92651255597534288, -3.613225851372795727, -4.302012675596341928 ) ) ;
#13875=ORIENTED_EDGE ( 'NONE', *, *, #9334, .F. ) ;
#13876=CARTESIAN_POINT ( 'NONE',  ( -75.57379153473316080, -3.643616896758648860, 8.892515182195944945 ) ) ;
#13877=CARTESIAN_POINT ( 'NONE',  ( 25.39897559319004827, 0.6933974945119176780, -4.599801555308138390 ) ) ;
#13881=CARTESIAN_POINT ( 'NONE',  ( 37.10418691205928354, -3.126297194733565821, -5.976226130023548855 ) ) ;
#13885=CARTESIAN_POINT ( 'NONE',  ( -72.42837670882107659, -47.11702805680359063, 5.809475019311127753 ) ) ;
#13897=CARTESIAN_POINT ( 'NONE',  ( 84.20866968570335587, 3.050835305001676101, 0.3231758755354003920 ) ) ;
#13898=CARTESIAN_POINT ( 'NONE',  ( 26.60317387207919637, 1.634061885071666387, 4.331281458463850598 ) ) ;
#13909=CARTESIAN_POINT ( 'NONE',  ( 24.21182342437587565, 2.662150305148283547, 3.985238629172898950 ) ) ;
#13910=CARTESIAN_POINT ( 'NONE',  ( 17.34275990732152195, 9.186172967928778021, -2.849824708884751256 ) ) ;
#13912=DIRECTION ( 'NONE',  ( 0.000000000000000000, 0.000000000000000000, -1.000000000000000000 ) ) ;
#13913=CARTESIAN_POINT ( 'NONE',  ( 22.87846855920513178, 4.336014621590010165, -3.060014917398448553 ) ) ;
#13914=ORIENTED_EDGE ( 'NONE', *, *, #39934, .F. ) ;
#13916=LINE ( 'NONE', #36157, #26763 ) ;
#13918=CARTESIAN_POINT ( 'NONE',  ( -71.75727376073825781, 2.199410611364987389, -9.965632999380227730 ) ) ;
#13932=CARTESIAN_POINT ( 'NONE',  ( 27.40694485339065523, 0.9632844686313415394, 4.483914602474418309 ) ) ;
#13934=VERTEX_POINT ( 'NONE', #28529 ) ;
#13936=CARTESIAN_POINT ( 'NONE',  ( 85.03556247682649882, 2.841744791465048880, -1.219259102000758821 ) ) ;
#13948=EDGE_CURVE ( 'NONE', #37746, #24175, #11747, .T. ) ;
#13950=APPLICATION_CONTEXT ( 'automotive_design' ) ;
#13954=CARTESIAN_POINT ( 'NONE',  ( 22.13516576602885166, 0.4647494749783319112, 7.195819920971479711 ) ) ;
#13962=CARTESIAN_POINT ( 'NONE',  ( 22.06885602671490432, 5.236225869313073211, -3.280147744283338440 ) ) ;
#13965=CARTESIAN_POINT ( 'NONE',  ( 21.85643539959777470, 6.775053487808889940, 8.548204544396675431 ) ) ;
#13966=CARTESIAN_POINT ( 'NONE',  ( 21.69289330443334407, 6.888012688853258680, -2.083760414291091490 ) ) ;
#13967=CARTESIAN_POINT ( 'NONE',  ( 15.45142765023373421, 8.160991103234476185, 3.484307100729007622 ) ) ;
#13970=CARTESIAN_POINT ( 'NONE',  ( 87.41819985312852737, -0.4314763451276128481, -5.556477619079806196 ) ) ;
#13973=CARTESIAN_POINT ( 'NONE',  ( 17.09951025371067246, -3.020100718152188612, 2.875190146946546843 ) ) ;
#13975=CARTESIAN_POINT ( 'NONE',  ( 31.37986798448046954, -3.012493565446135779, -5.103985342590017460 ) ) ;
#13976=CARTESIAN_POINT ( 'NONE',  ( 33.68735618323012204, -3.098775115391426471, -5.464124682821736023 ) ) ;
#13978=CARTESIAN_POINT ( 'NONE',  ( 84.10666795971768295, 3.009888640750769451, -0.3126704449478291403 ) ) ;
#13979=ORIENTED_EDGE ( 'NONE', *, *, #31418, .T. ) ;
#13985=CARTESIAN_POINT ( 'NONE',  ( 36.13231797942587775, -1.531115809672503492, 5.643701445848282816 ) ) ;
#13987=CARTESIAN_POINT ( 'NONE',  ( 33.44795012684379287, -3.712436240568119494, 5.220878576662950188 ) ) ;
#13988=CARTESIAN_POINT ( 'NONE',  ( 86.83780739659150072, -1.126960070541983550, 5.236682382497662047 ) ) ;
#13990=EDGE_CURVE ( 'NONE', #615, #38890, #33909, .T. ) ;
#13992=EDGE_CURVE ( 'NONE', #22597, #17373, #28481, .T. ) ;
#13999=CARTESIAN_POINT ( 'NONE',  ( 23.16222335850500613, 3.880895066624781009, 3.304975045450427196 ) ) ;
#14008=CARTESIAN_POINT ( 'NONE',  ( 22.92160100993126548, 2.713958931179029754, -4.448556569055366339 ) ) ;
#14010=FACE_OUTER_BOUND ( 'NONE', #31840, .T. ) ;
#14012=DIRECTION ( 'NONE',  ( 0.000000000000000000, 0.000000000000000000, 1.000000000000000000 ) ) ;
#14015=CARTESIAN_POINT ( 'NONE',  ( 87.43837438447430088, 0.1427924124619655843, -4.444214939316114332 ) ) ;
#14016=CARTESIAN_POINT ( 'NONE',  ( 33.14263624204154723, -3.231821542972313388, 5.586707398679605419 ) ) ;
#14018=CARTESIAN_POINT ( 'NONE',  ( -71.12440821180588557, -45.61702805680360484, 10.00000000000001066 ) ) ;
#14023=CARTESIAN_POINT ( 'NONE',  ( 32.81190345724319002, -0.8379345996357051574, -5.327489112023386930 ) ) ;
#14031=CARTESIAN_POINT ( 'NONE',  ( 33.66564864975276095, -3.596117103781460766, 5.375233385895072935 ) ) ;
#14040=CARTESIAN_POINT ( 'NONE',  ( 85.41573320709208872, 1.271949590728955970, -5.602497903006397273 ) ) ;
#14045=CARTESIAN_POINT ( 'NONE',  ( 23.74959400416620170, 3.568744068378384426, 3.161886204904667430 ) ) ;
#14049=CARTESIAN_POINT ( 'NONE',  ( 30.76629399850509827, -3.583112896957922899, -4.803821987783259750 ) ) ;
#14052=CARTESIAN_POINT ( 'NONE',  ( 21.99049160266946146, 0.2366918349952460976, 7.677809126247182370 ) ) ;
#14057=CARTESIAN_POINT ( 'NONE',  ( 35.49282083210901817, -3.770656079430354524, -5.543542841511455599 ) ) ;
#14059=DIRECTION ( 'NONE',  ( 0.000000000000000000, 0.000000000000000000, -1.000000000000000000 ) ) ;
#14060=CARTESIAN_POINT ( 'NONE',  ( 29.97903609306309747, -3.796949753938318128, 3.982659670407546759 ) ) ;
#14064=CARTESIAN_POINT ( 'NONE',  ( -79.05190533785294349, -5.483372927171442868, 5.843910349080737809 ) ) ;
#14065=CARTESIAN_POINT ( 'NONE',  ( 22.29617236214320641, 0.2616978831331430166, -7.104760123125566373 ) ) ;
#14069=CARTESIAN_POINT ( 'NONE',  ( 37.18610711987288653, -2.963366855433791525, -5.999999389906995440 ) ) ;
#14083=ORIENTED_EDGE ( 'NONE', *, *, #12229, .F. ) ;
#14084=CARTESIAN_POINT ( 'NONE',  ( 84.47734884986269321, 2.726878650076010491, -2.900369371603537694 ) ) ;
#14092=CARTESIAN_POINT ( 'NONE',  ( -70.92837670882107659, 10.37661300689600097, 0.000000000000000000 ) ) ;
#14096=CARTESIAN_POINT ( 'NONE',  ( 14.51114109149617981, 10.82491507747520387, -2.499999999998495426 ) ) ;
#14099=EDGE_CURVE ( 'NONE', #14684, #20369, #6954, .T. ) ;
#14103=CARTESIAN_POINT ( 'NONE',  ( -17.69482985384421880, -42.37473357531882101, -2.500000000000000000 ) ) ;
#14104=CARTESIAN_POINT ( 'NONE',  ( 21.85643539959774273, 10.54266624894746229, 1.842303177338921572 ) ) ;
#14109=CARTESIAN_POINT ( 'NONE',  ( 14.75671739045200326, -5.151268613661418527, 2.500000000000008438 ) ) ;
#14110=CARTESIAN_POINT ( 'NONE',  ( -75.63216817879452947, -3.684923045591205870, -10.23342513283385635 ) ) ;
#14112=CARTESIAN_POINT ( 'NONE',  ( 34.14251866354382514, -3.850829291023918799, -5.232138609549901176 ) ) ;
#14117=CARTESIAN_POINT ( 'NONE',  ( 31.21728410049454183, -0.3790710272928793922, 5.078610195387921245 ) ) ;
#14122=CARTESIAN_POINT ( 'NONE',  ( 87.15742208552646275, 0.4583713694408729777, 4.797783382239512839 ) ) ;
#14126=CARTESIAN_POINT ( 'NONE',  ( 34.33392167688137420, -1.483023185420157430, 5.565036865347550155 ) ) ;
#14129=CIRCLE ( 'NONE', #1035, 31.65266504832700534 ) ;
#14130=CARTESIAN_POINT ( 'NONE',  ( 85.64504565501374600, 2.098084819171330828, -4.577105872335450520 ) ) ;
#14133=DIRECTION ( 'NONE',  ( 1.385724075720358314E-16, -1.000000000000000000, 0.000000000000000000 ) ) ;
#14137=DIRECTION ( 'NONE',  ( -0.000000000000000000, -0.000000000000000000, -1.000000000000000000 ) ) ;
#14143=B_SPLINE_CURVE_WITH_KNOTS ( 'NONE', 3,
 ( #13799, #33145, #24470, #39917, #5135, #2686, #14789, #30250 ),
 .UNSPECIFIED., .F., .F.,
 ( 4, 2, 2, 4 ),
 ( -2.112996879340024923E-05, 0.0001977261364128406966, 0.0004165822416190816525, 0.0008542944520315643234 ),
 .UNSPECIFIED. ) ;
#14146=LINE ( 'NONE', #16433, #22070 ) ;
#14148=CARTESIAN_POINT ( 'NONE',  ( 23.14899473699292898, 0.4583984410259172027, 5.838797680875789098 ) ) ;
#14155=CARTESIAN_POINT ( 'NONE',  ( -0.7996099067669091287, -29.56993018339339940, -15.49999999999999822 ) ) ;
#14157=CARTESIAN_POINT ( 'NONE',  ( 22.47233723954558471, 4.599796910044377185, -3.286792849618373147 ) ) ;
#14162=CARTESIAN_POINT ( 'NONE',  ( 22.34899403049013245, 4.475801132629629642, -6.347516269785208998 ) ) ;
#14163=AXIS2_PLACEMENT_3D ( 'NONE', #16877, #20370, #30059 ) ;
#14165=CARTESIAN_POINT ( 'NONE',  ( 17.60335251145751911, 11.93951241251601658, 2.500000000000000444 ) ) ;
#14169=CARTESIAN_POINT ( 'NONE',  ( 88.07792789432249947, -1.225918755007668226, 4.438991276806098618 ) ) ;
#14171=DIRECTION ( 'NONE',  ( 1.000000000000000000, 0.000000000000000000, 0.000000000000000000 ) ) ;
#14177=CARTESIAN_POINT ( 'NONE',  ( 21.50439050508445149, -2.639863281018423269, -3.562678242604879753 ) ) ;
#14178=CARTESIAN_POINT ( 'NONE',  ( 36.78868941511550616, -3.039652253131195803, -5.948162739681252198 ) ) ;
#14180=CARTESIAN_POINT ( 'NONE',  ( 25.79188176699440760, 1.042700297243206009, -4.433481499727591313 ) ) ;
#14183=CARTESIAN_POINT ( 'NONE',  ( 37.04507163839541306, -2.801180510112711186, 5.988177386251506640 ) ) ;
#14188=CARTESIAN_POINT ( 'NONE',  ( 37.01009445965782874, -2.248872324984072080, 5.912996221296350718 ) ) ;
#14191=CARTESIAN_POINT ( 'NONE',  ( 86.30432403813082942, -0.2980101775014994958, 5.888268584329271249 ) ) ;
#14198=DIRECTION ( 'NONE',  ( 0.000000000000000000, 0.000000000000000000, -1.000000000000000000 ) ) ;
#14200=CARTESIAN_POINT ( 'NONE',  ( 24.12618649232457102, 3.044573673447521500, 3.674781211205538689 ) ) ;
#14210=CARTESIAN_POINT ( 'NONE',  ( 23.09589271538837352, 2.967069001993269506, -4.168098669102857201 ) ) ;
#14217=CARTESIAN_POINT ( 'NONE',  ( 86.81546468666313388, 0.8424741501213859340, -5.177899619954967392 ) ) ;
#14218=CARTESIAN_POINT ( 'NONE',  ( 33.69128717328723610, -4.440785898112559416, 4.348130384999381981 ) ) ;
#14223=CARTESIAN_POINT ( 'NONE',  ( -75.55143765322812044, -3.604765552797612571, -10.26479841964585127 ) ) ;
#14227=CARTESIAN_POINT ( 'NONE',  ( 36.91755608882559159, -3.049047347627591886, -5.968275500765976460 ) ) ;
#14234=CARTESIAN_POINT ( 'NONE',  ( 36.34368568239760577, -1.915824052793491328, 5.836657992818942375 ) ) ;
#14240=CARTESIAN_POINT ( 'NONE',  ( 86.01948820964511810, 0.2178104211941651880, -5.999583529693873984 ) ) ;
#14246=CARTESIAN_POINT ( 'NONE',  ( 22.87844296631609353, 4.332290514531911718, 3.065998780651157052 ) ) ;
#14253=CARTESIAN_POINT ( 'NONE',  ( 24.74313392016376412, 0.5480228596914666905, 4.780878997086071003 ) ) ;
#14254=CARTESIAN_POINT ( 'NONE',  ( 14.77475711260441393, -5.167191994590148774, -2.499999999999999556 ) ) ;
#14258=CIRCLE ( 'NONE', #24802, 2.500000000000000444 ) ;
#14263=CARTESIAN_POINT ( 'NONE',  ( 82.38753728249152175, 5.816132372599501110, -6.000000000000000888 ) ) ;
#14264=CARTESIAN_POINT ( 'NONE',  ( 26.59415400691353071, 2.826550869980146707, -2.084159418869949043 ) ) ;
#14268=CARTESIAN_POINT ( 'NONE',  ( 21.73396179380037552, 0.2160579277391266595, -9.105503571107611549 ) ) ;
#14270=B_SPLINE_CURVE_WITH_KNOTS ( 'NONE', 3,
 ( #20000, #3981, #35870, #23104, #32582, #16307, #13829, #38524, #13222, #16692 ),
 .UNSPECIFIED., .F., .F.,
 ( 4, 2, 2, 2, 4 ),
 ( 0.000000000000000000, 0.0003911417017416533534, 0.0007822834034833067067, 0.001173425105224960114, 0.001564566806966613413 ),
 .UNSPECIFIED. ) ;
#14274=CARTESIAN_POINT ( 'NONE',  ( 36.44373137833709109, -1.735229189699011743, -5.732540015342363127 ) ) ;
#14289=CARTESIAN_POINT ( 'NONE',  ( 87.90619863186083194, -2.144287391213948624, -2.780224877855328014 ) ) ;
#14299=CARTESIAN_POINT ( 'NONE',  ( 16.08591502891163572, 7.879342335236748873, -3.484773916741195965 ) ) ;
#14303=CARTESIAN_POINT ( 'NONE',  ( -4.444218661349752963, -35.94265729135299381, -6.000000000000000000 ) ) ;
#14305=CARTESIAN_POINT ( 'NONE',  ( 20.16773313137984758, 11.18254505362385132, 2.500000000000000000 ) ) ;
#14306=CARTESIAN_POINT ( 'NONE',  ( 21.85643539959777826, -3.868027658932458479, -14.06783426539529458 ) ) ;
#14308=CARTESIAN_POINT ( 'NONE',  ( 22.61512373101874118, 4.622147853589440913, -3.046406503706223567 ) ) ;
#14310=CARTESIAN_POINT ( 'NONE',  ( -77.75226058499177384, 9.861553516275824549, 8.926870939310843411 ) ) ;
#14311=CARTESIAN_POINT ( 'NONE',  ( 14.76739534775846074, -5.162396215499652996, 2.500000000000008438 ) ) ;
#14312=CARTESIAN_POINT ( 'NONE',  ( -77.74832814377666068, 9.864871290048851549, -8.937781199387956121 ) ) ;
#14321=DIRECTION ( 'NONE',  ( -0.000000000000000000, -0.000000000000000000, -1.000000000000000000 ) ) ;
#14326=CARTESIAN_POINT ( 'NONE',  ( 36.81793901403195690, -2.525225168568379974, 5.952727846996393346 ) ) ;
#14329=CARTESIAN_POINT ( 'NONE',  ( 85.56873805237422914, 2.242856678970356565, 3.827793690346343869 ) ) ;
#14331=CARTESIAN_POINT ( 'NONE',  ( 31.16512824583443475, -0.3608391175596852296, -5.070470012874099375 ) ) ;
#14344=CARTESIAN_POINT ( 'NONE',  ( 22.53023701225289344, 0.9678367267434657695, 6.208473668897325659 ) ) ;
#14346=VERTEX_POINT ( 'NONE', #6950 ) ;
#14356=CARTESIAN_POINT ( 'NONE',  ( 24.39979727116465114, 2.957582978230396176, -3.694537854723473735 ) ) ;
#14359=CARTESIAN_POINT ( 'NONE',  ( 22.82155563815204502, -7.011124981618892527, 0.5620805258418327677 ) ) ;
#14360=CARTESIAN_POINT ( 'NONE',  ( 21.86624219161040372, 3.264102293340572558, -3.922476187580016038 ) ) ;
#14365=CARTESIAN_POINT ( 'NONE',  ( 84.31734228151684363, 3.084090681639994003, 0.3216814846013044127 ) ) ;
#14368=CARTESIAN_POINT ( 'NONE',  ( 28.46177005721402153, 1.600858155335632027, -4.033575672602236928 ) ) ;
#14371=CARTESIAN_POINT ( 'NONE',  ( 28.89404039681430092, -3.378319669541595349, -4.594214991691023542 ) ) ;
#14372=CARTESIAN_POINT ( 'NONE',  ( 36.42059806513616849, -3.113254328073003396, -5.890713182194031283 ) ) ;
#14374=CARTESIAN_POINT ( 'NONE',  ( 21.73603501643664160, 0.2904304739139229596, -8.914614138416270706 ) ) ;
#14375=CARTESIAN_POINT ( 'NONE',  ( 29.69387923751475356, -3.790797245299356799, -4.444098776127088257 ) ) ;
#14377=CARTESIAN_POINT ( 'NONE',  ( 27.40455262169001927, 0.9565157424767126715, 4.483541236861189105 ) ) ;
#14378=CARTESIAN_POINT ( 'NONE',  ( 33.46397865298071395, -3.088978469517898340, -5.429261216816389179 ) ) ;
#14381=EDGE_LOOP ( 'NONE', ( #1310, #16726, #4803, #31475 ) ) ;
#14382=CARTESIAN_POINT ( 'NONE',  ( 37.10502815858426118, -3.127196235056679541, 5.976114625744155084 ) ) ;
#14384=CARTESIAN_POINT ( 'NONE',  ( -70.83040762834239956, -45.61702805680359063, 10.00000000000001066 ) ) ;
#14385=EDGE_CURVE ( 'NONE', #18658, #9338, #19444, .T. ) ;
#14387=ORIENTED_EDGE ( 'NONE', *, *, #34625, .T. ) ;
#14394=CARTESIAN_POINT ( 'NONE',  ( 1.700390093233090871, -29.56993018339339940, 2.499999999999998668 ) ) ;
#14395=EDGE_LOOP ( 'NONE', ( #7168, #4884, #23078, #12190 ) ) ;
#14397=CARTESIAN_POINT ( 'NONE',  ( 21.87278005295215166, 2.930088050433785174, -3.925081081564471663 ) ) ;
#14399=CARTESIAN_POINT ( 'NONE',  ( 24.11465845078392789, 3.025944685091374708, 3.701068920836044995 ) ) ;
#14402=VECTOR ( 'NONE', #27797, 1000.000000000000000 ) ;
#14405=( BOUNDED_SURFACE ( )  B_SPLINE_SURFACE ( 3, 2, ( 
 ( #37917, #23249, #28871 ),
 ( #32725, #13219, #25785 ),
 ( #7981, #31560, #25579 ),
 ( #267, #1434, #36009 ),
 ( #19198, #7788, #13967 ),
 ( #3578, #20339, #26535 ),
 ( #38876, #28671, #39070 ),
 ( #3383, #32918, #9926 ),
 ( #23635, #29816, #6844 ),
 ( #14165, #3779, #678 ),
 ( #12807, #17242, #26737 ),
 ( #38124, #15899, #39275 ),
 ( #11065, #10869, #10668 ),
 ( #22508, #35815, #1627 ),
 ( #7591, #35072, #28460 ),
 ( #20145, #9724, #22305 ),
 ( #19402, #20959, #12082 ),
 ( #5725, #8592, #30648 ) ),
 .UNSPECIFIED., .F., .F., .T. ) 
 B_SPLINE_SURFACE_WITH_KNOTS ( ( 4, 2, 2, 2, 2, 2, 2, 2, 4 ),
 ( 3, 3 ),
 ( 0.1120466800155300452, 0.1143735119802114647, 0.1149552199713818196, 0.1151006469691744083, 0.1151733604680706957, 0.1152460739669669970, 0.1155369279625521745, 0.1167003439448928842, 0.1213540078742557232 ),
 ( 0.000000000000000000, 0.5795136697007319260 ),
 .UNSPECIFIED. ) 
 GEOMETRIC_REPRESENTATION_ITEM ( )  RATIONAL_B_SPLINE_SURFACE ( (
 ( 1.000000000000000000, 0.9576553671123291256, 0.9643893214183871798),
 ( 1.000000000000000000, 0.9576100389905349841, 0.9643512017072020104),
 ( 1.000000000000000000, 0.9575646527973793454, 0.9643130331595894944),
 ( 1.000000000000000000, 0.9575078494902402593, 0.9642652631312538247),
 ( 1.000000000000000000, 0.9574964853007239540, 0.9642557061585608214),
 ( 1.000000000000000000, 0.9574822756861615103, 0.9642437562611960722),
 ( 1.000000000000000000, 0.9574794335443638227, 0.9642413660976467682),
 ( 1.000000000000000000, 0.9574751700039521030, 0.9642377805767230470),
 ( 1.000000000000000000, 0.9574763124065062136, 0.9642387413060384826),
 ( 1.000000000000000000, 0.9574763124065062136, 0.9642387413060384826),
 ( 1.000000000000000000, 0.9574763124065062136, 0.9642387413060387047),
 ( 1.000000000000000000, 0.9574763124065062136, 0.9642387413060387047),
 ( 1.000000000000000000, 0.9574763124065062136, 0.9642387413060384826),
 ( 1.000000000000000000, 0.9574763124065062136, 0.9642387413060384826),
 ( 1.000000000000000000, 0.9574763124065062136, 0.9642387413060384826),
 ( 1.000000000000000000, 0.9574763124065062136, 0.9642387413060384826),
 ( 1.000000000000000000, 0.9574763124065062136, 0.9642387413060384826),
 ( 1.000000000000000000, 0.9574763124065062136, 0.9642387413060384826) ) ) 
 REPRESENTATION_ITEM ( '' )  SURFACE ( )  );
#14407=CARTESIAN_POINT ( 'NONE',  ( 16.12894463104543874, -3.340519685027638186, -2.723709908311349626 ) ) ;
#14410=CARTESIAN_POINT ( 'NONE',  ( 24.56503363824644026, 2.726745707801141894, -3.881485574194932120 ) ) ;
#14417=CARTESIAN_POINT ( 'NONE',  ( -70.92837670882106238, -48.61702805680358352, 6.000000000000002665 ) ) ;
#14419=CARTESIAN_POINT ( 'NONE',  ( 86.23508606437836477, 1.494382965102754923, 4.690504771849753674 ) ) ;
#14420=CARTESIAN_POINT ( 'NONE',  ( 29.75157451403313758, 0.8046206704518127362, -4.785270562610461020 ) ) ;
#14421=CARTESIAN_POINT ( 'NONE',  ( -81.61576440455658599, -5.621349923170992469, -2.262421638520457634 ) ) ;
#14422=CARTESIAN_POINT ( 'NONE',  ( 33.11976541959475639, -3.702904870183194586, 5.168375141609065082 ) ) ;
#14424=CARTESIAN_POINT ( 'NONE',  ( 30.55152536728312285, -0.03400272534400829161, -4.974702443634486215 ) ) ;
#14432=CARTESIAN_POINT ( 'NONE',  ( 36.41835342286016441, -1.780275768523426283, 5.760862909898532891 ) ) ;
#14436=DIRECTION ( 'NONE',  ( 0.000000000000000000, -0.000000000000000000, -1.000000000000000000 ) ) ;
#14438=DIRECTION ( 'NONE',  ( -8.398074759113475787E-17, 1.000000000000000000, 0.000000000000000000 ) ) ;
#14446=CARTESIAN_POINT ( 'NONE',  ( 24.74716371176318219, 3.014745549408870406, 3.371973451314655534 ) ) ;
#14450=ADVANCED_FACE ( 'NONE', ( #30180 ), #36164, .F. ) ;
#14452=VERTEX_POINT ( 'NONE', #2001 ) ;
#14454=CARTESIAN_POINT ( 'NONE',  ( 23.58038339315848120, 0.3885796826799637893, 5.537669914968013529 ) ) ;
#14455=CARTESIAN_POINT ( 'NONE',  ( 14.63804428710352212, -4.770366908001074435, -2.500000000000007550 ) ) ;
#14459=CARTESIAN_POINT ( 'NONE',  ( 35.33400523470628940, -3.787639325471320539, -5.505966337058852744 ) ) ;
#14462=CARTESIAN_POINT ( 'NONE',  ( 29.80812890880734756, -3.278499718192964263, -4.781105184254491824 ) ) ;
#14467=CARTESIAN_POINT ( 'NONE',  ( 26.05868958960777704, 0.7870788155237375960, -4.421617872047712616 ) ) ;
#14470=CARTESIAN_POINT ( 'NONE',  ( 8.290806648384990041, -35.94265729135299381, 6.000000000000000000 ) ) ;
#14473=CARTESIAN_POINT ( 'NONE',  ( 37.10863271423323795, -2.405271516614433835, -5.952050369318877543 ) ) ;
#14474=CARTESIAN_POINT ( 'NONE',  ( 30.67406393699503298, -3.593393542108534344, -4.777508688867102116 ) ) ;
#14477=CARTESIAN_POINT ( 'NONE',  ( -72.42837670882107659, -47.11702805680359063, 38.00000000000000711 ) ) ;
#14490=CARTESIAN_POINT ( 'NONE',  ( 84.89189963960113516, 2.021164017676272184, 4.676249375175704159 ) ) ;
#14496=CARTESIAN_POINT ( 'NONE',  ( 23.14867680946094097, 4.061912727637136733, 3.041127315635880901 ) ) ;
#14502=CARTESIAN_POINT ( 'NONE',  ( 15.21972607795940391, 10.50943668950837839, -2.499999999997734701 ) ) ;
#14507=ORIENTED_EDGE ( 'NONE', *, *, #28267, .T. ) ;
#14508=CARTESIAN_POINT ( 'NONE',  ( 21.85643539959778181, 2.105182337828026995, -13.78739850581801996 ) ) ;
#14512=CARTESIAN_POINT ( 'NONE',  ( 14.70276859592049057, -4.942772565485702430, 2.499999999999277911 ) ) ;
#14513=CARTESIAN_POINT ( 'NONE',  ( -79.87450223356385948, 10.49415034902278698, -4.486381563923941052 ) ) ;
#14524=CARTESIAN_POINT ( 'NONE',  ( 88.04454721149249963, -0.5380896775427260748, 2.907127687869381916 ) ) ;
#14528=CARTESIAN_POINT ( 'NONE',  ( 35.86997984655084792, -2.084313029741385659, 5.804775892431827344 ) ) ;
#14530=CARTESIAN_POINT ( 'NONE',  ( 85.64278173364962754, 1.868356560669967470, -5.099220668941490509 ) ) ;
#14541=CARTESIAN_POINT ( 'NONE',  ( 26.54964660807501531, 1.667999962647538359, 4.320834639766450991 ) ) ;
#14544=B_SPLINE_CURVE_WITH_KNOTS ( 'NONE', 3,
 ( #10320, #39122, #16495, #28868, #29072, #13215, #878, #35466, #7238, #10518, #36061, #38721, #23098, #19801, #675, #38921, #10919, #20190, #26391, #13410, #10713, #13616, #32372, #25985, #29664, #23292, #38517 ),
 .UNSPECIFIED., .F., .F.,
 ( 4, 1, 2, 2, 1, 1, 1, 1, 2, 2, 1, 1, 1, 1, 1, 2, 2, 1, 4 ),
 ( 0.07055524994525608218, 0.1867358437020780471, 0.2448261405804889046, 0.2738712890196948191, 0.3029164374589006781, 0.4190970312157243916, 0.4771873280941357209, 0.4917099023137387892, 0.4989711894235402401, 0.5007865112009901587, 0.5026018329784399663, 0.5062324765333394705, 0.5352776249725555990, 0.6514582187294180038, 0.7095485156078492617, 0.7385936640470648351, 0.7531162382666727328, 0.7676388124862805196, 1.000000000000000000 ),
 .UNSPECIFIED. ) ;
#14548=CARTESIAN_POINT ( 'NONE',  ( 36.10284116201629701, 0.9159659085930716982, -6.000000000000000000 ) ) ;
#14552=CARTESIAN_POINT ( 'NONE',  ( 22.17125346225300575, 4.446648860891334820, -3.726893279828063843 ) ) ;
#14555=CARTESIAN_POINT ( 'NONE',  ( 22.76577552469399990, -5.388071312449273620, 6.143773694815460651 ) ) ;
#14559=CARTESIAN_POINT ( 'NONE',  ( 85.39132736373097998, 1.761725527925377399, -5.190388716534374502 ) ) ;
#14560=CARTESIAN_POINT ( 'NONE',  ( 8.290806648384990041, -35.94265729135299381, 2.500000000000000000 ) ) ;
#14562=CARTESIAN_POINT ( 'NONE',  ( 26.98979804764019264, 2.155375236454192933, -3.758468440649340714 ) ) ;
#14564=CARTESIAN_POINT ( 'NONE',  ( 22.18104894856640996, 5.504333011849090518, -2.539813209877764155 ) ) ;
#14565=CARTESIAN_POINT ( 'NONE',  ( 15.25857687985927136, -3.898425631526794000, -2.584722552834652465 ) ) ;
#14566=CARTESIAN_POINT ( 'NONE',  ( 36.14130771815730725, -3.140490948321353670, -5.847123168885349997 ) ) ;
#14568=CARTESIAN_POINT ( 'NONE',  ( 25.67091747518093570, 1.146822820001185184, -4.432699664903578807 ) ) ;
#14578=CARTESIAN_POINT ( 'NONE',  ( 33.45688159892293356, -3.834031077008411614, 5.088667958700237470 ) ) ;
#14580=CARTESIAN_POINT ( 'NONE',  ( 22.10870846509921250, -3.077893895552592074, -3.560816367895537127 ) ) ;
#14590=CARTESIAN_POINT ( 'NONE',  ( 14.75868448971168512, -5.144185890768196323, 2.500012889186591813 ) ) ;
#14593=CARTESIAN_POINT ( 'NONE',  ( 21.88711032996733863, 3.208699644456277866, -3.395463446387114725 ) ) ;
#14595=CARTESIAN_POINT ( 'NONE',  ( 22.00057757746165166, 4.523971029709453973, 3.846587773178183678 ) ) ;
#14599=CARTESIAN_POINT ( 'NONE',  ( 26.17280925958501214, -2.761831904353556411, -4.291297895378931138 ) ) ;
#14600=DIRECTION ( 'NONE',  ( 0.000000000000000000, 0.000000000000000000, 1.000000000000000000 ) ) ;
#14602=ORIENTED_EDGE ( 'NONE', *, *, #36087, .T. ) ;
#14603=CARTESIAN_POINT ( 'NONE',  ( 22.48581518839592874, 2.618461469189475199, -4.833321383114350667 ) ) ;
#14604=ORIENTED_EDGE ( 'NONE', *, *, #24443, .F. ) ;
#14611=CARTESIAN_POINT ( 'NONE',  ( 86.07545474579461597, 1.673688438695506431, -4.651254279175787154 ) ) ;
#14612=CARTESIAN_POINT ( 'NONE',  ( 29.24680661740138632, 2.095232292622827508, -1.948189103474716966 ) ) ;
#14615=CARTESIAN_POINT ( 'NONE',  ( 19.72131146634190557, -3.044362691710549296, 3.219876361117069763 ) ) ;
#14616=CARTESIAN_POINT ( 'NONE',  ( -4.224659823956008253, -51.67615071827237472, -6.000000000000000000 ) ) ;
#14617=CARTESIAN_POINT ( 'NONE',  ( 29.17646580786398758, 0.5759241497138282151, -4.760091143445980499 ) ) ;
#14624=CARTESIAN_POINT ( 'NONE',  ( -72.84815947045233031, 2.429809908903243443, -12.50000000000000000 ) ) ;
#14627=CARTESIAN_POINT ( 'NONE',  ( 33.68482843757833223, -3.836899954132453772, 5.141354644792926365 ) ) ;
#14631=EDGE_CURVE ( 'NONE', #20444, #3707, #413, .T. ) ;
#14638=CARTESIAN_POINT ( 'NONE',  ( -74.68498725152623763, 9.372166970630278371, 9.273481029445454382 ) ) ;
#14641=ORIENTED_EDGE ( 'NONE', *, *, #37075, .T. ) ;
#14642=CARTESIAN_POINT ( 'NONE',  ( 22.87956138668360495, 4.318478688965076806, 3.085875429863905950 ) ) ;
#14649=CARTESIAN_POINT ( 'NONE',  ( 21.78202853633694502, 0.2105828418074676689, 8.406744294290200870 ) ) ;
#14650=CARTESIAN_POINT ( 'NONE',  ( 14.75163840144606020, -5.120888621327094548, -2.500049689809528797 ) ) ;
#14659=CARTESIAN_POINT ( 'NONE',  ( 87.04213330793392345, 0.5878691963682337596, -6.000000000000000000 ) ) ;
#14660=CARTESIAN_POINT ( 'NONE',  ( 26.86540377008237357, 1.668949755151340586, -4.708546860826485769 ) ) ;
#14663=ORIENTED_EDGE ( 'NONE', *, *, #18792, .F. ) ;
#14665=CARTESIAN_POINT ( 'NONE',  ( 27.41552500817463667, 1.019591371738703955, -4.485159083204544928 ) ) ;
#14673=CARTESIAN_POINT ( 'NONE',  ( 37.00886176876311140, -2.250709667194641828, -5.913644327890312802 ) ) ;
#14678=LINE ( 'NONE', #7906, #22694 ) ;
#14681=CARTESIAN_POINT ( 'NONE',  ( 14.75069249142107886, -5.116492627577003738, -2.500060313030776804 ) ) ;
#14682=CARTESIAN_POINT ( 'NONE',  ( 23.33329484996965419, 2.006436124235808638, -4.751833140929669241 ) ) ;
#14684=VERTEX_POINT ( 'NONE', #22158 ) ;
#14699=CARTESIAN_POINT ( 'NONE',  ( 16.50401505813599101, 9.937674115411510911, -2.499999999999894751 ) ) ;
#14704=CARTESIAN_POINT ( 'NONE',  ( 14.82981423308607560, 12.75311901897797107, -2.505853893009207578 ) ) ;
#14706=CARTESIAN_POINT ( 'NONE',  ( 21.85643539959774273, 10.58808081918846256, 0.01331417752983106093 ) ) ;
#14709=CARTESIAN_POINT ( 'NONE',  ( 14.68624896554715598, -4.761818446054777887, 2.499999999999112266 ) ) ;
#14711=CARTESIAN_POINT ( 'NONE',  ( -75.05634802856252463, 7.993964939743821496, -10.46629622540592308 ) ) ;
#14717=CARTESIAN_POINT ( 'NONE',  ( -70.66690635095469020, 0.1910696742817396265, 9.997314914349638926 ) ) ;
#14726=ORIENTED_EDGE ( 'NONE', *, *, #3218, .T. ) ;
#14730=CARTESIAN_POINT ( 'NONE',  ( 86.60363381072151867, 0.9779648536402296699, 5.693185077828528229 ) ) ;
#14731=CARTESIAN_POINT ( 'NONE',  ( 29.28314298262022319, 1.964681093867868933, 2.525543949525632659 ) ) ;
#14746=CARTESIAN_POINT ( 'NONE',  ( 26.00408895386407693, 0.8598023161378668400, 4.425818499699599506 ) ) ;
#14748=ORIENTED_EDGE ( 'NONE', *, *, #8317, .F. ) ;
#14758=CARTESIAN_POINT ( 'NONE',  ( 22.21474492361291908, 5.152987084292143471, -3.146772455935926693 ) ) ;
#14759=ORIENTED_EDGE ( 'NONE', *, *, #8812, .T. ) ;
#14761=CARTESIAN_POINT ( 'NONE',  ( 23.99854160108877110, 3.116918725036224025, -4.608611027060286247 ) ) ;
#14764=CARTESIAN_POINT ( 'NONE',  ( -70.92837670882107659, -65.19654454972992141, 6.000000000000002665 ) ) ;
#14766=CARTESIAN_POINT ( 'NONE',  ( 85.00114435706898064, 2.071954908684588759, 4.651167869591634307 ) ) ;
#14767=CARTESIAN_POINT ( 'NONE',  ( 17.03294222275471270, 9.497926725977514195, 2.806642516075366078 ) ) ;
#14769=CARTESIAN_POINT ( 'NONE',  ( -70.92837670882107659, 3.729367930467589076, 0.000000000000000000 ) ) ;
#14774=CARTESIAN_POINT ( 'NONE',  ( 14.88813598356257195, -6.116304347389402984, -2.529251432410653422 ) ) ;
#14776=CARTESIAN_POINT ( 'NONE',  ( 22.91741166320089818, 2.643276093639356006, -3.783214368374389291 ) ) ;
#14778=VECTOR ( 'NONE', #3025, 1000.000000000000000 ) ;
#14787=CARTESIAN_POINT ( 'NONE',  ( 33.94748962458718466, -0.4853907904003012530, 5.118178450053537887 ) ) ;
#14789=CARTESIAN_POINT ( 'NONE',  ( 14.61802081865039682, 12.48098255133728784, -2.499999999999999556 ) ) ;
#14794=LINE ( 'NONE', #27364, #6909 ) ;
#14796=B_SPLINE_CURVE_WITH_KNOTS ( 'NONE', 3,
 ( #36549, #14305, #26680, #33486, #20902, #5464, #11410, #36153, #30168, #24398, #18004, #8118, #17797, #17189, #14923, #30383, #27492, #29964, #21115, #23589, #1571, #20690, #33273, #1775 ),
 .UNSPECIFIED., .F., .F.,
 ( 4, 1, 1, 1, 1, 1, 1, 2, 2, 1, 1, 1, 1, 1, 1, 2, 2, 4 ),
 ( 0.000000000000000000, 0.2499999999999679146, 0.3749999999999522049, 0.4374999999999445999, 0.4687499999999411027, 0.4843749999999393818, 0.4921874999999382716, 0.4960937499999385492, 0.4999999999999388267, 0.6249999999999987788, 0.6875000000000288658, 0.7187500000000447420, 0.7343750000000527356, 0.7421875000000558442, 0.7460937500000575096, 0.7480468750000581757, 0.7500000000000589528, 1.000000000000000000 ),
 .UNSPECIFIED. ) ;
#14808=CARTESIAN_POINT ( 'NONE',  ( 17.64783264544855257, -2.926693510814210697, -2.960769117404401740 ) ) ;
#14812=CARTESIAN_POINT ( 'NONE',  ( 23.49894466845412566, 3.019249802179449826, -3.929487204937235134 ) ) ;
#14819=PLANE ( 'NONE',  #12292 ) ;
#14821=CARTESIAN_POINT ( 'NONE',  ( 86.83829259450851623, 0.8168327605515373069, 4.998615091244022146 ) ) ;
#14825=CARTESIAN_POINT ( 'NONE',  ( 14.85476021617353304, -4.543106551388008896, 2.514844559792396517 ) ) ;
#14828=CARTESIAN_POINT ( 'NONE',  ( 36.42092789943291820, -3.115845811384692077, -5.890764660813112563 ) ) ;
#14836=CARTESIAN_POINT ( 'NONE',  ( 35.83209424069072924, -3.726939881646061270, 5.625185406441244318 ) ) ;
#14841=PLANE ( 'NONE',  #25352 ) ;
#14844=CARTESIAN_POINT ( 'NONE',  ( -80.32062948810629166, -6.645441929077266607, -3.458186301391593886 ) ) ;
#14851=CARTESIAN_POINT ( 'NONE',  ( 22.19529100421578960, 5.229607391819558693, 3.102197625450730634 ) ) ;
#14857=CARTESIAN_POINT ( 'NONE',  ( 21.97060183119601007, 0.2202240153287075564, 7.735562088727589547 ) ) ;
#14858=CARTESIAN_POINT ( 'NONE',  ( 14.75808067079221431, -5.143087478482986974, -2.500015154099217707 ) ) ;
#14869=CARTESIAN_POINT ( 'NONE',  ( 30.37020714367901775, -0.1410433206546675144, -5.583699017444894608 ) ) ;
#14874=CARTESIAN_POINT ( 'NONE',  ( 24.12552690779179798, 0.5099362638223552402, -5.092848330633646725 ) ) ;
#14879=CARTESIAN_POINT ( 'NONE',  ( -71.12492995964747422, -48.60730761282789558, 9.998528757544843160 ) ) ;
#14881=CARTESIAN_POINT ( 'NONE',  ( 34.79194643261769926, -3.831294807337672914, -5.380493905816994271 ) ) ;
#14882=CARTESIAN_POINT ( 'NONE',  ( 30.84634820625675644, -3.378268544268043350, -4.954352808572474842 ) ) ;
#14888=CARTESIAN_POINT ( 'NONE',  ( -74.02422384641097608, 6.646861260247477254, 10.77237409516136424 ) ) ;
#14890=CARTESIAN_POINT ( 'NONE',  ( 14.77222818450456643, -4.461908109758233820, -2.511961494517393145 ) ) ;
#14891=CARTESIAN_POINT ( 'NONE',  ( 22.53677427111851372, 1.671346796043067462, -5.585631968908431944 ) ) ;
#14895=PLANE ( 'NONE',  #23871 ) ;
#14898=AXIS2_PLACEMENT_3D ( 'NONE', #13521, #26092, #33281 ) ;
#14900=CARTESIAN_POINT ( 'NONE',  ( 87.05329302184628659, -1.423768201249274945, 4.835531253876708568 ) ) ;
#14903=CIRCLE ( 'NONE', #6375, 0.9999999999999971134 ) ;
#14912=CARTESIAN_POINT ( 'NONE',  ( 22.61586509580334337, 4.626878386862768089, 3.038062468280299022 ) ) ;
#14914=CARTESIAN_POINT ( 'NONE',  ( 22.16976678648915922, -3.079849535211031331, 3.569519670046482407 ) ) ;
#14918=CARTESIAN_POINT ( 'NONE',  ( 17.02720468749124905, 12.19482429969091619, -2.499999999999998668 ) ) ;
#14921=ADVANCED_FACE ( 'NONE', ( #22563 ), #7300, .T. ) ;
#14922=CARTESIAN_POINT ( 'NONE',  ( 22.91153608851413637, 3.594015725306300979, 3.782297342843620847 ) ) ;
#14923=CARTESIAN_POINT ( 'NONE',  ( 17.53293928993041106, 14.12932500356599164, 2.499999999999999556 ) ) ;
#14924=CARTESIAN_POINT ( 'NONE',  ( 21.85643539959774273, 9.214175136349357587, -0.8338435668127727185 ) ) ;
#14926=CARTESIAN_POINT ( 'NONE',  ( -76.92986009040373574, 10.85203011506569304, 8.001236914947885026 ) ) ;
#14929=CIRCLE ( 'NONE', #24820, 7.744449365083023729 ) ;
#14930=CARTESIAN_POINT ( 'NONE',  ( -74.64436830331966632, 7.527181902581737916, -9.332964955005275343 ) ) ;
#14934=CARTESIAN_POINT ( 'NONE',  ( 14.98917483460526512, 12.12204619583915566, 2.538718705410484500 ) ) ;
#14941=CARTESIAN_POINT ( 'NONE',  ( 87.24249188000140975, 0.3628169386305434840, 4.705374253625543624 ) ) ;
#14942=CARTESIAN_POINT ( 'NONE',  ( 24.72992518470875112, 2.633077311188870340, -3.926889863206841191 ) ) ;
#14945=CARTESIAN_POINT ( 'NONE',  ( 36.66725829508891366, -2.423845347316893939, 5.929210476578201217 ) ) ;
#14949=CARTESIAN_POINT ( 'NONE',  ( 86.10913233486274976, 1.283334762834210441, -5.698406565159564785 ) ) ;
#14956=ORIENTED_EDGE ( 'NONE', *, *, #29478, .T. ) ;
#14959=VERTEX_POINT ( 'NONE', #22964 ) ;
#14966=ORIENTED_EDGE ( 'NONE', *, *, #30612, .F. ) ;
#14969=ADVANCED_FACE ( 'NONE', ( #33240 ), #32640, .T. ) ;
#14972=EDGE_CURVE ( 'NONE', #23738, #1317, #30143, .T. ) ;
#14974=CARTESIAN_POINT ( 'NONE',  ( 4.938390203311415748E-15, -42.37473357531882101, 6.000000000000000000 ) ) ;
#14977=CARTESIAN_POINT ( 'NONE',  ( 23.73069679916937602, 3.541948203740225232, -3.238583379989644850 ) ) ;
#14980=CARTESIAN_POINT ( 'NONE',  ( 24.33615536228354514, 0.1518143133650739496, -6.924920736309362113 ) ) ;
#14984=CARTESIAN_POINT ( 'NONE',  ( 84.44530234979703209, 2.765803402995568927, 2.732740112990733383 ) ) ;
#14989=CARTESIAN_POINT ( 'NONE',  ( -70.92837670882107659, -45.61702805680359063, 10.00000000000000888 ) ) ;
#14992=CARTESIAN_POINT ( 'NONE',  ( 23.82764572543298698, -2.864586094091185586, -3.920064517359787892 ) ) ;
#14996=CARTESIAN_POINT ( 'NONE',  ( 33.46307027370517062, -3.080941673966315797, 5.429119442261287176 ) ) ;
#14997=CARTESIAN_POINT ( 'NONE',  ( 88.10293741339057760, -0.6036763236807990429, 2.641732887311516453 ) ) ;
#15001=CARTESIAN_POINT ( 'NONE',  ( 36.49386420176196566, -3.561635646996995419, 5.795649267797439386 ) ) ;
#15002=CARTESIAN_POINT ( 'NONE',  ( 26.15460830059191011, -2.761060381110045814, 4.288457195536199862 ) ) ;
#15003=CARTESIAN_POINT ( 'NONE',  ( 17.86011303457873467, -3.180593380899296108, -2.952765578688846038 ) ) ;
#15005=ORIENTED_EDGE ( 'NONE', *, *, #19261, .F. ) ;
#15007=ORIENTED_EDGE ( 'NONE', *, *, #25306, .F. ) ;
#15013=CARTESIAN_POINT ( 'NONE',  ( 24.06016172912751472, 2.745221661300574656, 3.954363946542386987 ) ) ;
#15014=CARTESIAN_POINT ( 'NONE',  ( 31.35971567531513315, 0.5160385187742575486, 4.592137409821144267 ) ) ;
#15022=DIRECTION ( 'NONE',  ( 0.000000000000000000, -1.000000000000000000, 0.000000000000000000 ) ) ;
#15025=CARTESIAN_POINT ( 'NONE',  ( 23.72685993228412471, 2.962434847395911230, -3.894494263829419545 ) ) ;
#15028=CARTESIAN_POINT ( 'NONE',  ( 21.85643539959781023, -13.06032977194142930, 9.178732910485948082 ) ) ;
#15029=FACE_BOUND ( 'NONE', #9586, .T. ) ;
#15034=CARTESIAN_POINT ( 'NONE',  ( 87.34032947353671261, 0.2529211099193515166, 5.122688537971352929 ) ) ;
#15039=AXIS2_PLACEMENT_3D ( 'NONE', #38914, #25978, #13815 ) ;
#15040=CARTESIAN_POINT ( 'NONE',  ( 36.91185272694033870, -2.638231765404660312, -5.967385353207440346 ) ) ;
#15046=CARTESIAN_POINT ( 'NONE',  ( -69.42837670882104817, -46.91912102050241629, 5.809475019311127753 ) ) ;
#15048=CARTESIAN_POINT ( 'NONE',  ( 37.15673189557763578, -2.580998988453131027, 5.983779168937476634 ) ) ;
#15049=B_SPLINE_CURVE_WITH_KNOTS ( 'NONE', 3,
 ( #5861, #6063, #31588, #3412 ),
 .UNSPECIFIED., .F., .F.,
 ( 4, 4 ),
 ( 0.000000000000000000, 0.6850855086804076288 ),
 .UNSPECIFIED. ) ;
#15054=EDGE_CURVE ( 'NONE', #6497, #1317, #10735, .T. ) ;
#15057=CARTESIAN_POINT ( 'NONE',  ( -79.81323911311395136, -6.649679829688860622, -4.608218461864638904 ) ) ;
#15058=CARTESIAN_POINT ( 'NONE',  ( 21.29228973259959901, 5.334523051338725175, 3.529574787382050882 ) ) ;
#15059=B_SPLINE_SURFACE_WITH_KNOTS ( 'NONE', 3, 3, ( 
 ( #3034, #40249, #28106, #40661 ),
 ( #23988, #11623, #2197, #33694 ),
 ( #6091, #18624, #31213, #37168 ),
 ( #24410, #17807, #15552, #36967 ),
 ( #5473, #27289, #36558, #30392 ),
 ( #39854, #2413, #31013, #20912 ),
 ( #34117, #36761, #8547, #15342 ),
 ( #18016, #30813, #21127, #2818 ),
 ( #30604, #40443, #14934, #27898 ),
 ( #40053, #11827, #27693, #8746 ),
 ( #21331, #8954, #33905, #5679 ),
 ( #12252, #2618, #24824, #12035 ),
 ( #7102, #38180, #22365, #37980 ),
 ( #3639, #16359, #31825, #16164 ),
 ( #19665, #28728, #19256, #540 ),
 ( #3842, #6708, #18845, #6905 ),
 ( #25638, #13076, #22562, #10178 ),
 ( #15759, #32239, #9983, #35127 ),
 ( #12663, #19461, #19056, #25238 ),
 ( #4039, #32035, #28933, #34519 ),
 ( #16555, #28314, #25842, #35333 ),
 ( #734, #37769, #12871, #21947 ),
 ( #25435, #31415, #34728, #3242 ),
 ( #6296, #13271, #132, #31619 ),
 ( #12463, #6508, #38376, #9576 ) ),
 .UNSPECIFIED., .F., .F., .F.,
 ( 4, 3, 3, 3, 3, 3, 3, 3, 4 ),
 ( 4, 4 ),
 ( 0.003645227204780212768, 0.004012130669716890488, 0.004379034134653567341, 0.005112841064526921914, 0.006580454924273630192, 0.008048068784020338470, 0.009515682643767047616, 0.01245091036326046417, 0.01538613808275388073 ),
 ( 0.000000000000000000, 1.006050268738574616 ),
 .UNSPECIFIED. ) ;
#15062=EDGE_LOOP ( 'NONE', ( #11973, #30357, #27354, #25981, #5346, #38055, #29026, #18038, #15886, #27128, #18887, #2957 ) ) ;
#15063=CARTESIAN_POINT ( 'NONE',  ( 24.34017676013632325, 3.136949483460702570, 3.398357025751408855 ) ) ;
#15071=CARTESIAN_POINT ( 'NONE',  ( 26.06250554953703613, 0.7788941295968891954, 4.421378155111866270 ) ) ;
#15072=CARTESIAN_POINT ( 'NONE',  ( 14.75748024341934439, -4.578899578309257201, -2.509460294425407412 ) ) ;
#15078=CARTESIAN_POINT ( 'NONE',  ( -7.890026461918812295, -8.913725925455491250, -6.000000000000000000 ) ) ;
#15080=CARTESIAN_POINT ( 'NONE',  ( 29.21535032918476915, 2.216127810226045547, -1.021449648108430086 ) ) ;
#15081=CARTESIAN_POINT ( 'NONE',  ( 14.74047039395649605, -5.121629765571634074, -2.499999999999999556 ) ) ;
#15084=CARTESIAN_POINT ( 'NONE',  ( 24.72931927919737660, 0.6236087402561421023, -4.781898317253668651 ) ) ;
#15090=CARTESIAN_POINT ( 'NONE',  ( 36.39222352889621703, -1.827525151019651517, -5.788514553718531630 ) ) ;
#15092=CARTESIAN_POINT ( 'NONE',  ( -70.92837670882107659, -23.80776546975053520, 10.00000000000000533 ) ) ;
#15099=CARTESIAN_POINT ( 'NONE',  ( 14.73622163650396999, -5.027757633256064729, -2.500471392631596235 ) ) ;
#15100=CARTESIAN_POINT ( 'NONE',  ( 23.91523202801653269, 2.089873375604069494, -4.428822888773534139 ) ) ;
#15116=CARTESIAN_POINT ( 'NONE',  ( 24.41296328559054984, 3.167430643262210133, 3.253911296061570368 ) ) ;
#15122=CARTESIAN_POINT ( 'NONE',  ( 15.78341776548205111, 8.012724091073605948, -3.484800346807145566 ) ) ;
#15128=CARTESIAN_POINT ( 'NONE',  ( 21.85643539959775339, -5.954433958055524556, -11.26730592371362505 ) ) ;
#15130=CARTESIAN_POINT ( 'NONE',  ( -80.85577149014498843, 10.55954795747387820, 1.459777158011418496 ) ) ;
#15134=CARTESIAN_POINT ( 'NONE',  ( 28.22828621824402973, -3.406067573266987392, -4.612104786675601531 ) ) ;
#15135=CARTESIAN_POINT ( 'NONE',  ( 27.81756494040502048, 1.846260971994820199, -3.902053172858347185 ) ) ;
#15143=CARTESIAN_POINT ( 'NONE',  ( 37.13687059807102031, -2.464987586452376256, -5.964471309820316591 ) ) ;
#15144=CARTESIAN_POINT ( 'NONE',  ( 26.61436230569603723, 1.627489583404493345, -4.333517427382849618 ) ) ;
#15148=CARTESIAN_POINT ( 'NONE',  ( 32.84220568043447486, -0.7495606313452212177, 5.332218506814426995 ) ) ;
#15152=PRODUCT_DEFINITION ( 'UNKNOWN', '', #28109, #36584 ) ;
#15153=CARTESIAN_POINT ( 'NONE',  ( 88.90249899953845159, -1.697492344831515121, -0.8687328377452782080 ) ) ;
#15155=CARTESIAN_POINT ( 'NONE',  ( 29.20166386951125048, 2.268204792580242213, 0.006282727923920283265 ) ) ;
#15156=CARTESIAN_POINT ( 'NONE',  ( 35.95119605051105083, -2.121419093699826952, -5.817451645281153993 ) ) ;
#15173=DIRECTION ( 'NONE',  ( -0.000000000000000000, -0.000000000000000000, -1.000000000000000000 ) ) ;
#15176=CARTESIAN_POINT ( 'NONE',  ( 23.72115022044104293, 3.525691739180937923, -3.279221235023926262 ) ) ;
#15180=CARTESIAN_POINT ( 'NONE',  ( 26.75871784592184710, 2.055338430770167424, -4.125980934060708982 ) ) ;
#15184=CARTESIAN_POINT ( 'NONE',  ( 88.16134551068515179, -2.448791080374484341, 0.2153404935567143075 ) ) ;
#15185=CARTESIAN_POINT ( 'NONE',  ( 14.77315594796471743, 13.19392823276620419, 2.499999999999996891 ) ) ;
#15192=CARTESIAN_POINT ( 'NONE',  ( 33.95701888394219736, -3.573114794754973733, -5.438351141695983770 ) ) ;
#15193=CARTESIAN_POINT ( 'NONE',  ( 32.77851786469086903, -0.9351265186074488867, -5.322278482871990235 ) ) ;
#15198=CARTESIAN_POINT ( 'NONE',  ( 22.91836776944852261, 2.645787328278193851, 3.783363591877844101 ) ) ;
#15202=CARTESIAN_POINT ( 'NONE',  ( 87.04213330793400871, 0.5878691963681530464, -4.891134986362597914 ) ) ;
#15203=ORIENTED_EDGE ( 'NONE', *, *, #21675, .T. ) ;
#15206=CARTESIAN_POINT ( 'NONE',  ( 36.68582491073361496, -1.914190917646145129, 5.802815688716031595 ) ) ;
#15207=CARTESIAN_POINT ( 'NONE',  ( 15.79641112846907625, -3.685450897386115532, -2.654044247040655335 ) ) ;
#15208=CARTESIAN_POINT ( 'NONE',  ( 14.71640407929426964, 12.89631605134570691, -2.500000000000019096 ) ) ;
#15209=EDGE_LOOP ( 'NONE', ( #13914, #39900, #27569 ) ) ;
#15210=DIRECTION ( 'NONE',  ( 0.000000000000000000, 0.000000000000000000, 1.000000000000000000 ) ) ;
#15211=VERTEX_POINT ( 'NONE', #34280 ) ;
#15216=ORIENTED_EDGE ( 'NONE', *, *, #40287, .F. ) ;
#15217=CARTESIAN_POINT ( 'NONE',  ( 24.34875050026406029, 2.411635393770941604, 4.109526650664126812 ) ) ;
#15218=CARTESIAN_POINT ( 'NONE',  ( 21.52272803504227383, 7.572183114303116191, -2.831506016415840321 ) ) ;
#15219=ORIENTED_EDGE ( 'NONE', *, *, #29796, .F. ) ;
#15229=CARTESIAN_POINT ( 'NONE',  ( 23.97548348472609092, 2.871991460080824066, -3.880200249615740393 ) ) ;
#15230=ORIENTED_EDGE ( 'NONE', *, *, #20088, .F. ) ;
#15231=LINE ( 'NONE', #27785, #25069 ) ;
#15233=CARTESIAN_POINT ( 'NONE',  ( 21.85643539959775694, 4.302923821179891029, -14.48878861646959315 ) ) ;
#15237=CARTESIAN_POINT ( 'NONE',  ( 88.66415851257785619, -1.234066499448195131, -0.8261491842984883816 ) ) ;
#15238=CARTESIAN_POINT ( 'NONE',  ( 29.28314298262022319, 1.964681093867868933, 2.525543949525632659 ) ) ;
#15240=CARTESIAN_POINT ( 'NONE',  ( 31.36171663430588197, -3.287353811999296660, 5.090714763224706729 ) ) ;
#15241=CARTESIAN_POINT ( 'NONE',  ( -89.00859394718983708, 2.429809908903242555, -12.50000000000000000 ) ) ;
#15243=CARTESIAN_POINT ( 'NONE',  ( 36.44757542402881256, -2.353335513535177448, -5.894923651499230921 ) ) ;
#15246=FACE_OUTER_BOUND ( 'NONE', #30256, .T. ) ;
#15248=CARTESIAN_POINT ( 'NONE',  ( 21.85643539959777115, -33.54387950140291963, 2.500000000000000000 ) ) ;
#15252=ORIENTED_EDGE ( 'NONE', *, *, #37599, .F. ) ;
#15253=CARTESIAN_POINT ( 'NONE',  ( 33.67928082117678201, -3.778927839680616518, 5.203631254605035394 ) ) ;
#15254=( BOUNDED_SURFACE ( )  B_SPLINE_SURFACE ( 3, 2, ( 
 ( #23008, #37818, #34978 ),
 ( #31465, #31669, #3485 ),
 ( #6753, #3685, #16209 ),
 ( #13126, #25685, #7344 ) ),
 .UNSPECIFIED., .F., .F., .T. ) 
 B_SPLINE_SURFACE_WITH_KNOTS ( ( 4, 4 ),
 ( 3, 3 ),
 ( 0.005270629645086826603, 0.007540928297313504239 ),
 ( 0.000000000000000000, 1.000000000000000000 ),
 .UNSPECIFIED. ) 
 GEOMETRIC_REPRESENTATION_ITEM ( )  RATIONAL_B_SPLINE_SURFACE ( (
 ( 1.000000000000000000, 0.8929511290151087577, 1.000000000000000000),
 ( 1.000000000000000000, 0.8751608305411335831, 1.000000000000000000),
 ( 1.000000000000000000, 0.8609515519834827213, 1.000000000000000000),
 ( 1.000000000000000000, 0.8503725744608083836, 1.000000000000000000) ) ) 
 REPRESENTATION_ITEM ( '' )  SURFACE ( )  );
#15257=CARTESIAN_POINT ( 'NONE',  ( -71.43139732235886186, 0.09104805635102961037, 9.988066921647986263 ) ) ;
#15266=ORIENTED_EDGE ( 'NONE', *, *, #19381, .F. ) ;
#15267=CARTESIAN_POINT ( 'NONE',  ( 24.35304765632307067, 3.141127394751760615, 3.377496490332608126 ) ) ;
#15279=ORIENTED_EDGE ( 'NONE', *, *, #19262, .F. ) ;
#15283=ORIENTED_EDGE ( 'NONE', *, *, #32006, .T. ) ;
#15287=CARTESIAN_POINT ( 'NONE',  ( 31.36201648005763332, -1.233860125724708379, -5.969386505766030915 ) ) ;
#15291=CARTESIAN_POINT ( 'NONE',  ( 21.73499591390137908, 0.2555434075777953118, -9.002945845404971337 ) ) ;
#15293=ORIENTED_EDGE ( 'NONE', *, *, #19677, .T. ) ;
#15297=CARTESIAN_POINT ( 'NONE',  ( -71.31679049852404262, -48.56916478021601336, 9.992914751153948671 ) ) ;
#15298=CARTESIAN_POINT ( 'NONE',  ( 25.66381174941535903, 2.554701667279945632, -3.769256280910082246 ) ) ;
#15306=CARTESIAN_POINT ( 'NONE',  ( 14.75656734209353438, -5.138193647293536337, -2.500021671374450971 ) ) ;
#15307=CARTESIAN_POINT ( 'NONE',  ( 24.36996980807726487, 1.959928190074600174, -4.382497187266871208 ) ) ;
#15314=ORIENTED_EDGE ( 'NONE', *, *, #11883, .F. ) ;
#15315=CARTESIAN_POINT ( 'NONE',  ( 86.43572624768424362, -0.5192074800720991590, -5.777013305174518720 ) ) ;
#15320=VERTEX_POINT ( 'NONE', #34071 ) ;
#15321=CARTESIAN_POINT ( 'NONE',  ( 22.61561539124943820, 4.625252967631755752, 3.040925913900980770 ) ) ;
#15329=FACE_OUTER_BOUND ( 'NONE', #26810, .T. ) ;
#15330=CARTESIAN_POINT ( 'NONE',  ( -70.92837670882107659, -37.87473357531881391, -6.000000000000002665 ) ) ;
#15331=CARTESIAN_POINT ( 'NONE',  ( 22.49462040199967916, -0.5704057512449431933, -9.208717712401224276 ) ) ;
#15333=CARTESIAN_POINT ( 'NONE',  ( -72.84144643148528075, 2.639073776085810508, 9.875428661471469027 ) ) ;
#15335=CARTESIAN_POINT ( 'NONE',  ( 37.13484346446838202, -3.067129328972788560, 5.985434385025355297 ) ) ;
#15340=CARTESIAN_POINT ( 'NONE',  ( 30.88496348195457486, 0.7017159523777027896, -4.487237605170554033 ) ) ;
#15342=CARTESIAN_POINT ( 'NONE',  ( 14.88745559820020503, 12.58383137495263426, 2.513086349116905538 ) ) ;
#15344=CARTESIAN_POINT ( 'NONE',  ( 29.66982562896108533, -3.795200865155387238, 4.436618837228561318 ) ) ;
#15347=CARTESIAN_POINT ( 'NONE',  ( 17.33042790160538615, 14.30105679307200717, -2.500000000000000000 ) ) ;
#15348=CARTESIAN_POINT ( 'NONE',  ( 26.47073111379101817, 1.156830035182202288, -4.368930852996396830 ) ) ;
#15349=CARTESIAN_POINT ( 'NONE',  ( 36.88979637976984804, -2.115963839364304544, -5.872280461611828706 ) ) ;
#15350=CARTESIAN_POINT ( 'NONE',  ( 24.72423210327035648, 2.636217293557414632, -3.925404993220885430 ) ) ;
#15354=CARTESIAN_POINT ( 'NONE',  ( 34.12043071199392585, -3.462209586952626150, 5.516511185785388349 ) ) ;
#15358=CARTESIAN_POINT ( 'NONE',  ( 87.94592890065770519, -0.6044765299818539717, 4.822713664802365408 ) ) ;
#15359=CARTESIAN_POINT ( 'NONE',  ( 37.05071641422330231, -2.827661766178285685, -5.989058390038934476 ) ) ;
#15361=CARTESIAN_POINT ( 'NONE',  ( 24.70880527336989374, 2.644804217804675339, 3.921322591264182034 ) ) ;
#15364=ORIENTED_EDGE ( 'NONE', *, *, #17140, .T. ) ;
#15380=ADVANCED_FACE ( 'NONE', ( #29436 ), #7582, .T. ) ;
#15381=CARTESIAN_POINT ( 'NONE',  ( 21.71185578408363881, 6.328645931448866335, 3.192210964217056191 ) ) ;
#15382=CARTESIAN_POINT ( 'NONE',  ( 22.44128072547340125, 4.727156261423415273, -3.200930849007907586 ) ) ;
#15384=DIRECTION ( 'NONE',  ( -7.232507224765808510E-18, 1.000000000000000000, 0.000000000000000000 ) ) ;
#15387=CARTESIAN_POINT ( 'NONE',  ( 25.48535437492803624, -4.309695067542732794, -2.926019122942394191 ) ) ;
#15388=CARTESIAN_POINT ( 'NONE',  ( -79.68766234410863092, -5.608549218928701841, -4.839603289619596183 ) ) ;
#15391=CARTESIAN_POINT ( 'NONE',  ( 88.27260010123318068, -2.240648412321151639, -1.886171102315310266 ) ) ;
#15392=CARTESIAN_POINT ( 'NONE',  ( 14.78134360068729336, 12.96929629928027516, 2.499999999999999112 ) ) ;
#15393=VERTEX_POINT ( 'NONE', #22414 ) ;
#15401=CARTESIAN_POINT ( 'NONE',  ( 35.33522214168899467, -3.170233168067363216, 5.721314019424172059 ) ) ;
#15402=CARTESIAN_POINT ( 'NONE',  ( 85.14289959633329374, 2.721178644307868044, -0.4516327360412458747 ) ) ;
#15407=CARTESIAN_POINT ( 'NONE',  ( 17.26328941701764919, -2.999363701367865787, 2.900751846394634459 ) ) ;
#15410=CARTESIAN_POINT ( 'NONE',  ( 27.36782613089871674, -4.434391534612712960, -3.677648743169859902 ) ) ;
#15415=EDGE_LOOP ( 'NONE', ( #18284, #5927, #19344, #39993 ) ) ;
#15416=CARTESIAN_POINT ( 'NONE',  ( 22.04653420616095616, 3.143092986063939165, 4.783053969572811148 ) ) ;
#15417=CARTESIAN_POINT ( 'NONE',  ( 21.56339383302955071, 7.351415377951304286, -2.885032705794761121 ) ) ;
#15421=ADVANCED_FACE ( 'NONE', ( #9839 ), #34373, .F. ) ;
#15424=CARTESIAN_POINT ( 'NONE',  ( -70.42444715658567134, 0.09064798068341432813, 5.980032331837195514 ) ) ;
#15425=DIRECTION ( 'NONE',  ( -1.000000000000000000, -7.232507224765808510E-18, 0.000000000000000000 ) ) ;
#15429=CARTESIAN_POINT ( 'NONE',  ( 22.04016737215521360, 3.514630979057402183, -4.507021302255509454 ) ) ;
#15430=ORIENTED_EDGE ( 'NONE', *, *, #18405, .T. ) ;
#15432=VECTOR ( 'NONE', #17554, 1000.000000000000000 ) ;
#15433=CARTESIAN_POINT ( 'NONE',  ( 21.85643539959776760, 8.340603020592608274, -8.602649199348869402 ) ) ;
#15436=ORIENTED_EDGE ( 'NONE', *, *, #8507, .F. ) ;
#15440=CARTESIAN_POINT ( 'NONE',  ( 87.34576652878352832, 0.2468139514080059382, -4.863684402402743245 ) ) ;
#15445=CARTESIAN_POINT ( 'NONE',  ( 28.88870476122235331, -3.262720734457520422, 4.666716578517512204 ) ) ;
#15446=CARTESIAN_POINT ( 'NONE',  ( 21.53525696227849551, 7.395501062873577780, -0.9772312434468740650 ) ) ;
#15447=CARTESIAN_POINT ( 'NONE',  ( 34.93088199418607331, -1.706447725614655520, -5.658206960402972996 ) ) ;
#15454=CARTESIAN_POINT ( 'NONE',  ( 36.20082885389868466, -3.649409372564311305, 5.718625934384519383 ) ) ;
#15458=CARTESIAN_POINT ( 'NONE',  ( 87.64754863977299237, -2.175244042755086760, -2.906226134380668125 ) ) ;
#15459=AXIS2_PLACEMENT_3D ( 'NONE', #23838, #36413, #2675 ) ;
#15468=CARTESIAN_POINT ( 'NONE',  ( 24.03052928095394591, 3.323090062041115011, 3.304702637807089172 ) ) ;
#15473=ORIENTED_EDGE ( 'NONE', *, *, #38202, .F. ) ;
#15477=CARTESIAN_POINT ( 'NONE',  ( 17.79339514573547376, 8.594434151433056002, -2.958563574914779615 ) ) ;
#15480=ORIENTED_EDGE ( 'NONE', *, *, #11400, .T. ) ;
#15490=CARTESIAN_POINT ( 'NONE',  ( 28.73718198699435433, 0.3327373454474676917, -5.564570571917969666 ) ) ;
#15494=CARTESIAN_POINT ( 'NONE',  ( 26.64541687229243294, 1.018703328949602138, -4.378789651849845477 ) ) ;
#15502=CARTESIAN_POINT ( 'NONE',  ( 37.17267509869564890, -2.956902742721974953, -5.999791034500704612 ) ) ;
#15506=( BOUNDED_SURFACE ( )  B_SPLINE_SURFACE ( 3, 2, ( 
 ( #4649, #1566, #29359 ),
 ( #13712, #14096, #39210 ),
 ( #10998, #14502, #2393 ),
 ( #33266, #40036, #14918 ),
 ( #18000, #1982, #24187 ),
 ( #24595, #14699, #24392 ),
 ( #21522, #36951, #34097 ),
 ( #15122, #30162, #39413 ),
 ( #11608, #5251, #17579 ),
 ( #33679, #5049, #11203 ),
 ( #8528, #36743, #36344 ),
 ( #30585, #30998, #21111 ),
 ( #14299, #27077, #8112 ),
 ( #39622, #23969, #2181 ),
 ( #11809, #11403, #20681 ),
 ( #27268, #8320, #40234 ),
 ( #5459, #27486, #8938 ),
 ( #20894, #33480, #8730 ) ),
 .UNSPECIFIED., .F., .F., .T. ) 
 B_SPLINE_SURFACE_WITH_KNOTS ( ( 4, 2, 2, 2, 2, 2, 2, 2, 4 ),
 ( 3, 3 ),
 ( 0.1120466800099417792, 0.1143735122104352075, 0.1149552202605585716, 0.1151006472730894126, 0.1151733607793548331, 0.1152460742856202536, 0.1155369283106819356, 0.1167003444109286497, 0.1213540088119155202 ),
 ( 0.4204862958135378581, 1.000000000000000000 ),
 .UNSPECIFIED. ) 
 GEOMETRIC_REPRESENTATION_ITEM ( )  RATIONAL_B_SPLINE_SURFACE ( (
 ( 0.9643893222201109783, 0.9576553645928089775, 1.000000000000000000),
 ( 0.9643512025059277626, 0.9576100364637323281, 1.000000000000000000),
 ( 0.9643130339552848929, 0.9575646502632511048, 1.000000000000000000),
 ( 0.9642652639231832357, 0.9575078469469748832, 1.000000000000000000),
 ( 0.9642557069497447175, 0.9574964827556402547, 1.000000000000000000),
 ( 0.9642437570514184042, 0.9574822731387686581, 1.000000000000000000),
 ( 0.9642413668876821387, 0.9574794309965157790, 1.000000000000000000),
 ( 0.9642377813664757547, 0.9574751674554182745, 1.000000000000000000),
 ( 0.9642387421108769008, 0.9574763098760044056, 1.000000000000000000),
 ( 0.9642387421108769008, 0.9574763098760044056, 1.000000000000000000),
 ( 0.9642387421108765677, 0.9574763098760041835, 1.000000000000000000),
 ( 0.9642387421108765677, 0.9574763098760041835, 1.000000000000000000),
 ( 0.9642387421108769008, 0.9574763098760044056, 1.000000000000000000),
 ( 0.9642387421108769008, 0.9574763098760044056, 1.000000000000000000),
 ( 0.9642387421108769008, 0.9574763098760044056, 1.000000000000000000),
 ( 0.9642387421108769008, 0.9574763098760044056, 1.000000000000000000),
 ( 0.9642387421108769008, 0.9574763098760044056, 1.000000000000000000),
 ( 0.9642387421108769008, 0.9574763098760044056, 1.000000000000000000) ) ) 
 REPRESENTATION_ITEM ( '' )  SURFACE ( )  );
#15511=CARTESIAN_POINT ( 'NONE',  ( 87.06807637922989329, 0.009568187950425697044, -5.830412620327568796 ) ) ;
#15525=CARTESIAN_POINT ( 'NONE',  ( 23.43876222436442802, 3.796239004519351923, 3.093510792665742137 ) ) ;
#15527=CARTESIAN_POINT ( 'NONE',  ( 18.65469762088386574, -3.106616286309057617, 3.066837553255504556 ) ) ;
#15532=CARTESIAN_POINT ( 'NONE',  ( 24.67241584745087479, 0.7088272946872185010, 4.794457209858541624 ) ) ;
#15537=CARTESIAN_POINT ( 'NONE',  ( 0.000000000000000000, 0.000000000000000000, 2.500000000000000000 ) ) ;
#15541=CARTESIAN_POINT ( 'NONE',  ( 21.85643539959774628, 5.695295784951009743, -9.764639101464164028 ) ) ;
#15544=CARTESIAN_POINT ( 'NONE',  ( -72.05672345664538625, 4.865640908481359439, 9.936545240694519165 ) ) ;
#15548=CARTESIAN_POINT ( 'NONE',  ( -80.68923699068490407, 10.55697554841911590, -2.212078010654421334 ) ) ;
#15550=CARTESIAN_POINT ( 'NONE',  ( 27.81823897074509233, 1.847144674410869936, -3.899787536903625895 ) ) ;
#15552=CARTESIAN_POINT ( 'NONE',  ( 14.74910353868988899, 12.91027092149337641, 2.503635293877921164 ) ) ;
#15554=LINE ( 'NONE', #5891, #17464 ) ;
#15557=CARTESIAN_POINT ( 'NONE',  ( 26.39112261854958064, 1.214606541396050066, -4.362303127903641276 ) ) ;
#15558=CARTESIAN_POINT ( 'NONE',  ( 30.97689734888565383, -3.765698233401996387, -4.598238574220234298 ) ) ;
#15559=CARTESIAN_POINT ( 'NONE',  ( 25.99837217835952075, 1.969169038965218332, -4.208579848621752717 ) ) ;
#15560=ORIENTED_EDGE ( 'NONE', *, *, #17986, .T. ) ;
#15564=CARTESIAN_POINT ( 'NONE',  ( 21.30795797853340900, 3.457867745315728047, 3.532020196095992493 ) ) ;
#15569=CARTESIAN_POINT ( 'NONE',  ( 85.30740962031771346, 1.871039318281703334, 5.038373847784950676 ) ) ;
#15571=CARTESIAN_POINT ( 'NONE',  ( 35.94856560473117923, -2.120269416292473785, -5.817041100599634973 ) ) ;
#15572=ORIENTED_EDGE ( 'NONE', *, *, #1296, .T. ) ;
#15573=CARTESIAN_POINT ( 'NONE',  ( 25.19497952292325493, 2.388040330658791621, 4.036871176649600379 ) ) ;
#15575=FACE_OUTER_BOUND ( 'NONE', #3421, .T. ) ;
#15578=EDGE_CURVE ( 'NONE', #13284, #4251, #38380, .T. ) ;
#15590=CARTESIAN_POINT ( 'NONE',  ( -71.18984706668749141, -21.75705254805669853, 9.997314914349638926 ) ) ;
#15593=CARTESIAN_POINT ( 'NONE',  ( 23.14704033844979492, 3.979479066984730640, -3.185135796097247063 ) ) ;
#15596=CARTESIAN_POINT ( 'NONE',  ( 25.32326662574907772, -3.445015843796760624, -4.932833089913290614 ) ) ;
#15597=CARTESIAN_POINT ( 'NONE',  ( -77.45835083621990691, -4.875850942340420602, -9.162514641918679814 ) ) ;
#15600=CARTESIAN_POINT ( 'NONE',  ( 86.69339609521894374, -0.1977197225095213562, 5.906572220802119411 ) ) ;
#15604=FACE_OUTER_BOUND ( 'NONE', #18466, .T. ) ;
#15605=EDGE_CURVE ( 'NONE', #37831, #16241, #38745, .T. ) ;
#15610=ORIENTED_EDGE ( 'NONE', *, *, #2071, .F. ) ;
#15611=CARTESIAN_POINT ( 'NONE',  ( 34.33227999214794579, -1.487593080494464592, 5.564780640740604412 ) ) ;
#15613=ORIENTED_EDGE ( 'NONE', *, *, #1468, .F. ) ;
#15624=CARTESIAN_POINT ( 'NONE',  ( 27.35736631516831352, -4.438324952666481416, -3.674147289654650095 ) ) ;
#15629=CARTESIAN_POINT ( 'NONE',  ( 34.93810637183052847, -3.179019197238403205, 5.659334499256591045 ) ) ;
#15631=CARTESIAN_POINT ( 'NONE',  ( 24.00126456572668943, 2.472460351644033771, 4.166039721954374997 ) ) ;
#15632=CARTESIAN_POINT ( 'NONE',  ( 36.10487649157640533, -1.522124056221337396, 5.639071623872836447 ) ) ;
#15638=CARTESIAN_POINT ( 'NONE',  ( 86.25914659815089180, 1.467357031587646743, -4.709363322567870824 ) ) ;
#15643=CARTESIAN_POINT ( 'NONE',  ( 22.41886727961536252, 3.592987785001729328, -4.133826006051191548 ) ) ;
#15644=VERTEX_POINT ( 'NONE', #13131 ) ;
#15646=CARTESIAN_POINT ( 'NONE',  ( 21.85643539959775339, -7.728916438363212293, -14.50668795789714771 ) ) ;
#15648=ORIENTED_EDGE ( 'NONE', *, *, #28970, .F. ) ;
#15652=CARTESIAN_POINT ( 'NONE',  ( 86.82658554816774199, 0.8299826706514633612, -5.353109082705294952 ) ) ;
#15656=CARTESIAN_POINT ( 'NONE',  ( 16.26588554675592491, -3.448400933796594625, 2.730870020955348476 ) ) ;
#15657=CARTESIAN_POINT ( 'NONE',  ( 33.68691125750341087, -3.105118810531902085, -5.464055241398425800 ) ) ;
#15661=ADVANCED_BREP_SHAPE_REPRESENTATION ( '', ( #39057, #30744 ), #7710 ) ;
#15666=CARTESIAN_POINT ( 'NONE',  ( 37.17580397388785229, -2.565365416181118352, 5.981100958229804476 ) ) ;
#15668=CARTESIAN_POINT ( 'NONE',  ( 87.68276862112787740, -2.218184809142153657, -2.724441466588327199 ) ) ;
#15671=ORIENTED_EDGE ( 'NONE', *, *, #38248, .T. ) ;
#15676=ORIENTED_EDGE ( 'NONE', *, *, #24394, .F. ) ;
#15680=CARTESIAN_POINT ( 'NONE',  ( 21.84320321800310438, 5.888203138701116224, 3.167919337418751091 ) ) ;
#15683=VERTEX_POINT ( 'NONE', #2418 ) ;
#15685=CARTESIAN_POINT ( 'NONE',  ( 14.70402854863798048, 12.78588281574406871, -2.501317291925987174 ) ) ;
#15688=CARTESIAN_POINT ( 'NONE',  ( 15.37524305911110289, 11.52859259604422526, -2.577749823976538401 ) ) ;
#15698=CARTESIAN_POINT ( 'NONE',  ( 31.58133870531054654, -3.380569343585269504, 5.164673136779329710 ) ) ;
#15699=PLANE ( 'NONE',  #20111 ) ;
#15700=CARTESIAN_POINT ( 'NONE',  ( 15.71680133604306029, -1.673294295210183247, 2.499999999999999556 ) ) ;
#15702=CARTESIAN_POINT ( 'NONE',  ( 14.77222818450456643, -4.461908109758233820, -2.511961494517393145 ) ) ;
#15708=CARTESIAN_POINT ( 'NONE',  ( 36.07747683933082783, -1.633048991712910736, -5.715736162573779033 ) ) ;
#15717=CARTESIAN_POINT ( 'NONE',  ( 21.88122113745853170, -13.31826209935299232, 2.500000000000000000 ) ) ;
#15732=ORIENTED_EDGE ( 'NONE', *, *, #13990, .T. ) ;
#15733=CARTESIAN_POINT ( 'NONE',  ( 21.82879977636547864, 5.975179493283890864, 3.129347940797799765 ) ) ;
#15739=CARTESIAN_POINT ( 'NONE',  ( 23.60934223726077974, 0.4472814905813886632, 5.505706761109173009 ) ) ;
#15749=DIRECTION ( 'NONE',  ( -1.000000000000000000, -1.165409145176969993E-16, 0.000000000000000000 ) ) ;
#15751=CARTESIAN_POINT ( 'NONE',  ( -75.06536287548681230, 8.003295856082973003, 10.46294883374669027 ) ) ;
#15752=CARTESIAN_POINT ( 'NONE',  ( 37.19747299874393320, -2.841585884120807481, 5.999818732555961098 ) ) ;
#15753=DIRECTION ( 'NONE',  ( 1.000000000000000000, 0.000000000000000000, 0.000000000000000000 ) ) ;
#15754=CARTESIAN_POINT ( 'NONE',  ( -81.25386658927445183, 10.50434922290921413, -3.708380354180676797 ) ) ;
#15756=CARTESIAN_POINT ( 'NONE',  ( 33.46399183110135311, -3.088807006424163948, -5.429263273580746230 ) ) ;
#15757=CARTESIAN_POINT ( 'NONE',  ( 30.88430831131045906, 0.7006950504784862366, -4.489146872953734047 ) ) ;
#15759=CARTESIAN_POINT ( 'NONE',  ( 17.26693970169123560, 8.754007361387712294, 2.901321561600415322 ) ) ;
#15761=CARTESIAN_POINT ( 'NONE',  ( 29.59347476571312185, -3.810682212465021923, 4.411907216274745913 ) ) ;
#15766=CARTESIAN_POINT ( 'NONE',  ( 23.17369588073228925, 0.5344006672354065790, -5.787134729987309711 ) ) ;
#15767=CARTESIAN_POINT ( 'NONE',  ( 31.79454364665378208, -3.762500967924790274, -4.762111375201251384 ) ) ;
#15768=CARTESIAN_POINT ( 'NONE',  ( 25.68847553089295488, 2.131605409771632598, -4.143887395686703279 ) ) ;
#15772=CARTESIAN_POINT ( 'NONE',  ( 36.80687207428664465, -3.101440543725207277, 5.951000583394169041 ) ) ;
#15773=CIRCLE ( 'NONE', #33539, 10.00000000000000533 ) ;
#15774=EDGE_CURVE ( 'NONE', #38743, #17308, #29429, .T. ) ;
#15776=CARTESIAN_POINT ( 'NONE',  ( 84.71993633203089757, 2.603525311087758531, 3.468835001793752593 ) ) ;
#15778=CARTESIAN_POINT ( 'NONE',  ( 22.06574104993566721, 4.215197008693921887, 2.277743168818826991 ) ) ;
#15782=CARTESIAN_POINT ( 'NONE',  ( 26.39040341943793067, 1.756034159389934235, 4.288588000376896581 ) ) ;
#15788=CARTESIAN_POINT ( 'NONE',  ( -17.69482985384421880, -29.56993018339339940, -2.500000000000000000 ) ) ;
#15799=CARTESIAN_POINT ( 'NONE',  ( -70.92837670882238399, -21.78299143689875095, 10.00000000000113154 ) ) ;
#15801=CARTESIAN_POINT ( 'NONE',  ( 22.61627571821124150, 4.610947867309832304, -3.060900723906414100 ) ) ;
#15806=CARTESIAN_POINT ( 'NONE',  ( -79.97971716480111581, -5.605125688071920464, -6.478939869332222656 ) ) ;
#15809=CARTESIAN_POINT ( 'NONE',  ( 84.89189963960113516, 2.021164017676272184, 4.676249375175704159 ) ) ;
#15813=CARTESIAN_POINT ( 'NONE',  ( 21.59025852387176769, 7.197660357961259692, -2.960420257542255129 ) ) ;
#15821=CARTESIAN_POINT ( 'NONE',  ( 35.45270935990075856, -1.916751615000411801, 5.739650741265255540 ) ) ;
#15822=CARTESIAN_POINT ( 'NONE',  ( 88.11777217834651310, -0.6203394357796320202, -3.242821525125987758 ) ) ;
#15826=CARTESIAN_POINT ( 'NONE',  ( 14.66103313215672088, -4.888004096372116969, 2.500000000000000000 ) ) ;
#15831=CARTESIAN_POINT ( 'NONE',  ( -78.05373003007660770, -6.395912128405124797, 7.028357164679021274 ) ) ;
#15836=CARTESIAN_POINT ( 'NONE',  ( 22.27216333610519072, 1.991400367839498475, 5.539784122813447453 ) ) ;
#15837=CARTESIAN_POINT ( 'NONE',  ( 21.58863023475808873, 7.202558683720228672, -2.923977588977705544 ) ) ;
#15840=DIRECTION ( 'NONE',  ( 8.398074759113475787E-17, -1.000000000000000000, 0.000000000000000000 ) ) ;
#15842=CARTESIAN_POINT ( 'NONE',  ( 85.59084391823684257, 2.218026321225774478, -3.342052983375342734 ) ) ;
#15846=CARTESIAN_POINT ( 'NONE',  ( 22.38852551694001036, 3.992526559945270392, -3.863756592174965920 ) ) ;
#15848=CARTESIAN_POINT ( 'NONE',  ( 21.85643539959774273, 11.61750052538138256, -3.706567411524428479 ) ) ;
#15853=CARTESIAN_POINT ( 'NONE',  ( 87.54465900634191655, 0.02340848060778613626, -4.593250482506632260 ) ) ;
#15858=CARTESIAN_POINT ( 'NONE',  ( 14.71571335596265229, -5.054827965358537512, 2.496165019355487846 ) ) ;
#15859=EDGE_CURVE ( 'NONE', #38743, #31898, #21560, .T. ) ;
#15860=CARTESIAN_POINT ( 'NONE',  ( 22.92029997850032075, 2.650801711463111499, -3.783665159831076874 ) ) ;
#15875=CARTESIAN_POINT ( 'NONE',  ( 87.74107704030866728, -0.1972175777057878776, -3.821749651402456482 ) ) ;
#15883=ADVANCED_FACE ( 'NONE', ( #27307 ), #3298, .T. ) ;
#15886=ORIENTED_EDGE ( 'NONE', *, *, #5070, .F. ) ;
#15890=CARTESIAN_POINT ( 'NONE',  ( 15.50095926939750512, 11.04212219595600430, -2.625697604742827984 ) ) ;
#15899=CARTESIAN_POINT ( 'NONE',  ( 16.81957507921353212, 9.797913115272733009, 2.499999999999583000 ) ) ;
#15900=CARTESIAN_POINT ( 'NONE',  ( 31.28551011801044268, -2.837290201336624129, -5.599793116354693012 ) ) ;
#15910=CARTESIAN_POINT ( 'NONE',  ( -62.92837670882106238, 0.7293679304675899644, -6.000000000000000000 ) ) ;
#15911=CARTESIAN_POINT ( 'NONE',  ( 35.81800206278433052, -3.623520638983628750, -5.691500669916689681 ) ) ;
#15914=CARTESIAN_POINT ( 'NONE',  ( 14.81690770463735696, -6.144096738234146926, -2.518934814212393292 ) ) ;
#15921=ORIENTED_EDGE ( 'NONE', *, *, #15997, .F. ) ;
#15924=CARTESIAN_POINT ( 'NONE',  ( 22.81051389511380378, 3.483508258214782494, 3.928497976265352687 ) ) ;
#15929=CARTESIAN_POINT ( 'NONE',  ( 23.75025100005262146, 3.569496731975624115, 3.159471240185062424 ) ) ;
#15934=CARTESIAN_POINT ( 'NONE',  ( 27.36415855513426010, 1.088262529702572090, 4.476529622290722266 ) ) ;
#15939=EDGE_CURVE ( 'NONE', #29684, #9599, #17158, .T. ) ;
#15944=CARTESIAN_POINT ( 'NONE',  ( 22.32365817596653557, 5.835156701882857178, 3.488260158266504263 ) ) ;
#15947=CARTESIAN_POINT ( 'NONE',  ( -72.95894646306267362, 3.821331306903040126, 10.95076600805725597 ) ) ;
#15948=CARTESIAN_POINT ( 'NONE',  ( 23.58291088458457452, 0.3979808540708968390, -5.534409494045887890 ) ) ;
#15954=CARTESIAN_POINT ( 'NONE',  ( -80.96011311534428501, 11.45103779093585139, -0.1896456026672926065 ) ) ;
#15955=CARTESIAN_POINT ( 'NONE',  ( 32.88854752500713374, -3.408127832021003112, -5.320408019716786896 ) ) ;
#15956=CARTESIAN_POINT ( 'NONE',  ( 29.48946025503517987, 1.221228239622528911, -4.218580362071199019 ) ) ;
#15958=LINE ( 'NONE', #938, #19627 ) ;
#15965=CARTESIAN_POINT ( 'NONE',  ( 24.90850614488217474, 1.271311299353267366, -4.572860818722448428 ) ) ;
#15966=CARTESIAN_POINT ( 'NONE',  ( 30.12331966194739508, -3.814067162060288396, -4.420979061340549521 ) ) ;
#15970=LINE ( 'NONE', #18439, #33243 ) ;
#15971=CARTESIAN_POINT ( 'NONE',  ( 85.98972789526511917, 0.6168376674493800671, -5.987237289632960646 ) ) ;
#15972=ORIENTED_EDGE ( 'NONE', *, *, #2122, .T. ) ;
#15973=CARTESIAN_POINT ( 'NONE',  ( 24.62487772016506327, 2.984843784653229193, 3.535646819143488884 ) ) ;
#15994=CARTESIAN_POINT ( 'NONE',  ( 23.42789715074077606, 3.768348859778905435, -3.162797842696227324 ) ) ;
#15995=VERTEX_POINT ( 'NONE', #3096 ) ;
#15997=EDGE_CURVE ( 'NONE', #21048, #24927, #38616, .T. ) ;
#15998=VERTEX_POINT ( 'NONE', #21801 ) ;
#16004=EDGE_CURVE ( 'NONE', #6415, #36097, #9019, .T. ) ;
#16005=CARTESIAN_POINT ( 'NONE',  ( -79.68099787142058688, -6.645740692013860418, -4.853373096521103491 ) ) ;
#16009=CARTESIAN_POINT ( 'NONE',  ( 86.92455237868826146, -1.249784692553891574, -5.093375875629621241 ) ) ;
#16010=DIRECTION ( 'NONE',  ( 0.000000000000000000, 0.000000000000000000, 1.000000000000000000 ) ) ;
#16013=CARTESIAN_POINT ( 'NONE',  ( 21.58875153664575919, 7.202486658336689551, 2.923638573957438869 ) ) ;
#16019=CARTESIAN_POINT ( 'NONE',  ( 29.09974842620354707, 0.3540232340485665596, 4.748117540621001886 ) ) ;
#16020=CARTESIAN_POINT ( 'NONE',  ( 86.42578330747443260, 1.280182770620154953, -5.202446006352976937 ) ) ;
#16033=CARTESIAN_POINT ( 'NONE',  ( 21.71185578408363881, 6.328645931448866335, 3.192210964217056191 ) ) ;
#16034=CARTESIAN_POINT ( 'NONE',  ( 22.81665940757572031, 1.447765978769897766, 5.493635244331218637 ) ) ;
#16046=CARTESIAN_POINT ( 'NONE',  ( 22.40063203884636067, 3.836966881894201098, -3.968227663424939600 ) ) ;
#16049=CARTESIAN_POINT ( 'NONE',  ( 21.85643539959779247, -11.31796667593991401, 0.7532527802845886411 ) ) ;
#16051=ADVANCED_FACE ( 'NONE', ( #20977 ), #33819, .T. ) ;
#16054=CARTESIAN_POINT ( 'NONE',  ( 84.92887162652053235, 2.911150016110632510, -2.020846097872043501 ) ) ;
#16056=CARTESIAN_POINT ( 'NONE',  ( -81.77906269993763999, -5.605534135063645174, 1.073826742008731294 ) ) ;
#16058=CARTESIAN_POINT ( 'NONE',  ( 19.69623932494216945, -2.759629735801022665, 3.280472520642130352 ) ) ;
#16061=CARTESIAN_POINT ( 'NONE',  ( 36.64613206243796384, -2.461592254012722414, -5.925913217033152769 ) ) ;
#16063=CARTESIAN_POINT ( 'NONE',  ( 21.79065355195778153, 5.486589654648796888, 3.529560796445746274 ) ) ;
#16069=CARTESIAN_POINT ( 'NONE',  ( 30.68859365574981624, -3.022523058033317778, 4.996095265064695923 ) ) ;
#16072=CARTESIAN_POINT ( 'NONE',  ( 25.73193413792037987, 2.635028621324468467, 3.526313263793730446 ) ) ;
#16084=VERTEX_POINT ( 'NONE', #37135 ) ;
#16086=EDGE_CURVE ( 'NONE', #19840, #22023, #11390, .T. ) ;
#16088=AXIS2_PLACEMENT_3D ( 'NONE', #29726, #937, #20451 ) ;
#16089=CIRCLE ( 'NONE', #29260, 9.386006772603931125 ) ;
#16093=CARTESIAN_POINT ( 'NONE',  ( -71.31920275879095072, -45.66549222223517290, 5.988038532114558166 ) ) ;
#16095=CARTESIAN_POINT ( 'NONE',  ( 19.02761876096537463, 7.101601804412763563, -3.176118110984106568 ) ) ;
#16101=DIRECTION ( 'NONE',  ( 1.000000000000000000, 0.000000000000000000, 0.000000000000000000 ) ) ;
#16107=CARTESIAN_POINT ( 'NONE',  ( 30.07020345058763766, -4.232275913155626235, -2.900971327107725983 ) ) ;
#16112=LINE ( 'NONE', #22713, #17685 ) ;
#16113=CARTESIAN_POINT ( 'NONE',  ( 33.43921609458320177, -3.587388448609353020, -5.336552248008303856 ) ) ;
#16114=CARTESIAN_POINT ( 'NONE',  ( 32.91483545724720017, -0.5485586877609884837, -5.320376416278755904 ) ) ;
#16120=CIRCLE ( 'NONE', #15459, 6.000000000000002665 ) ;
#16121=CARTESIAN_POINT ( 'NONE',  ( 22.22081959608184931, -10.19411496085875157, 2.499999999999999556 ) ) ;
#16122=AXIS2_PLACEMENT_3D ( 'NONE', #20127, #16827, #20516 ) ;
#16123=DIRECTION ( 'NONE',  ( -0.000000000000000000, -0.000000000000000000, -1.000000000000000000 ) ) ;
#16131=CARTESIAN_POINT ( 'NONE',  ( 30.88699261567396093, -3.468694606085327425, 4.911399322420932911 ) ) ;
#16132=CARTESIAN_POINT ( 'NONE',  ( 22.78168706071813077, 3.725697157195321019, 3.755607005719465263 ) ) ;
#16145=CARTESIAN_POINT ( 'NONE',  ( 22.64667696449940237, 0.3053113478315905849, 6.452936397408012503 ) ) ;
#16152=CARTESIAN_POINT ( 'NONE',  ( 22.79131883835711037, -5.922936844141047708, 5.170149038749508819 ) ) ;
#16155=CARTESIAN_POINT ( 'NONE',  ( -74.32232877538925209, 7.099204298189413009, 10.69770487804055215 ) ) ;
#16156=CARTESIAN_POINT ( 'NONE',  ( 23.04471710095623038, 0.3232145568372689626, -5.972274008649366195 ) ) ;
#16161=CARTESIAN_POINT ( 'NONE',  ( 28.41783740563939631, -4.024351259184133944, -4.165758313493220122 ) ) ;
#16162=CARTESIAN_POINT ( 'NONE',  ( 36.44474408801026755, -1.733425704062592221, -5.731406469632323031 ) ) ;
#16164=CARTESIAN_POINT ( 'NONE',  ( 16.22309343533386539, 10.39346123325232085, 2.693864712708880393 ) ) ;
#16166=DIRECTION ( 'NONE',  ( 0.000000000000000000, 0.000000000000000000, 1.000000000000000000 ) ) ;
#16169=CARTESIAN_POINT ( 'NONE',  ( 34.59489306780999129, -0.7688126975909262972, -5.270100711184057651 ) ) ;
#16176=CARTESIAN_POINT ( 'NONE',  ( 84.35358620389857265, 3.041238144818853684, 1.123552906098365112 ) ) ;
#16180=CARTESIAN_POINT ( 'NONE',  ( 24.86489394813727216, 2.560632942376066534, 3.960803519163274444 ) ) ;
#16182=VECTOR ( 'NONE', #36109, 1000.000000000000114 ) ;
#16186=ORIENTED_EDGE ( 'NONE', *, *, #10627, .F. ) ;
#16188=ORIENTED_EDGE ( 'NONE', *, *, #38248, .F. ) ;
#16199=CARTESIAN_POINT ( 'NONE',  ( 21.85643539959774273, 11.82890447862143546, -1.931159885854170311 ) ) ;
#16200=CARTESIAN_POINT ( 'NONE',  ( 23.42914634548708364, 3.774006297069265159, -3.150363682666455389 ) ) ;
#16206=DIRECTION ( 'NONE',  ( 1.000000000000000000, 7.232507224765808510E-18, 0.000000000000000000 ) ) ;
#16209=CARTESIAN_POINT ( 'NONE',  ( 21.63116867190874260, 6.951708668987069295, -2.990534277344490732 ) ) ;
#16211=CARTESIAN_POINT ( 'NONE',  ( 25.01091298175674993, 3.329590532569525418, 1.936828115940083084 ) ) ;
#16218=CYLINDRICAL_SURFACE ( 'NONE', #38496, 21.28220113893567245 ) ;
#16220=CARTESIAN_POINT ( 'NONE',  ( 36.42101398311888261, -3.115835042429591972, 5.890778096254243756 ) ) ;
#16221=CARTESIAN_POINT ( 'NONE',  ( 86.07545474579461597, 1.673688438695506431, -4.651254279175787154 ) ) ;
#16224=CARTESIAN_POINT ( 'NONE',  ( 21.74105249613594992, 4.237279478211291028, 2.792868651270881131 ) ) ;
#16227=ORIENTED_EDGE ( 'NONE', *, *, #22931, .T. ) ;
#16231=CARTESIAN_POINT ( 'NONE',  ( -79.77824834640263418, -6.648693431677500598, 4.674947531023576630 ) ) ;
#16238=CARTESIAN_POINT ( 'NONE',  ( 22.35184836610467229, 4.907951308887271935, 3.033114723143640390 ) ) ;
#16240=CARTESIAN_POINT ( 'NONE',  ( 24.81935351061392936, 2.321748820690546111, 4.088153248315227195 ) ) ;
#16241=VERTEX_POINT ( 'NONE', #31586 ) ;
#16249=CARTESIAN_POINT ( 'NONE',  ( 23.88318583406893936, 3.159564200708308235, -3.647954507178626127 ) ) ;
#16251=VERTEX_POINT ( 'NONE', #99 ) ;
#16252=CARTESIAN_POINT ( 'NONE',  ( 21.85643539959774273, -8.640774161329524361, 8.772446831725494221 ) ) ;
#16253=CARTESIAN_POINT ( 'NONE',  ( 21.87751110071505778, 4.134169920263886411, 2.121951800777925445 ) ) ;
#16257=CARTESIAN_POINT ( 'NONE',  ( 14.72830186850272938, 12.61371249416686702, 2.505105730543339515 ) ) ;
#16258=CARTESIAN_POINT ( 'NONE',  ( 16.21738897043104899, -3.323621905045633262, 2.737513786506908353 ) ) ;
#16259=CARTESIAN_POINT ( 'NONE',  ( 36.76006098925728338, -2.519186585992552185, 5.943694581444969316 ) ) ;
#16260=CARTESIAN_POINT ( 'NONE',  ( 33.25546742218144658, -3.823472235995165835, 5.051159332570485105 ) ) ;
#16261=CARTESIAN_POINT ( 'NONE',  ( 36.44714645434917344, -2.354196673243254434, -5.894856700406053029 ) ) ;
#16264=VECTOR ( 'NONE', #34646, 1000.000000000000000 ) ;
#16269=CARTESIAN_POINT ( 'NONE',  ( 28.79959244091942594, -3.877818713555981400, 4.349622696032581004 ) ) ;
#16272=CARTESIAN_POINT ( 'NONE',  ( 33.45666195923615049, -3.831709260703673792, 5.091247116679021190 ) ) ;
#16278=CARTESIAN_POINT ( 'NONE',  ( -61.24591834330252027, 3.729367930467589076, 2.500000000000000000 ) ) ;
#16280=EDGE_LOOP ( 'NONE', ( #26381, #35167 ) ) ;
#16284=CARTESIAN_POINT ( 'NONE',  ( 23.71002378246611997, 3.505939628316281809, 3.324835373315420561 ) ) ;
#16288=VERTEX_POINT ( 'NONE', #3411 ) ;
#16293=CARTESIAN_POINT ( 'NONE',  ( 14.83458786958485121, 12.32104755890018843, -2.521694231548856191 ) ) ;
#16296=ORIENTED_EDGE ( 'NONE', *, *, #9414, .T. ) ;
#16297=ORIENTED_EDGE ( 'NONE', *, *, #29780, .F. ) ;
#16298=CARTESIAN_POINT ( 'NONE',  ( 14.61802081865033820, 0.000000000000000000, 2.500000000000000000 ) ) ;
#16300=LINE ( 'NONE', #38317, #38108 ) ;
#16303=FACE_OUTER_BOUND ( 'NONE', #4954, .T. ) ;
#16304=CARTESIAN_POINT ( 'NONE',  ( 30.11529565287584020, -4.511537616843412479, 1.859944388213511157 ) ) ;
#16307=CARTESIAN_POINT ( 'NONE',  ( -70.31378976201078501, -21.58254907604969119, 9.981524770340065800 ) ) ;
#16312=CARTESIAN_POINT ( 'NONE',  ( 31.93469105406368413, 0.01670955582175310053, -5.060964027022966327 ) ) ;
#16320=CIRCLE ( 'NONE', #1889, 15.73502530973474478 ) ;
#16325=CARTESIAN_POINT ( 'NONE',  ( 22.59185701846717365, 3.735489254463754349, 3.886158523879209348 ) ) ;
#16329=CARTESIAN_POINT ( 'NONE',  ( 22.18602618867068443, 5.272228373216523600, 3.073292335441606848 ) ) ;
#16332=AXIS2_PLACEMENT_3D ( 'NONE', #29868, #14012, #11312 ) ;
#16338=CARTESIAN_POINT ( 'NONE',  ( 21.79343922618468810, 0.2295100222190576966, 8.344713507481587911 ) ) ;
#16342=EDGE_LOOP ( 'NONE', ( #8486, #17243, #14759, #11085 ) ) ;
#16347=CARTESIAN_POINT ( 'NONE',  ( 25.22633673370294360, -3.172752697882940343, -5.351597462314125586 ) ) ;
#16350=VERTEX_POINT ( 'NONE', #16712 ) ;
#16351=CARTESIAN_POINT ( 'NONE',  ( -74.87498290905593024, -4.683714315110599102, 9.194508750764200045 ) ) ;
#16352=CARTESIAN_POINT ( 'NONE',  ( 21.73387437812568734, 0.2123458951770110792, -9.115319698840053775 ) ) ;
#16353=ORIENTED_EDGE ( 'NONE', *, *, #3110, .T. ) ;
#16356=CARTESIAN_POINT ( 'NONE',  ( 28.33577056900993085, -3.844698498189621283, -4.468379450010504961 ) ) ;
#16357=CARTESIAN_POINT ( 'NONE',  ( 37.21170653579515175, -2.744006139658493826, -6.000908227333882294 ) ) ;
#16359=CARTESIAN_POINT ( 'NONE',  ( 16.06488434713086022, 10.27331943285140703, 2.713711751702661434 ) ) ;
#16367=CARTESIAN_POINT ( 'NONE',  ( 25.86636253853731304, 2.039549717436321963, -4.181506972325073512 ) ) ;
#16368=CARTESIAN_POINT ( 'NONE',  ( 28.98805360192195835, 1.403918898879884747, -4.132826440151677438 ) ) ;
#16373=CARTESIAN_POINT ( 'NONE',  ( 88.23373314635465192, -2.194529332924425091, 2.156499936145213070 ) ) ;
#16375=ORIENTED_EDGE ( 'NONE', *, *, #13335, .F. ) ;
#16376=CARTESIAN_POINT ( 'NONE',  ( -78.43906097479739969, 10.12407436886776857, -8.325837142764415333 ) ) ;
#16383=ORIENTED_EDGE ( 'NONE', *, *, #3818, .F. ) ;
#16388=ORIENTED_EDGE ( 'NONE', *, *, #1551, .F. ) ;
#16394=CARTESIAN_POINT ( 'NONE',  ( 21.85643539959774984, 10.28856666709980594, -7.862822601098399034 ) ) ;
#16395=CARTESIAN_POINT ( 'NONE',  ( 22.39111293279836090, 4.899164074087773990, -3.083163210143192057 ) ) ;
#16401=CARTESIAN_POINT ( 'NONE',  ( -73.27260478087752915, -2.820680093043031356, -9.724700656314139380 ) ) ;
#16405=CARTESIAN_POINT ( 'NONE',  ( 84.23599009083828548, 2.852497016463987567, -2.111805961397795084 ) ) ;
#16408=CARTESIAN_POINT ( 'NONE',  ( 21.53535333134909635, 7.395104665118339859, -0.5014549742099433383 ) ) ;
#16409=CARTESIAN_POINT ( 'NONE',  ( 33.33044624270629441, -1.121386909979642077, 5.408420254699600527 ) ) ;
#16418=CARTESIAN_POINT ( 'NONE',  ( 37.04599030669736237, -2.800861170604020511, 5.988320766658103089 ) ) ;
#16420=CARTESIAN_POINT ( 'NONE',  ( 88.48259847388298738, -1.030129646626848361, 1.133857545573457415 ) ) ;
#16427=CARTESIAN_POINT ( 'NONE',  ( 24.55255634016017297, -6.099742195186348859, -2.771823335699560964 ) ) ;
#16429=CARTESIAN_POINT ( 'NONE',  ( -73.43598941707226402, -3.052414302668824853, 9.681195182795574894 ) ) ;
#16433=CARTESIAN_POINT ( 'NONE',  ( -61.24591834330252027, -23.80776546975053520, 2.500000000000000000 ) ) ;
#16434=CARTESIAN_POINT ( 'NONE',  ( 22.25885516624144600, 1.430813568335262964, 6.081876650313324362 ) ) ;
#16440=CARTESIAN_POINT ( 'NONE',  ( 85.30059172038076554, 2.544051366058079466, 2.076667998869941911 ) ) ;
#16441=CARTESIAN_POINT ( 'NONE',  ( -8.295002936191391285, 28.24537450226321411, -2.500000000000000000 ) ) ;
#16442=B_SPLINE_SURFACE_WITH_KNOTS ( 'NONE', 5, 3, ( 
 ( #14996, #36618, #39490, #30448, #33352, #5331, #7997, #1645, #11890, #8804, #36417, #40111, #4920, #14183, #20553, #26753, #30040, #8189, #20761, #8402, #39293, #11485, #33556, #5128, #23651, #24259, #1855, #5531, #17866, #14377, #36822, #30243, #2058, #11279 ),
 ( #18075, #17661, #27145, #30664, #27555, #39697, #30870, #5944, #9420, #34583, #34987, #40718, #22417, #18279, #9017, #2678, #18482, #37225, #27959, #6150, #185, #15821, #21597, #27754, #2879, #18691, #40307, #3496, #16019, #12518, #25092, #15198, #394, #12932 ),
 ( #3299, #31069, #34788, #28376, #15401, #34177, #9637, #12723, #12313, #37621, #40502, #25297, #24888, #12097, #6565, #25494, #22008, #37425, #24674, #34377, #6360, #38042, #31274, #15611, #31476, #9221, #31678, #9842, #28163, #21800, #18907, #3094, #37832, #22218 ),
 ( #19111, #28584, #22619, #38642, #10636, #26110, #10439, #10037, #10833, #26503, #35585, #32295, #7554, #16418, #23213, #7159, #39034, #32099, #38841, #35389, #20109, #999, #28991, #7356, #10240, #23017, #25694, #23409, #29585, #13932, #792, #17010, #35187, #19314 ),
 ( #19914, #6960, #16605, #6762, #1401, #19721, #16811, #16220, #31886, #29391, #3697, #13322, #32689, #19519, #28789, #596, #4093, #38434, #3903, #4488, #32485, #38237, #13136, #1210, #13535, #29189, #25899, #22820, #4284, #13744, #26308, #35778, #40062, #11843 ),
 ( #17211, #8348, #7756, #39238, #21138, #33508, #1596, #27099, #20710, #7953, #36568, #17610, #30187, #36370, #20303, #32889, #4868, #33704, #5484, #2008, #14528, #30616, #27511, #14126, #4676, #5279, #27298, #20924, #20501, #11635, #30402, #33083, #11027, #39864 ),
 ( #39649, #17402, #2207, #29985, #29778, #24212, #18027, #11433, #1801, #26704, #11229, #23997, #2425, #8141, #33296, #36773, #14326, #14945, #26895, #5079, #39438, #23796, #27910, #16517, #30822, #18856, #25047, #6103, #9588, #31225, #37579, #29093, #15564, #12674 ),
 ( #895, #12476, #9177, #25250, #34129, #144, #24836, #24421, #8963, #15772, #12264, #37781, #18639, #5898, #9375, #40453, #40672, #2628, #36977, #6519, #31630, #18436, #34741, #27707, #21341, #15148, #33913, #40261, #31025, #2832, #3044, #5692, #28120, #21961 ),
 ( #6307, #18233, #15354, #22170, #12045, #24624, #37177, #21749, #37384, #21552, #19066, #34534, #34332, #31429, #3253, #28328, #23314, #26008, #1110, #4586, #29685, #30102, #35884, #17508, #13431, #4189, #38539, #13640, #32396, #23117, #1305, #36084, #10938, #16706 ),
 ( #26213, #14031, #7662, #29296, #1498, #13842, #26411, #35686, #7257, #20213, #17309, #7861, #26806, #38744, #19821, #10346, #10539, #38940, #7459, #14234, #4980, #20014, #39142, #32990, #4774, #35486, #26605, #22918, #32596, #39344, #23517, #4394, #17114, #10734 ),
 ( #16916, #11136, #23707, #32796, #20411, #8048, #29496, #29886, #1703, #36273, #20606, #33193, #30297, #18331, #40165, #2111, #5183, #34023, #27608, #36669, #36878, #27202, #37072, #11535, #18538, #30923, #24730, #21235, #8453, #11333, #17924, #33809, #37282, #2313 ),
 ( #23898, #15253, #9073, #39965, #1911, #5588, #5384, #21650, #8246, #8862, #2523, #24314, #27806, #8658, #15048, #34229, #18128, #2730, #6001, #14432, #30720, #11946, #24522, #21448, #5794, #40360, #24106, #21036, #27003, #12156, #39549, #36469, #20816, #33412 ),
 ( #17715, #14627, #39758, #33610, #30507, #14836, #27403, #11736, #2938, #21851, #28014, #6206, #25140, #9473, #25346, #38292, #12775, #37885, #34636, #7011, #12987, #25754, #35040, #19166, #34427, #34840, #13188, #37672, #35241, #10094, #16072, #22678, #28638, #234 ),
 ( #22272, #6818, #9694, #6615, #18749, #31123, #15454, #31732, #28427, #31940, #43, #19372, #31527, #40561, #15666, #22472, #18961, #3747, #3546, #12572, #443, #6410, #25551, #9273, #12373, #24943, #37476, #22062, #652, #31325, #28212, #3352, #38092, #9895 ),
 ( #16272, #28844, #19966, #29641, #29045, #26759, #1453, #39299, #1057, #20363, #35441, #3954, #13381, #16866, #10491, #22871, #32942, #38897, #38491, #16473, #13985, #13796, #29448, #32155, #7211, #10691, #35837, #36224, #1260, #23658, #19579, #10293, #850, #19775 ),
 ( #32350, #4730, #17063, #25959, #23271, #4343, #4145, #20164, #26364, #7611, #32545, #16659, #29246, #13590, #26164, #1653, #14188, #38694, #32750, #23073, #17264, #35640, #4542, #7410, #26558, #39094, #29838, #11086, #10890, #23465, #36033, #7812, #8003, #4925 ),
 ( #14578, #17458, #24054, #39915, #30877, #8409, #5337, #21189, #30045, #18081, #1860, #40313, #30669, #39497, #11689, #2683, #2063, #12102, #15206, #33760, #27759, #5540, #17871, #33561, #23847, #24267, #11896, #27356, #36829, #11284, #24680, #20559, #8611, #30455 ),
 ( #40118, #2262, #17666, #27151, #33143, #33971, #2478, #15001, #5744, #24469, #36423, #14382, #27561, #37026, #26951, #8194, #8810, #39704, #20765, #21396, #18286, #33359, #5133, #30248, #14787, #11491, #36623, #20982, #6570, #5948, #3703, #19116, #16224, #18697 ) ),
 .UNSPECIFIED., .F., .F., .F.,
 ( 6, 5, 2, 5, 6 ),
 ( 4, 1, 1, 1, 1, 1, 1, 1, 1, 1, 1, 1, 1, 1, 1, 1, 1, 1, 1, 1, 1, 1, 1, 1, 1, 1, 1, 1, 1, 1, 1, 4 ),
 ( -0.01000000000000000021, 0.000000000000000000, 0.5000000000000000000, 1.000000000000000000, 1.010000000000000009 ),
 ( 0.000000000000000000, 0.0006830822270650580572, 0.001366164454130116114, 0.001935399643350998100, 0.002390787794727703471, 0.002732328908260232229, 0.003016946502870673438, 0.003244640578559025799, 0.003386949375864246187, 0.003500796413708422584, 0.003586181692091554990, 0.003671566970474687830, 0.003756952248857819369, 0.003842337527240952209, 0.003956184565085128606, 0.004098493362390348560, 0.004269263919156613372, 0.004496957994844966167, 0.004781575589455406942, 0.005123116702987936567, 0.005578504854364642156, 0.006147740043585522840, 0.006830822270650581222, 0.007513904497715638738, 0.008424680800469050782, 0.009563151178910813885, 0.01092931563304092892, 0.01229548008717104568, 0.01411703269267786803, 0.01639397344956139424, 0.01912630235782162777, 0.02185863126608186130 ),
 .UNSPECIFIED. ) ;
#16445=CARTESIAN_POINT ( 'NONE',  ( 24.34601857225426613, 2.911169162268197663, -3.762662789421892029 ) ) ;
#16449=CARTESIAN_POINT ( 'NONE',  ( 21.85643539959777826, -9.955546997263933662, -6.545918539092090427 ) ) ;
#16452=CARTESIAN_POINT ( 'NONE',  ( 21.85643539958836357, 4.448544635526659796, 2.117591927225508375 ) ) ;
#16455=CARTESIAN_POINT ( 'NONE',  ( 88.42327724305060599, -1.151963697325209202, 3.685007885677881401 ) ) ;
#16460=CARTESIAN_POINT ( 'NONE',  ( 35.96749414751118223, -2.128554350996951339, 5.819995357488987331 ) ) ;
#16463=CARTESIAN_POINT ( 'NONE',  ( 36.19435599471948706, -2.231546916727529695, -5.855402635420312585 ) ) ;
#16465=CARTESIAN_POINT ( 'NONE',  ( 84.35969326541092528, 2.698637575869491378, 2.857603098124533947 ) ) ;
#16470=CARTESIAN_POINT ( 'NONE',  ( 30.68920804271916936, -3.119417099748506672, 4.996191155010656360 ) ) ;
#16473=CARTESIAN_POINT ( 'NONE',  ( 36.44468416319452331, -1.733384222877294878, 5.731389134260409080 ) ) ;
#16480=FACE_OUTER_BOUND ( 'NONE', #24223, .T. ) ;
#16484=CARTESIAN_POINT ( 'NONE',  ( 24.61641440591999341, 2.982913459046241833, 3.546506353475846307 ) ) ;
#16495=CARTESIAN_POINT ( 'NONE',  ( 22.36662521325363429, 4.219501547067421754, -3.697250822039899187 ) ) ;
#16498=CARTESIAN_POINT ( 'NONE',  ( 28.70293208761703241, -1.592347763559425200, -5.966126087555218227 ) ) ;
#16507=EDGE_CURVE ( 'NONE', #10538, #1864, #29302, .T. ) ;
#16508=CARTESIAN_POINT ( 'NONE',  ( 35.10421778843286944, -1.272554766392203440, -5.608957993449237733 ) ) ;
#16514=CARTESIAN_POINT ( 'NONE',  ( 14.77222812468899349, 12.33286846116284252, -2.511961485181726239 ) ) ;
#16517=CARTESIAN_POINT ( 'NONE',  ( 34.36128308910517859, -1.406858267515045169, 5.569307275463330598 ) ) ;
#16523=DIRECTION ( 'NONE',  ( -7.232507224765808510E-18, 1.000000000000000000, 0.000000000000000000 ) ) ;
#16524=CARTESIAN_POINT ( 'NONE',  ( 23.02262922662109546, 3.378767241194165383, 3.887974689243142823 ) ) ;
#16529=CARTESIAN_POINT ( 'NONE',  ( 23.14201580508249734, 4.050829872694250433, 3.071595331972348131 ) ) ;
#16536=CARTESIAN_POINT ( 'NONE',  ( 25.39364064017554767, 0.7063433326595477402, 4.600238427421414755 ) ) ;
#16537=CARTESIAN_POINT ( 'NONE',  ( 14.61802060715431750, -4.492938368545131844, -2.500000000000015987 ) ) ;
#16544=CARTESIAN_POINT ( 'NONE',  ( 22.46150523612397976, 0.3089437977474873143, 9.145744397224946809 ) ) ;
#16546=ORIENTED_EDGE ( 'NONE', *, *, #1562, .T. ) ;
#16547=CARTESIAN_POINT ( 'NONE',  ( -75.80815061396138788, -5.389879833924653418, 8.736367909994982028 ) ) ;
#16548=CARTESIAN_POINT ( 'NONE',  ( 24.12050462314963895, 0.4787749110952863596, -5.098002984902643142 ) ) ;
#16553=CARTESIAN_POINT ( 'NONE',  ( 21.73904017688714063, 4.235523729101259072, -2.801162699060028238 ) ) ;
#16555=CARTESIAN_POINT ( 'NONE',  ( 19.02452760875551618, 7.104206974277733622, 3.175635661921960118 ) ) ;
#16560=CARTESIAN_POINT ( 'NONE',  ( 31.70551703006545097, 0.3859655886019467408, -4.660405379804645420 ) ) ;
#16561=CARTESIAN_POINT ( 'NONE',  ( -62.92837670882106238, -39.37473357531882101, -6.000000000000000000 ) ) ;
#16565=CARTESIAN_POINT ( 'NONE',  ( 21.71182896267971074, 6.328908860361642574, -3.192117583127509928 ) ) ;
#16566=CARTESIAN_POINT ( 'NONE',  ( 84.75081314860828741, 2.206698042984908792, -4.319373971756642838 ) ) ;
#16570=CARTESIAN_POINT ( 'NONE',  ( -80.84835038658981432, 10.51112849907171132, -4.793973201337777823 ) ) ;
#16571=EDGE_CURVE ( 'NONE', #37970, #11084, #36884, .T. ) ;
#16579=DIRECTION ( 'NONE',  ( -1.000000000000000000, 0.000000000000000000, 0.000000000000000000 ) ) ;
#16586=CARTESIAN_POINT ( 'NONE',  ( 21.85643539959774273, -7.673977846683588844, 14.52234238348545681 ) ) ;
#16592=CARTESIAN_POINT ( 'NONE',  ( -72.46938654171589178, -1.268490862809277919, -9.881656514212606268 ) ) ;
#16594=CYLINDRICAL_SURFACE ( 'NONE', #14898, 7.744449365083023729 ) ;
#16595=DIRECTION ( 'NONE',  ( 0.000000000000000000, 0.000000000000000000, 1.000000000000000000 ) ) ;
#16597=CARTESIAN_POINT ( 'NONE',  ( 84.10013685850573495, 3.017793503712738357, 0.3246723698904760980 ) ) ;
#16602=CARTESIAN_POINT ( 'NONE',  ( 20.58577122809306204, 5.855186692365746737, -3.419305487539204158 ) ) ;
#16605=CARTESIAN_POINT ( 'NONE',  ( 34.13616914347945652, -3.136032219204479610, 5.534172799846977853 ) ) ;
#16608=CARTESIAN_POINT ( 'NONE',  ( 86.64693249831780975, 1.031777503091004800, -5.158387491453222395 ) ) ;
#16616=CARTESIAN_POINT ( 'NONE',  ( -80.91065676098010329, -6.597313057213482601, -0.5950503846463383040 ) ) ;
#16618=B_SPLINE_CURVE_WITH_KNOTS ( 'NONE', 5,
 ( #39301, #23075, #13987, #29644, #39097, #7814, #20365, #32945 ),
 .UNSPECIFIED., .F., .F.,
 ( 6, 2, 6 ),
 ( 0.000000000000000000, 0.5000000000000000000, 1.000000000000000000 ),
 .UNSPECIFIED. ) ;
#16623=ADVANCED_FACE ( 'NONE', ( #36279 ), #20613, .F. ) ;
#16624=CARTESIAN_POINT ( 'NONE',  ( 26.09009134676806241, 1.922323258887854269, 4.227532586804973569 ) ) ;
#16627=ADVANCED_FACE ( 'NONE', ( #26813 ), #11339, .T. ) ;
#16630=CARTESIAN_POINT ( 'NONE',  ( 14.73664178711198147, 12.61985148690504133, -2.505541970458011747 ) ) ;
#16634=CARTESIAN_POINT ( 'NONE',  ( 22.81500972751208067, 3.448192808966587197, -3.952749550737099327 ) ) ;
#16636=CARTESIAN_POINT ( 'NONE',  ( -71.72734076235239797, -0.1676685021849017854, 5.947290612307118529 ) ) ;
#16638=CARTESIAN_POINT ( 'NONE',  ( 21.85643539959777826, -5.315239383820637542, 13.63683724657638052 ) ) ;
#16639=CARTESIAN_POINT ( 'NONE',  ( 19.99661396372949440, 11.93735323785185543, 1.251290237290588149E-12 ) ) ;
#16642=CARTESIAN_POINT ( 'NONE',  ( 86.36811837411410409, 0.9377611381114191458, -5.884791073222536362 ) ) ;
#16646=CARTESIAN_POINT ( 'NONE',  ( 33.94823428658630604, -3.200574468876375533, 5.504841020207380531 ) ) ;
#16647=CARTESIAN_POINT ( 'NONE',  ( 31.54670663170724865, -3.759141947944208084, 4.713116287240913138 ) ) ;
#16648=CARTESIAN_POINT ( 'NONE',  ( 14.67364265041105753, -5.606975079573447651, -2.496574837622112408 ) ) ;
#16649=CARTESIAN_POINT ( 'NONE',  ( 36.97956974538411146, -2.956624624668434009, -5.977954231677896857 ) ) ;
#16651=CARTESIAN_POINT ( 'NONE',  ( -74.96765694090700549, -3.041086699640438429, 10.49870045681198683 ) ) ;
#16652=CARTESIAN_POINT ( 'NONE',  ( -4.890026461918812295, -8.951974136083761024, -2.500000000000000000 ) ) ;
#16656=CARTESIAN_POINT ( 'NONE',  ( 33.44795012684379287, -3.712436240568119494, 5.220878576662950188 ) ) ;
#16657=ORIENTED_EDGE ( 'NONE', *, *, #20915, .T. ) ;
#16659=CARTESIAN_POINT ( 'NONE',  ( 37.10451636438106249, -3.126525554563963194, 5.976203789056629745 ) ) ;
#16670=FACE_OUTER_BOUND ( 'NONE', #30516, .T. ) ;
#16680=CARTESIAN_POINT ( 'NONE',  ( 21.49033551098300165, 5.616517115020018380, -3.514817270055297094 ) ) ;
#16690=CARTESIAN_POINT ( 'NONE',  ( 26.56136967304951213, 3.021295450130037530, 0.006841891102512360698 ) ) ;
#16692=CARTESIAN_POINT ( 'NONE',  ( -70.92837670882238399, -21.78299143689875095, 10.00000000000113154 ) ) ;
#16694=LINE ( 'NONE', #19611, #1820 ) ;
#16697=CARTESIAN_POINT ( 'NONE',  ( 35.04487071626047623, -1.406682813658225673, -5.661182748920821517 ) ) ;
#16706=CARTESIAN_POINT ( 'NONE',  ( 20.66011059366096703, 4.228419983037499996, 3.378133128719581268 ) ) ;
#16712=CARTESIAN_POINT ( 'NONE',  ( -61.24591834330252027, -42.37473357531882812, -2.500000000000000000 ) ) ;
#16714=CARTESIAN_POINT ( 'NONE',  ( 23.22017056567068494, 3.363622401179964250, 3.779250300422446696 ) ) ;
#16720=CARTESIAN_POINT ( 'NONE',  ( 22.87850294736509582, 4.337130434239091947, 3.058172268432443275 ) ) ;
#16726=ORIENTED_EDGE ( 'NONE', *, *, #29784, .T. ) ;
#16728=CARTESIAN_POINT ( 'NONE',  ( 21.98532980874193399, 0.2335280526894900899, 7.692103986081960443 ) ) ;
#16734=LINE ( 'NONE', #10160, #1738 ) ;
#16739=CARTESIAN_POINT ( 'NONE',  ( 22.80834877297060004, -6.429644848144123515, 3.896382617761176892 ) ) ;
#16742=CARTESIAN_POINT ( 'NONE',  ( -81.10044192579809419, -5.650254496098106038, 4.158657536701277913 ) ) ;
#16746=B_SPLINE_CURVE_WITH_KNOTS ( 'NONE', 3,
 ( #18683, #31268, #9835, #6951 ),
 .UNSPECIFIED., .F., .F.,
 ( 4, 4 ),
 ( 8.335636658244670956E-05, 0.008874052763743587799 ),
 .UNSPECIFIED. ) ;
#16749=CARTESIAN_POINT ( 'NONE',  ( 33.45650472609418102, -3.831704090213303715, -5.091214335412847625 ) ) ;
#16750=CARTESIAN_POINT ( 'NONE',  ( 30.71467839345701023, -3.288362829192787107, -4.965898286879354195 ) ) ;
#16765=CARTESIAN_POINT ( 'NONE',  ( 84.25787434187677150, 2.991901652185509075, -1.300773176381055940 ) ) ;
#16768=CARTESIAN_POINT ( 'NONE',  ( -81.82309097574839996, 10.46037581310753772, 0.2594491973369116300 ) ) ;
#16770=CARTESIAN_POINT ( 'NONE',  ( -83.92837670882109080, 2.429809908903242999, 12.50000000000000000 ) ) ;
#16774=CARTESIAN_POINT ( 'NONE',  ( -70.92837670882107659, -23.80776546975053520, 10.00000000000000888 ) ) ;
#16778=ORIENTED_EDGE ( 'NONE', *, *, #29344, .T. ) ;
#16783=CARTESIAN_POINT ( 'NONE',  ( 26.91783537306902119, 1.348898915238470497, 4.407577238912754325 ) ) ;
#16786=CARTESIAN_POINT ( 'NONE',  ( 21.85643539959776760, 9.535790418011023561, -9.299971273199719946 ) ) ;
#16787=DIRECTION ( 'NONE',  ( -0.000000000000000000, 0.000000000000000000, 1.000000000000000000 ) ) ;
#16788=VERTEX_POINT ( 'NONE', #40169 ) ;
#16792=CARTESIAN_POINT ( 'NONE',  ( -74.17935931525508408, -3.991321171111944732, -9.458026139773300756 ) ) ;
#16799=B_SPLINE_CURVE_WITH_KNOTS ( 'NONE', 3,
 ( #27244, #33653, #27453, #8703, #24362, #21746, #24620, #37380, #40059, #37776, #3250, #28325, #15144, #31425, #21134, #33701, #12259, #15559, #36974, #27703, #40256, #15768, #21549, #31221, #30613, #140, #3041, #12671, #2625, #21956, #8754, #5480, #14942, #15350, #9372, #18023, #30819, #40450, #11838, #2419, #28116, #18636, #21338, #2829, #24833, #33910, #34530, #25246, #5688, #6099, #40669, #12473, #27508, #34329, #24417, #18230, #6303, #25042, #12042, #9174, #5895, #34125, #37174, #18852, #18433, #8959, #31021, #27906, #37576 ),
 .UNSPECIFIED., .F., .F.,
 ( 4, 2, 2, 1, 1, 1, 1, 1, 2, 2, 2, 1, 1, 1, 1, 1, 2, 2, 2, 2, 1, 1, 1, 1, 1, 2, 2, 1, 2, 2, 1, 1, 2, 1, 2, 2, 2, 1, 2, 2, 2, 1, 2, 2, 4 ),
 ( 0.000000000000000000, 0.1250000000000453804, 0.1875000000000680567, 0.2187500000000786871, 0.2343750000000833222, 0.2421875000000850153, 0.2460937500000858480, 0.2480468750000862643, 0.2490234375000858480, 0.2500000000000854317, 0.3750000000001176281, 0.4375000000001337264, 0.4687500000001417755, 0.4843750000001458278, 0.4921875000001487144, 0.4960937500001492695, 0.4980468750001496581, 0.5000000000001499911, 0.6250000000002199352, 0.6875000000002549072, 0.7187500000002723377, 0.7343750000002787770, 0.7421875000002816636, 0.7460937500002862155, 0.7480468750002851053, 0.7490234375002847722, 0.7500000000002845502, 0.7812500000002576828, 0.7968750000002441380, 0.8007812500002396972, 0.8046875000002351452, 0.8125000000002252643, 0.8437500000001855183, 0.8593750000001656453, 0.8671875000001554312, 0.8750000000001451061, 0.8906250000001246780, 0.8984375000001154632, 0.9023437500001109113, 0.9062500000001062483, 0.9218750000000908162, 0.9296875000000820455, 0.9335937500000766054, 0.9375000000000711653, 1.000000000000000000 ),
 .UNSPECIFIED. ) ;
#16801=CARTESIAN_POINT ( 'NONE',  ( 33.61621798268036798, -1.223546897810831480, 5.453021846138203621 ) ) ;
#16811=CARTESIAN_POINT ( 'NONE',  ( 36.14170422902504498, -3.144485308923159028, 5.847185053995919368 ) ) ;
#16815=CARTESIAN_POINT ( 'NONE',  ( 87.43361094620441065, 0.1481429324132612357, -5.028924837761966415 ) ) ;
#16820=ORIENTED_EDGE ( 'NONE', *, *, #5875, .F. ) ;
#16822=CARTESIAN_POINT ( 'NONE',  ( 23.06591706423118637, -8.086835649431872497, -2.500000000000005773 ) ) ;
#16825=ADVANCED_FACE ( 'NONE', ( #30510, #11140 ), #14841, .T. ) ;
#16827=DIRECTION ( 'NONE',  ( 0.000000000000000000, -0.000000000000000000, -1.000000000000000000 ) ) ;
#16829=CARTESIAN_POINT ( 'NONE',  ( 22.09304849718642316, 0.3726161401571594922, 7.354740019033460641 ) ) ;
#16833=CARTESIAN_POINT ( 'NONE',  ( 85.42670333274200800, 2.402396817435708876, 2.739882088504116631 ) ) ;
#16838=CARTESIAN_POINT ( 'NONE',  ( 21.96956884823482881, 4.963862418377736674, -3.595920138844930669 ) ) ;
#16842=EDGE_CURVE ( 'NONE', #23233, #17714, #37825, .T. ) ;
#16843=CARTESIAN_POINT ( 'NONE',  ( 21.85643539959778536, -8.233350057040109249, -11.92691213149646678 ) ) ;
#16844=CARTESIAN_POINT ( 'NONE',  ( 21.86257038566819588, 3.862145465818127121, -3.386728275810359623 ) ) ;
#16847=CARTESIAN_POINT ( 'NONE',  ( 85.85116863490735284, 1.861966474136578231, -4.950709030323501736 ) ) ;
#16849=ORIENTED_EDGE ( 'NONE', *, *, #8027, .T. ) ;
#16850=CARTESIAN_POINT ( 'NONE',  ( -78.42754742544201463, -5.260774960203544737, 8.337059064591437973 ) ) ;
#16852=CARTESIAN_POINT ( 'NONE',  ( 14.82083291377484358, -6.154340523497400461, 2.519547438029839270 ) ) ;
#16853=CARTESIAN_POINT ( 'NONE',  ( 32.63305097123843979, -3.795354871036205058, 4.923932146436776236 ) ) ;
#16854=CARTESIAN_POINT ( 'NONE',  ( 14.64249155491722831, -5.613241577028397877, -2.491712955778045746 ) ) ;
#16855=CARTESIAN_POINT ( 'NONE',  ( 34.13628169468366735, -3.131472990218530317, -5.534190366183364240 ) ) ;
#16861=EDGE_CURVE ( 'NONE', #21048, #18658, #23710, .T. ) ;
#16866=CARTESIAN_POINT ( 'NONE',  ( 37.21169332916825567, -2.743835684017817744, 6.000896651629099132 ) ) ;
#16871=CARTESIAN_POINT ( 'NONE',  ( 86.88453911838293209, -1.192694612346317573, 5.156246139204053947 ) ) ;
#16872=AXIS2_PLACEMENT_3D ( 'NONE', #13123, #25682, #10022 ) ;
#16877=CARTESIAN_POINT ( 'NONE',  ( 1.700390093233090871, -29.56993018339339940, -6.000000000000000000 ) ) ;
#16881=CARTESIAN_POINT ( 'NONE',  ( 14.66962918947518979, -4.461995682952458964, -2.500000000000003553 ) ) ;
#16888=CARTESIAN_POINT ( 'NONE',  ( 22.72845964424274001, 2.421760147549044895, -4.797409384227349527 ) ) ;
#16897=CARTESIAN_POINT ( 'NONE',  ( 30.37020714367901775, -0.1410433206546675144, -5.583699017444894608 ) ) ;
#16908=CARTESIAN_POINT ( 'NONE',  ( 31.78482901221541823, -0.3652494130366964464, -5.167189304987498844 ) ) ;
#16915=ORIENTED_EDGE ( 'NONE', *, *, #4349, .T. ) ;
#16916=CARTESIAN_POINT ( 'NONE',  ( 33.44586992423308658, -3.711826566333543909, 5.220901829495124602 ) ) ;
#16923=CARTESIAN_POINT ( 'NONE',  ( 85.65342632314096250, 0.8846110238782115553, -5.852385830138683076 ) ) ;
#16931=CARTESIAN_POINT ( 'NONE',  ( 22.38745053706796284, 4.913031730865500712, 3.072246906157164670 ) ) ;
#16933=CARTESIAN_POINT ( 'NONE',  ( 17.95234582529949563, -3.169824730388413947, 2.966045911591449702 ) ) ;
#16938=CARTESIAN_POINT ( 'NONE',  ( 21.73454763666067890, 0.2393990557980432143, 9.044420270734587319 ) ) ;
#16946=CIRCLE ( 'NONE', #7754, 12.38600677260393113 ) ;
#16947=CARTESIAN_POINT ( 'NONE',  ( 28.10206848396558499, 1.736549293047330300, -3.980455106513370200 ) ) ;
#16949=ORIENTED_EDGE ( 'NONE', *, *, #10112, .T. ) ;
#16950=CARTESIAN_POINT ( 'NONE',  ( -73.25244780539486555, -2.789250568390547080, 9.729507352929793740 ) ) ;
#16951=CARTESIAN_POINT ( 'NONE',  ( 24.74342160786476086, 0.5916730990911962529, -4.777714225875230980 ) ) ;
#16953=DIRECTION ( 'NONE',  ( -1.000000000000000000, 0.000000000000000000, 0.000000000000000000 ) ) ;
#16955=CARTESIAN_POINT ( 'NONE',  ( 24.57142899942570224, 3.461735479277903149, 1.987691357384508528 ) ) ;
#16956=EDGE_CURVE ( 'NONE', #39349, #10538, #14129, .T. ) ;
#16957=VERTEX_POINT ( 'NONE', #27205 ) ;
#16958=CARTESIAN_POINT ( 'NONE',  ( 36.44525044284685578, -1.732523961244382571, -5.730839696777302983 ) ) ;
#16963=CARTESIAN_POINT ( 'NONE',  ( 30.15929301752064973, -3.700805759990258181, 4.595697454274616511 ) ) ;
#16973=CARTESIAN_POINT ( 'NONE',  ( 84.21365554304541945, 2.879787869890822360, 1.939519519617897592 ) ) ;
#16983=CARTESIAN_POINT ( 'NONE',  ( 37.13838689045984154, -2.480252515904725730, 5.965224451857021215 ) ) ;
#16990=CARTESIAN_POINT ( 'NONE',  ( -5.316495087772345585, -32.84709638682603838, 2.500000000000000000 ) ) ;
#16994=CARTESIAN_POINT ( 'NONE',  ( -72.89992789846300525, 1.434322839394358784, -10.95649126954176467 ) ) ;
#17005=CARTESIAN_POINT ( 'NONE',  ( 17.27255596930787362, 8.732200699463135152, -2.902198115991937222 ) ) ;
#17010=CARTESIAN_POINT ( 'NONE',  ( 22.92029331350176946, 2.650804407416140318, 3.783664119596848785 ) ) ;
#17012=CARTESIAN_POINT ( 'NONE',  ( 88.57583237253618336, -1.134854386742023546, -1.768762308819206375 ) ) ;
#17024=ORIENTED_EDGE ( 'NONE', *, *, #8449, .F. ) ;
#17028=CARTESIAN_POINT ( 'NONE',  ( 23.58901020575210694, 0.9355507091876290593, 5.296862904573749198 ) ) ;
#17031=CARTESIAN_POINT ( 'NONE',  ( 59.69572451838116933, -0.8894979772356270686, 5.999999999999999112 ) ) ;
#17034=CARTESIAN_POINT ( 'NONE',  ( 23.42116204356915432, 3.682620607390830969, -3.312496470421961714 ) ) ;
#17035=ORIENTED_EDGE ( 'NONE', *, *, #36241, .F. ) ;
#17038=CARTESIAN_POINT ( 'NONE',  ( 22.71767909661236118, -4.608197067329504293, -7.212190040765698917 ) ) ;
#17039=CARTESIAN_POINT ( 'NONE',  ( 18.05491602130007678, 13.75800355181789847, -1.937621434240431872 ) ) ;
#17044=CARTESIAN_POINT ( 'NONE',  ( 88.66616934308579800, -1.912773240965560673, 2.173515562489431563 ) ) ;
#17049=CARTESIAN_POINT ( 'NONE',  ( 18.23781241676677567, -2.821824372035762529, 3.052849729433298354 ) ) ;
#17052=CARTESIAN_POINT ( 'NONE',  ( 14.76670373698843441, -5.963909898562598677, -2.511099270873083267 ) ) ;
#17054=CARTESIAN_POINT ( 'NONE',  ( 33.62697853900108669, -1.233820033134908067, -5.454701291197152635 ) ) ;
#17057=CARTESIAN_POINT ( 'NONE',  ( 29.67732598669241639, -3.794111227251059315, -4.438748131648309503 ) ) ;
#17059=CARTESIAN_POINT ( 'NONE',  ( -70.92837670882107659, -37.87473357531881391, 10.00000000000000888 ) ) ;
#17061=EDGE_LOOP ( 'NONE', ( #39945, #18098, #40518, #709 ) ) ;
#17063=CARTESIAN_POINT ( 'NONE',  ( 34.14243320110696089, -3.848523200534588184, 5.234472016327581301 ) ) ;
#17066=CARTESIAN_POINT ( 'NONE',  ( 87.44460083197550659, -1.924926740212006049, 3.742195158538892397 ) ) ;
#17071=ORIENTED_EDGE ( 'NONE', *, *, #8507, .T. ) ;
#17075=DIRECTION ( 'NONE',  ( 0.000000000000000000, -0.000000000000000000, -1.000000000000000000 ) ) ;
#17077=CARTESIAN_POINT ( 'NONE',  ( 23.65048145441440042, 3.304400666319548652, 3.618209137605786552 ) ) ;
#17088=CARTESIAN_POINT ( 'NONE',  ( 22.26524600916998153, 2.472677414347903113, -5.130491956431036726 ) ) ;
#17089=LINE ( 'NONE', #29662, #27024 ) ;
#17092=DIRECTION ( 'NONE',  ( -1.000000000000000000, 0.000000000000000000, 0.000000000000000000 ) ) ;
#17096=CARTESIAN_POINT ( 'NONE',  ( 85.63852691662546590, 2.164466514264067332, 3.769402685279828358 ) ) ;
#17097=CARTESIAN_POINT ( 'NONE',  ( 33.80908501075300165, -4.930824710404003497, 3.361253013157701197 ) ) ;
#17100=CARTESIAN_POINT ( 'NONE',  ( -76.89654088401167087, -4.574922981678376743, -9.546023619539889538 ) ) ;
#17106=CARTESIAN_POINT ( 'NONE',  ( 35.89366792997662969, -2.027922232554310700, -5.808472990748899001 ) ) ;
#17114=CARTESIAN_POINT ( 'NONE',  ( 21.58554998001892855, 4.069564031488925870, 3.350827065184835085 ) ) ;
#17117=EDGE_CURVE ( 'NONE', #21802, #8630, #35265, .T. ) ;
#17121=CARTESIAN_POINT ( 'NONE',  ( 86.29622000419868755, -0.2868749532368798372, -5.899445999458320600 ) ) ;
#17127=CARTESIAN_POINT ( 'NONE',  ( 22.61751675538066664, 4.606962110408180600, 3.064415097794543463 ) ) ;
#17130=CARTESIAN_POINT ( 'NONE',  ( 21.32955647224502371, -0.9288166341206904875, -4.803821987765101831 ) ) ;
#17134=CARTESIAN_POINT ( 'NONE',  ( 22.61765175499198222, 0.2967575410182891060, 6.491500821813259492 ) ) ;
#17135=CARTESIAN_POINT ( 'NONE',  ( 14.69558624142723247, -4.492723223190125736, -2.499999999998670841 ) ) ;
#17136=EDGE_CURVE ( 'NONE', #25549, #833, #23426, .T. ) ;
#17140=EDGE_CURVE ( 'NONE', #5954, #40651, #37153, .T. ) ;
#17142=CIRCLE ( 'NONE', #22439, 15.73502530973474478 ) ;
#17144=CARTESIAN_POINT ( 'NONE',  ( 91.69672933337632514, -4.640393979863029372, -6.000000000000000888 ) ) ;
#17145=CARTESIAN_POINT ( 'NONE',  ( 23.92064240948634790, 4.179079982057642972, -0.5982227118658990372 ) ) ;
#17148=CARTESIAN_POINT ( 'NONE',  ( -79.00905634357600604, -6.586509439605085170, 5.904778360221698108 ) ) ;
#17149=CARTESIAN_POINT ( 'NONE',  ( 26.73391117787527449, 0.9274956043777666803, -4.382155566154702697 ) ) ;
#17150=CARTESIAN_POINT ( 'NONE',  ( -62.92837670882106238, 3.729367930467589076, 6.000000000000000000 ) ) ;
#17153=CARTESIAN_POINT ( 'NONE',  ( 20.91779001269123484, 4.579617817846264316, -2.660979186370516114 ) ) ;
#17158=B_SPLINE_CURVE_WITH_KNOTS ( 'NONE', 3,
 ( #14378, #38894, #11082, #30245, #1450, #11487, #2060, #33140, #24050, #4922, #17261, #32939, #35834, #39296, #11280 ),
 .UNSPECIFIED., .F., .F.,
 ( 4, 1, 1, 1, 1, 1, 1, 1, 2, 2, 4 ),
 ( 0.000000000000000000, 0.2499999999992528754, 0.3749999999988793409, 0.4374999999986877164, 0.4687499999985918486, 0.4843749999985348387, 0.4921874999985063615, 0.4960937499984923171, 0.4980468749984970911, 0.4999999999985018651, 1.000000000000000000 ),
 .UNSPECIFIED. ) ;
#17163=ORIENTED_EDGE ( 'NONE', *, *, #10112, .F. ) ;
#17169=CARTESIAN_POINT ( 'NONE',  ( 85.86655237490620607, 0.5075193453549979861, -5.999391133436077439 ) ) ;
#17170=AXIS2_PLACEMENT_3D ( 'NONE', #38915, #10707, #20185 ) ;
#17175=EDGE_CURVE ( 'NONE', #22380, #17583, #14146, .T. ) ;
#17182=CARTESIAN_POINT ( 'NONE',  ( 37.16547997189702812, -2.549274111243842622, 5.977208762129640363 ) ) ;
#17185=B_SPLINE_CURVE_WITH_KNOTS ( 'NONE', 3,
 ( #12146, #28005, #9064, #34220 ),
 .UNSPECIFIED., .F., .F.,
 ( 4, 4 ),
 ( 0.000000000000000000, 1.000000000000000000 ),
 .UNSPECIFIED. ) ;
#17188=CARTESIAN_POINT ( 'NONE',  ( 16.43915176107237031, 10.14349373407899790, -2.724152508961429575 ) ) ;
#17189=CARTESIAN_POINT ( 'NONE',  ( 17.71472783233827641, 13.97198263493282688, 2.499999999999999556 ) ) ;
#17190=CARTESIAN_POINT ( 'NONE',  ( 21.85643539959775694, 2.022457263371903569, 13.81434276849105558 ) ) ;
#17195=CARTESIAN_POINT ( 'NONE',  ( 14.74825476816264391, -5.104108582077598655, 2.500092996181281890 ) ) ;
#17197=CARTESIAN_POINT ( 'NONE',  ( -73.13538128175785857, 0.2574294580082270301, -10.93005075941053938 ) ) ;
#17201=CARTESIAN_POINT ( 'NONE',  ( -71.92837670882107659, -0.7829914368874778541, 5.916079783099617906 ) ) ;
#17205=CARTESIAN_POINT ( 'NONE',  ( 31.28402977554648601, -0.4023986077216939461, 5.089027472230029048 ) ) ;
#17211=CARTESIAN_POINT ( 'NONE',  ( 33.46244823565493220, -3.089030447167950832, 5.429022358179501850 ) ) ;
#17213=CARTESIAN_POINT ( 'NONE',  ( 87.20660408302002509, 0.2574974038930863407, -5.635807106906071340 ) ) ;
#17221=VERTEX_POINT ( 'NONE', #19927 ) ;
#17227=CARTESIAN_POINT ( 'NONE',  ( 22.77570511409684073, 0.4895864838293038646, 6.218135402904170661 ) ) ;
#17228=CARTESIAN_POINT ( 'NONE',  ( -69.92837670882107659, -0.7829914368874778541, 5.916079783099612577 ) ) ;
#17234=CARTESIAN_POINT ( 'NONE',  ( 63.05383694556373797, -7.271989087314214117, -6.000000000000000000 ) ) ;
#17236=LINE ( 'NONE', #38868, #36289 ) ;
#17238=CARTESIAN_POINT ( 'NONE',  ( 22.14579855485407123, 4.734495042501529305, -3.551530763287582548 ) ) ;
#17240=CARTESIAN_POINT ( 'NONE',  ( -71.54306152300276267, 0.01646366005082695524, 5.969151678864089483 ) ) ;
#17241=CARTESIAN_POINT ( 'NONE',  ( 22.40835304001176098, 2.012838380346585243, -8.570566085397546274 ) ) ;
#17242=CARTESIAN_POINT ( 'NONE',  ( 16.70600419673038672, 9.848044529300576500, 2.500000000000113687 ) ) ;
#17243=ORIENTED_EDGE ( 'NONE', *, *, #39305, .T. ) ;
#17246=CARTESIAN_POINT ( 'NONE',  ( 85.17963886742116131, 2.035184340541872139, -4.783483324554544502 ) ) ;
#17248=ORIENTED_EDGE ( 'NONE', *, *, #24489, .F. ) ;
#17252=CARTESIAN_POINT ( 'NONE',  ( 17.00616749447241105, -3.062907964995312593, -2.860621751864253159 ) ) ;
#17253=CARTESIAN_POINT ( 'NONE',  ( 21.25348834460957193, 3.320962670253897908, -3.523518892371187761 ) ) ;
#17254=DIRECTION ( 'NONE',  ( 1.000000000000000000, -8.959828616340678715E-16, 0.000000000000000000 ) ) ;
#17256=CARTESIAN_POINT ( 'NONE',  ( 29.77376427528636782, -3.774992202640799377, -4.469883408169392780 ) ) ;
#17261=CARTESIAN_POINT ( 'NONE',  ( 31.82986595668942797, -2.965385599430104158, -5.174218409395310303 ) ) ;
#17264=CARTESIAN_POINT ( 'NONE',  ( 36.13284885545721181, -1.530137503075135186, 5.642985908650910432 ) ) ;
#17267=CARTESIAN_POINT ( 'NONE',  ( 87.45314133599802631, -1.935575868345978057, 3.712183661284619962 ) ) ;
#17275=CARTESIAN_POINT ( 'NONE',  ( 22.33423834887513237, 4.544082872025895448, 3.505951737637754029 ) ) ;
#17277=CARTESIAN_POINT ( 'NONE',  ( 14.77222818450456643, -4.461908109758233820, -2.511961494517393145 ) ) ;
#17278=EDGE_CURVE ( 'NONE', #6636, #10306, #11651, .T. ) ;
#17282=CARTESIAN_POINT ( 'NONE',  ( 16.23110856389288514, -3.299995616322477954, -2.739655060876247106 ) ) ;
#17286=CARTESIAN_POINT ( 'NONE',  ( 23.31884880910575220, 2.914054986383341816, -4.090107105141986388 ) ) ;
#17293=CARTESIAN_POINT ( 'NONE',  ( 88.13490256179494509, -0.6395810955261213016, -2.488665338685403849 ) ) ;
#17294=CARTESIAN_POINT ( 'NONE',  ( 32.32438508616473882, -2.203219671913323019, -5.968588774572396893 ) ) ;
#17296=CARTESIAN_POINT ( 'NONE',  ( -71.85035947768736264, -45.91779912024241384, 9.958377439660317521 ) ) ;
#17297=CARTESIAN_POINT ( 'NONE',  ( -73.32814786518467542, -0.3430638954784143158, -10.90362257782414446 ) ) ;
#17299=AXIS2_PLACEMENT_3D ( 'NONE', #541, #32036, #32240 ) ;
#17302=CARTESIAN_POINT ( 'NONE',  ( 27.48830597204979398, 1.193411793497110018, -4.496612972767297656 ) ) ;
#17308=VERTEX_POINT ( 'NONE', #30633 ) ;
#17309=CARTESIAN_POINT ( 'NONE',  ( 36.96305683104023387, -3.150446582698992248, 5.966424068676240644 ) ) ;
#17314=ORIENTED_EDGE ( 'NONE', *, *, #24676, .F. ) ;
#17322=CARTESIAN_POINT ( 'NONE',  ( 23.74696602062051554, 3.565733413989425671, 3.171546063783087455 ) ) ;
#17323=CARTESIAN_POINT ( 'NONE',  ( -71.92837670882107659, -0.7829914368874778541, 9.949874371066204759 ) ) ;
#17330=CARTESIAN_POINT ( 'NONE',  ( 21.97535319280600064, 0.2262477332863455926, 7.720624099575212895 ) ) ;
#17331=CARTESIAN_POINT ( 'NONE',  ( 14.76033746053277262, -5.150563244451003442, -2.500007713060570236 ) ) ;
#17335=CARTESIAN_POINT ( 'NONE',  ( 36.28802971627182217, -3.619218337158335075, -5.742874455817792878 ) ) ;
#17338=CARTESIAN_POINT ( 'NONE',  ( 28.36395155556995817, 1.046816072451675517, -4.961098188302698553 ) ) ;
#17340=ORIENTED_EDGE ( 'NONE', *, *, #33850, .T. ) ;
#17341=CARTESIAN_POINT ( 'NONE',  ( 85.57577930415899914, 1.015208198401525541, 5.782835925834406865 ) ) ;
#17342=CARTESIAN_POINT ( 'NONE',  ( 21.78506910207827829, 0.2162159629002408934, -8.389536844142153171 ) ) ;
#17344=CARTESIAN_POINT ( 'NONE',  ( 13.52694889643372278, 17.29870644234688370, -2.500000000000000000 ) ) ;
#17345=ORIENTED_EDGE ( 'NONE', *, *, #2031, .T. ) ;
#17347=CARTESIAN_POINT ( 'NONE',  ( 35.36129965878185999, -3.735671557810035015, -5.554315758203441256 ) ) ;
#17362=EDGE_CURVE ( 'NONE', #10579, #16251, #29292, .T. ) ;
#17365=CARTESIAN_POINT ( 'NONE',  ( 87.68748590470411841, -1.878626560869070872, 3.708385665356400906 ) ) ;
#17369=FACE_OUTER_BOUND ( 'NONE', #16280, .T. ) ;
#17370=CARTESIAN_POINT ( 'NONE',  ( 23.76457672120657705, 3.581884546121536061, 3.114801549680321191 ) ) ;
#17373=VERTEX_POINT ( 'NONE', #21568 ) ;
#17375=FACE_OUTER_BOUND ( 'NONE', #4317, .T. ) ;
#17379=CIRCLE ( 'NONE', #6256, 6.000000000000002665 ) ;
#17380=PLANE ( 'NONE',  #3120 ) ;
#17384=CARTESIAN_POINT ( 'NONE',  ( 21.85643539959775694, 0.6980322203039187601, 15.81276153107902616 ) ) ;
#17387=CARTESIAN_POINT ( 'NONE',  ( 14.67710233104394923, -4.950387941734374131, 2.499999999999891198 ) ) ;
#17388=CARTESIAN_POINT ( 'NONE',  ( -76.77055093545936870, 10.78502741370083662, -8.125255635421307687 ) ) ;
#17396=CARTESIAN_POINT ( 'NONE',  ( -70.42482556194003962, 0.09084953194484755856, 9.988048282181825499 ) ) ;
#17402=CARTESIAN_POINT ( 'NONE',  ( 33.68138841437632180, -3.186010531076846508, 5.463193268119806767 ) ) ;
#17407=CARTESIAN_POINT ( 'NONE',  ( 85.61973765214487742, 2.185571507920985646, -3.964146163151171187 ) ) ;
#17419=CARTESIAN_POINT ( 'NONE',  ( 23.18011674250855236, 1.027085359276848298, 5.502131735125781908 ) ) ;
#17428=CARTESIAN_POINT ( 'NONE',  ( 21.77142106763977125, 5.727955254944006924, -3.425362973661377985 ) ) ;
#17433=CARTESIAN_POINT ( 'NONE',  ( 22.80834877297060004, -6.429644848144123515, 3.896382617761176892 ) ) ;
#17437=CARTESIAN_POINT ( 'NONE',  ( 84.61987491094994596, 3.070148169510762415, -1.277140785624046426 ) ) ;
#17442=DIRECTION ( 'NONE',  ( 1.000000000000000000, 0.000000000000000000, 0.000000000000000000 ) ) ;
#17443=EDGE_CURVE ( 'NONE', #23822, #13567, #26646, .T. ) ;
#17444=CARTESIAN_POINT ( 'NONE',  ( 15.28076414829719099, -3.924379092781201450, -2.583448059524448226 ) ) ;
#17445=CARTESIAN_POINT ( 'NONE',  ( 36.19345537505340360, -2.233535067971714305, -5.855262071939852042 ) ) ;
#17447=CARTESIAN_POINT ( 'NONE',  ( 24.12089549473325789, 0.5573315953133365364, -5.091603771319967109 ) ) ;
#17453=DIRECTION ( 'NONE',  ( 0.000000000000000000, -0.000000000000000000, -1.000000000000000000 ) ) ;
#17458=CARTESIAN_POINT ( 'NONE',  ( 33.68527224689047017, -3.841537723288600326, 5.136372516007956968 ) ) ;
#17464=VECTOR ( 'NONE', #134, 1000.000000000000000 ) ;
#17472=CARTESIAN_POINT ( 'NONE',  ( 22.16804255864639117, 4.482405448724880337, 3.705173013356440670 ) ) ;
#17477=CARTESIAN_POINT ( 'NONE',  ( -62.92837670882106238, -39.37473357531882101, 6.000000000000000000 ) ) ;
#17481=CARTESIAN_POINT ( 'NONE',  ( 24.28285221899144375, 2.481502257502904651, -4.080882954547480956 ) ) ;
#17485=DIRECTION ( 'NONE',  ( 1.682730792515357087E-16, -1.000000000000000000, 0.000000000000000000 ) ) ;
#17489=CARTESIAN_POINT ( 'NONE',  ( 86.52980085923458375, 1.163345319512251841, 5.105528906334227734 ) ) ;
#17490=CARTESIAN_POINT ( 'NONE',  ( 28.07449379822080004, 1.807001228253011016, 3.913063849393144888 ) ) ;
#17493=CARTESIAN_POINT ( 'NONE',  ( -72.38040341225585905, -46.72818906933961358, 9.894038184624683652 ) ) ;
#17494=CARTESIAN_POINT ( 'NONE',  ( -72.84815947045233031, 2.429809908903064919, -10.96147798754375202 ) ) ;
#17496=CARTESIAN_POINT ( 'NONE',  ( 14.74399611399054955, -5.056622873111205507, 2.496408223985688402 ) ) ;
#17498=CARTESIAN_POINT ( 'NONE',  ( 35.79004886699985377, -3.279176249207559568, -5.792300729934813930 ) ) ;
#17501=PLANE ( 'NONE',  #1372 ) ;
#17507=ORIENTED_EDGE ( 'NONE', *, *, #4600, .T. ) ;
#17508=CARTESIAN_POINT ( 'NONE',  ( 34.45373390281926618, -1.156888603319897513, 5.566325156673125996 ) ) ;
#17519=CARTESIAN_POINT ( 'NONE',  ( 24.06122720769042900, 3.344954272100802761, 3.221752643096582158 ) ) ;
#17523=CARTESIAN_POINT ( 'NONE',  ( 14.37770146410593597, -5.023675042449286643, -2.500000000000009326 ) ) ;
#17526=CARTESIAN_POINT ( 'NONE',  ( 25.40522689125253564, 0.6233671799178808204, 4.602606971976870298 ) ) ;
#17535=B_SPLINE_CURVE_WITH_KNOTS ( 'NONE', 3,
 ( #5154, #29861, #30691, #5559, #14599, #11303, #27376, #36245, #2284, #26976, #18100, #11108, #26780, #8219, #2498, #36850, #39521, #36647, #36054, #33782, #8426, #21210, #30478, #27171, #1675, #2087, #23868, #20790, #8022, #20382, #33385, #14808, #21004, #11712, #17282, #32961, #39115, #39318, #14407, #23679, #24288, #17691, #26575, #10911 ),
 .UNSPECIFIED., .F., .F.,
 ( 4, 1, 1, 2, 2, 1, 1, 1, 1, 1, 1, 1, 1, 2, 2, 1, 1, 1, 1, 1, 1, 2, 2, 1, 1, 1, 1, 1, 2, 2, 1, 1, 1, 4 ),
 ( 0.000000000000000000, 0.2462456440929807477, 0.2481694381874572086, 0.2491313352346954668, 0.2500932322819336973, 0.2539408204708873407, 0.2616359968487950716, 0.2770263496046105334, 0.3078070551162413460, 0.3693684661395030822, 0.4924912881860259994, 0.4963388763749802535, 0.4982626704694577136, 0.4992245675166965269, 0.5001864645639352291, 0.5078816409418428490, 0.5232719936976579778, 0.5540526992092877911, 0.6156141102325467518, 0.7387369322790644510, 0.7464321086569721819, 0.7483559027514491424, 0.7502796968459262139, 0.7541272850348799128, 0.7695176377906951526, 0.8002983433023260762, 0.8618597543255873683, 0.8695549307034944331, 0.8734025188924475769, 0.8753263129869242043, 0.8772501070814008317, 0.8926404598372128518, 0.9234211653488365590, 0.9849825763720841953 ),
 .UNSPECIFIED. ) ;
#17540=CARTESIAN_POINT ( 'NONE',  ( 82.38753728249152175, 5.816132372599501110, 5.999999999999998224 ) ) ;
#17541=CARTESIAN_POINT ( 'NONE',  ( 23.94338804316802438, 3.829326634665836782, 2.990621344434266415 ) ) ;
#17546=CARTESIAN_POINT ( 'NONE',  ( 23.05616258268533159, 0.3493913546029596695, -5.956410236909607470 ) ) ;
#17548=CARTESIAN_POINT ( 'NONE',  ( 10.58508780786439374, 19.59913305159139441, -2.500000000000000000 ) ) ;
#17551=LINE ( 'NONE', #14470, #20999 ) ;
#17552=CYLINDRICAL_SURFACE ( 'NONE', #36731, 10.00000000000000533 ) ;
#17553=CARTESIAN_POINT ( 'NONE',  ( 37.18584374690863115, -2.963240108125716699, -5.999995304506872351 ) ) ;
#17554=DIRECTION ( 'NONE',  ( 0.000000000000000000, -1.000000000000000000, 0.000000000000000000 ) ) ;
#17565=AXIS2_PLACEMENT_3D ( 'NONE', #7532, #7332, #13912 ) ;
#17568=CARTESIAN_POINT ( 'NONE',  ( 86.38407091574619301, -0.4420343715668084150, 5.843987706619403255 ) ) ;
#17579=CARTESIAN_POINT ( 'NONE',  ( 17.55902072822312832, 11.95912221219358607, -2.500000000000012434 ) ) ;
#17583=VERTEX_POINT ( 'NONE', #36834 ) ;
#17585=DIRECTION ( 'NONE',  ( 1.000000000000000000, 0.000000000000000000, 0.000000000000000000 ) ) ;
#17588=CARTESIAN_POINT ( 'NONE',  ( 21.85643539959774273, 11.92045248574714300, 0.01447246376323708950 ) ) ;
#17591=CARTESIAN_POINT ( 'NONE',  ( -80.17799140349276854, 10.47773439577431631, 6.111419866882078722 ) ) ;
#17593=CARTESIAN_POINT ( 'NONE',  ( 14.63786011423607114, -4.769655762138079069, 2.500000000000003109 ) ) ;
#17594=CARTESIAN_POINT ( 'NONE',  ( -79.46433441440639456, 10.38016200751361851, -7.169073381784508925 ) ) ;
#17604=CARTESIAN_POINT ( 'NONE',  ( 87.91080083688075320, -0.3878594015929205940, 3.341311120819375979 ) ) ;
#17610=CARTESIAN_POINT ( 'NONE',  ( 36.98008712529284026, -2.957219606516312993, 5.978034981325530239 ) ) ;
#17613=CARTESIAN_POINT ( 'NONE',  ( 88.63860240521751166, -1.205360666695063365, 1.162049942889349818 ) ) ;
#17614=CARTESIAN_POINT ( 'NONE',  ( -71.19005252498740788, -21.75701227484909950, 5.995519781525873171 ) ) ;
#17615=CARTESIAN_POINT ( 'NONE',  ( 32.83291512613813268, -0.9452453669511491352, -5.330768491123616393 ) ) ;
#17621=EDGE_CURVE ( 'NONE', #12163, #7910, #4947, .T. ) ;
#17628=CARTESIAN_POINT ( 'NONE',  ( 24.08422046648111348, 0.7197875013252986731, 5.070242109043855194 ) ) ;
#17635=CARTESIAN_POINT ( 'NONE',  ( 36.10284116201629701, 0.9159659085930716982, 5.999999999999999112 ) ) ;
#17637=FACE_OUTER_BOUND ( 'NONE', #27157, .T. ) ;
#17640=CARTESIAN_POINT ( 'NONE',  ( 22.30947672616612110, 4.711638434871365355, -3.402558136683496048 ) ) ;
#17645=CARTESIAN_POINT ( 'NONE',  ( 22.32070839933769690, 6.022037317923602195, -2.674548383380369376 ) ) ;
#17650=CARTESIAN_POINT ( 'NONE',  ( 87.06807637922989329, 0.009568187950425697044, -5.830412620327568796 ) ) ;
#17655=CARTESIAN_POINT ( 'NONE',  ( 17.05035514590630186, -3.238823860988104375, -2.847664724424037175 ) ) ;
#17656=CARTESIAN_POINT ( 'NONE',  ( 21.25246063494507709, 3.318379548260936396, -3.523358493422822146 ) ) ;
#17657=DIRECTION ( 'NONE',  ( 1.000000000000000000, 0.000000000000000000, -0.000000000000000000 ) ) ;
#17658=CARTESIAN_POINT ( 'NONE',  ( 26.23190562806670201, 1.330159553823745400, -4.349047677718131055 ) ) ;
#17659=CARTESIAN_POINT ( 'NONE',  ( 30.19012588776831052, -3.695353065752804866, -4.605591824749690311 ) ) ;
#17661=CARTESIAN_POINT ( 'NONE',  ( 33.68739442648515592, -3.100371856129508163, 5.464130651605732858 ) ) ;
#17666=CARTESIAN_POINT ( 'NONE',  ( 34.14266073545298497, -3.850829098075486456, 5.232169337272932985 ) ) ;
#17668=CARTESIAN_POINT ( 'NONE',  ( 27.25263714637349466, -3.363254830459760925, -4.292962941291143864 ) ) ;
#17672=ORIENTED_EDGE ( 'NONE', *, *, #4112, .F. ) ;
#17673=ORIENTED_EDGE ( 'NONE', *, *, #40496, .F. ) ;
#17677=CARTESIAN_POINT ( 'NONE',  ( 14.75054140592678920, -5.115303881675558273, 2.500062186397897790 ) ) ;
#17678=ORIENTED_EDGE ( 'NONE', *, *, #37782, .T. ) ;
#17680=CARTESIAN_POINT ( 'NONE',  ( -70.92837670882107659, -65.19654454972992141, 0.000000000000000000 ) ) ;
#17682=ADVANCED_FACE ( 'NONE', ( #30054 ), #36428, .F. ) ;
#17683=CARTESIAN_POINT ( 'NONE',  ( 22.98309003772910231, 3.680112614338335586, 3.663265023080902960 ) ) ;
#17685=VECTOR ( 'NONE', #13225, 1000.000000000000000 ) ;
#17689=PRODUCT_DEFINITION_SHAPE ( 'NONE', 'NONE',  #15152 ) ;
#17691=CARTESIAN_POINT ( 'NONE',  ( 15.19171747855076937, -3.846800078502829567, -2.577432944240219292 ) ) ;
#17692=FACE_BOUND ( 'NONE', #12581, .T. ) ;
#17694=CARTESIAN_POINT ( 'NONE',  ( 23.48117969904087232, 2.411688234495183103, -4.382658167535084637 ) ) ;
#17702=CARTESIAN_POINT ( 'NONE',  ( 86.96272348114096928, 0.6770660828398197273, -5.145113290124521122 ) ) ;
#17703=CARTESIAN_POINT ( 'NONE',  ( 33.42314280165584961, -3.731500252021894948, -5.214789010484834897 ) ) ;
#17705=CARTESIAN_POINT ( 'NONE',  ( 14.72985901586098834, -5.055727223184880437, 2.496285957478483919 ) ) ;
#17707=CARTESIAN_POINT ( 'NONE',  ( 36.49090136167231435, -2.266358383019391187, -5.901685711910262810 ) ) ;
#17714=VERTEX_POINT ( 'NONE', #19323 ) ;
#17715=CARTESIAN_POINT ( 'NONE',  ( 33.45644231954936032, -3.829387444398935969, 5.093826274657804021 ) ) ;
#17718=CARTESIAN_POINT ( 'NONE',  ( -9.796229648729232409, -33.54387950140292673, 2.500000000000000000 ) ) ;
#17719=ORIENTED_EDGE ( 'NONE', *, *, #1016, .F. ) ;
#17720=DIRECTION ( 'NONE',  ( -0.000000000000000000, 0.000000000000000000, 1.000000000000000000 ) ) ;
#17723=CARTESIAN_POINT ( 'NONE',  ( 85.76276611814323303, 0.6947132229710382134, -5.930772436601586151 ) ) ;
#17728=CARTESIAN_POINT ( 'NONE',  ( 21.71529350491948662, 6.299837801999743192, 3.203318375066928514 ) ) ;
#17734=CARTESIAN_POINT ( 'NONE',  ( 24.12314213337219471, 0.4937462159112996907, 5.095090315528720382 ) ) ;
#17744=CARTESIAN_POINT ( 'NONE',  ( 36.40251230580387443, -3.583875492086917358, -5.773602733574922929 ) ) ;
#17749=CARTESIAN_POINT ( 'NONE',  ( 14.69558838330753936, -3.003688195628454238, -6.000000000000000888 ) ) ;
#17750=CARTESIAN_POINT ( 'NONE',  ( 29.35164812155991854, -2.438811642646435018, -5.575705495130315548 ) ) ;
#17751=ORIENTED_EDGE ( 'NONE', *, *, #38760, .T. ) ;
#17752=CARTESIAN_POINT ( 'NONE',  ( -80.88307586610955013, -6.600601063053268547, 1.034001549581234691 ) ) ;
#17753=CARTESIAN_POINT ( 'NONE',  ( 23.05858422394668494, 0.3510769165348703313, -5.953811706270123238 ) ) ;
#17754=CYLINDRICAL_SURFACE ( 'NONE', #5093, 15.73502530973474478 ) ;
#17758=AXIS2_PLACEMENT_3D ( 'NONE', #35285, #26209, #4770 ) ;
#17759=CARTESIAN_POINT ( 'NONE',  ( -72.12675090261940625, -48.04006991943428062, 9.928906425387692636 ) ) ;
#17760=CARTESIAN_POINT ( 'NONE',  ( 25.73262918993416903, 2.635805330050151163, -3.523857060088606552 ) ) ;
#17761=CARTESIAN_POINT ( 'NONE',  ( 30.86448711380490906, -3.396658003756702016, -4.948646710216845435 ) ) ;
#17764=CARTESIAN_POINT ( 'NONE',  ( -72.42837670882107659, -47.31363652731821645, 5.809475019311128641 ) ) ;
#17769=CARTESIAN_POINT ( 'NONE',  ( 23.61768953064343179, 2.039297767802271899, -4.577865503187037888 ) ) ;
#17783=ORIENTED_EDGE ( 'NONE', *, *, #36814, .T. ) ;
#17786=CARTESIAN_POINT ( 'NONE',  ( 22.26369084603574322, -3.082934178409861392, 3.582914324214749868 ) ) ;
#17794=FACE_OUTER_BOUND ( 'NONE', #8223, .T. ) ;
#17796=CARTESIAN_POINT ( 'NONE',  ( 14.77315594796849574, 13.19392823276453441, -2.500000000000005773 ) ) ;
#17797=CARTESIAN_POINT ( 'NONE',  ( 18.06312555530757180, 13.66100638925423638, 2.499999999999999112 ) ) ;
#17798=CARTESIAN_POINT ( 'NONE',  ( 21.85643539959776049, -3.417000210761661272, 14.19984240075801374 ) ) ;
#17800=CARTESIAN_POINT ( 'NONE',  ( -81.60310545337347321, 10.48532311983779231, 2.459591873363855985 ) ) ;
#17802=CARTESIAN_POINT ( 'NONE',  ( 14.69558626228978149, -4.492521580652499402, 2.500000000002278622 ) ) ;
#17803=CARTESIAN_POINT ( 'NONE',  ( -73.75202015018511759, 8.355648094992089270, -9.596423266730763402 ) ) ;
#17805=CARTESIAN_POINT ( 'NONE',  ( 34.79254740251967348, -3.836931395608193185, -5.375521320436218886 ) ) ;
#17807=CARTESIAN_POINT ( 'NONE',  ( 14.69386405977045840, 12.90286227655693985, 2.499730877609119606 ) ) ;
#17817=B_SPLINE_CURVE_WITH_KNOTS ( 'NONE', 3,
 ( #13484, #26059, #34938, #10395, #9991, #29339 ),
 .UNSPECIFIED., .F., .F.,
 ( 4, 2, 4 ),
 ( 0.001562288773108196386, 0.004630526322482777721, 0.007698763871857358838 ),
 .UNSPECIFIED. ) ;
#17819=EDGE_CURVE ( 'NONE', #37746, #24052, #8195, .T. ) ;
#17821=CARTESIAN_POINT ( 'NONE',  ( 84.70654116317179216, 2.970325471579660981, -2.062712134826208299 ) ) ;
#17822=CARTESIAN_POINT ( 'NONE',  ( 32.22946493318451644, -2.099509172777830557, 5.989391533279509794 ) ) ;
#17825=CARTESIAN_POINT ( 'NONE',  ( 85.69091256600084705, 1.101904404422226147, 5.757845717007028519 ) ) ;
#17834=CARTESIAN_POINT ( 'NONE',  ( 27.32771548703534137, 1.129468208573155552, 4.470271327343472656 ) ) ;
#17841=CARTESIAN_POINT ( 'NONE',  ( 66.41194937274630661, -13.65448019739280028, 6.000000000000001776 ) ) ;
#17846=CARTESIAN_POINT ( 'NONE',  ( 22.65020874192035549, 4.493281994308780725, -3.164719311941372570 ) ) ;
#17849=CARTESIAN_POINT ( 'NONE',  ( 23.98959816390508593, 3.209834647534565377, 4.521976212143768770 ) ) ;
#17850=CARTESIAN_POINT ( 'NONE',  ( 21.86951112228127769, 3.097095171887178644, -3.923778634572244073 ) ) ;
#17854=CARTESIAN_POINT ( 'NONE',  ( 84.57490107788032674, 3.121871263001978924, -0.4841835102440271710 ) ) ;
#17856=ORIENTED_EDGE ( 'NONE', *, *, #13948, .F. ) ;
#17860=CARTESIAN_POINT ( 'NONE',  ( 14.85674990071718682, -5.934158909055215148, -2.520779269183912596 ) ) ;
#17863=CARTESIAN_POINT ( 'NONE',  ( 23.60906662612009299, 0.4468475687248973927, -5.506013801080326786 ) ) ;
#17866=CARTESIAN_POINT ( 'NONE',  ( 29.09901106016964434, 0.3518894619724439732, 4.748002456818146477 ) ) ;
#17867=CARTESIAN_POINT ( 'NONE',  ( 85.17388679999480416, 2.686372346413934409, 1.032998165733738816 ) ) ;
#17868=ORIENTED_EDGE ( 'NONE', *, *, #1157, .F. ) ;
#17871=CARTESIAN_POINT ( 'NONE',  ( 35.22132403397331757, -1.046696322805372503, 5.410263585848889001 ) ) ;
#17872=CARTESIAN_POINT ( 'NONE',  ( 26.17872147609876876, -2.762083417368125016, 4.292220639753399958 ) ) ;
#17875=CARTESIAN_POINT ( 'NONE',  ( 17.87230948671713193, -3.179145971208983568, -2.954519006336920217 ) ) ;
#17878=VERTEX_POINT ( 'NONE', #38853 ) ;
#17880=CARTESIAN_POINT ( 'NONE',  ( 8.290806648384990041, 0.000000000000000000, 6.000000000000000000 ) ) ;
#17891=CARTESIAN_POINT ( 'NONE',  ( 22.56545177997091756, 3.994598255509013374, 3.706573800970350607 ) ) ;
#17895=EDGE_CURVE ( 'NONE', #4105, #38156, #31791, .T. ) ;
#17898=CARTESIAN_POINT ( 'NONE',  ( -80.92837670882107659, 2.429809908903242555, 12.50000000000000000 ) ) ;
#17901=CARTESIAN_POINT ( 'NONE',  ( 22.42500037023215498, 3.508167257036367559, -4.192016948695993506 ) ) ;
#17907=CARTESIAN_POINT ( 'NONE',  ( 85.39749695915146788, 2.435202802470831873, -2.633776547657810774 ) ) ;
#17915=CARTESIAN_POINT ( 'NONE',  ( 22.92222552203326913, 2.655818790012281827, -3.783965687468869188 ) ) ;
#17918=CARTESIAN_POINT ( 'NONE',  ( -17.27251170661583402, 0.7293679304675921848, 6.000000000000000000 ) ) ;
#17919=ADVANCED_FACE ( 'NONE', ( #3914 ), #29792, .F. ) ;
#17920=DIRECTION ( 'NONE',  ( -0.000000000000000000, -1.000000000000000000, -0.000000000000000000 ) ) ;
#17924=CARTESIAN_POINT ( 'NONE',  ( 25.66379520857860896, 2.554708175624311295, 3.769253407694455937 ) ) ;
#17929=ORIENTED_EDGE ( 'NONE', *, *, #36087, .F. ) ;
#17931=CARTESIAN_POINT ( 'NONE',  ( 86.36844116871179722, -0.4091080490822271987, -5.842633456154400662 ) ) ;
#17937=DIRECTION ( 'NONE',  ( 8.398074759113475787E-17, -1.000000000000000000, 0.000000000000000000 ) ) ;
#17938=ORIENTED_EDGE ( 'NONE', *, *, #11586, .T. ) ;
#17939=CARTESIAN_POINT ( 'NONE',  ( 24.37389473963558828, 3.149138647862574025, 3.338671700856682634 ) ) ;
#17942=CARTESIAN_POINT ( 'NONE',  ( 22.35187765366807255, 4.908147690922692874, -3.032796251420805334 ) ) ;
#17945=CARTESIAN_POINT ( 'NONE',  ( 21.73414723497777601, 0.2237007742282378919, 9.085389038113099502 ) ) ;
#17946=CARTESIAN_POINT ( 'NONE',  ( 14.75311975069267767, -5.145954708339309569, -2.499999999999999556 ) ) ;
#17953=FACE_OUTER_BOUND ( 'NONE', #3307, .T. ) ;
#17954=CARTESIAN_POINT ( 'NONE',  ( 14.69558838330753936, 10.99631180437154399, 5.999999999999998224 ) ) ;
#17956=CARTESIAN_POINT ( 'NONE',  ( 27.87470673840761037, 2.608020033772324275, -0.5247038454205935620 ) ) ;
#17961=DIRECTION ( 'NONE',  ( 1.000000000000000000, 1.165409145176969993E-16, 0.000000000000000000 ) ) ;
#17963=DIRECTION ( 'NONE',  ( -0.2744342186262705430, -0.9616058754224562355, 0.000000000000000000 ) ) ;
#17966=CARTESIAN_POINT ( 'NONE',  ( 35.72922540656550439, -1.306583851340389568, -5.539915139646041098 ) ) ;
#17974=B_SPLINE_CURVE_WITH_KNOTS ( 'NONE', 3,
 ( #33171, #39528, #27178, #29866 ),
 .UNSPECIFIED., .F., .F.,
 ( 4, 4 ),
 ( -0.001266773094470111972, 0.007521117280178637142 ),
 .UNSPECIFIED. ) ;
#17975=CARTESIAN_POINT ( 'NONE',  ( 14.74770783127116225, -5.101789873208831594, -2.500101740053638721 ) ) ;
#17976=CARTESIAN_POINT ( 'NONE',  ( 24.65075606035322409, 2.451163913605999500, -4.035534303674817913 ) ) ;
#17986=EDGE_CURVE ( 'NONE', #218, #40623, #36940, .T. ) ;
#18000=CARTESIAN_POINT ( 'NONE',  ( 15.45142779812353595, 8.160990771695352919, -3.484307217422537128 ) ) ;
#18004=CARTESIAN_POINT ( 'NONE',  ( 18.51121960923875420, 13.22484341366685179, 2.500000000000000000 ) ) ;
#18005=CARTESIAN_POINT ( 'NONE',  ( 21.85643539959778536, -8.233350057040109249, -11.92691213149646678 ) ) ;
#18007=CARTESIAN_POINT ( 'NONE',  ( -80.33892546431293624, 10.54035603179613645, 3.406678657042826686 ) ) ;
#18011=VECTOR ( 'NONE', #10380, 1000.000000000000000 ) ;
#18012=CARTESIAN_POINT ( 'NONE',  ( -74.59285101708645982, 9.286242826285279861, -9.309355451202566911 ) ) ;
#18016=CARTESIAN_POINT ( 'NONE',  ( 14.77394331808939754, 12.30091350227530178, 2.512229182593968879 ) ) ;
#18023=CARTESIAN_POINT ( 'NONE',  ( 24.72039900981634020, 2.638341910851478289, -3.924397643197742980 ) ) ;
#18025=ORIENTED_EDGE ( 'NONE', *, *, #5584, .F. ) ;
#18027=CARTESIAN_POINT ( 'NONE',  ( 36.14556864329624375, -3.195503675045440417, 5.847788189304162998 ) ) ;
#18029=CARTESIAN_POINT ( 'NONE',  ( 88.07792789432249947, -1.225918755007668226, 4.438991276806098618 ) ) ;
#18038=ORIENTED_EDGE ( 'NONE', *, *, #25014, .F. ) ;
#18042=CARTESIAN_POINT ( 'NONE',  ( 23.11977184038386568, 0.3886633077729012564, 5.889684842570323653 ) ) ;
#18048=CARTESIAN_POINT ( 'NONE',  ( -70.92837670882107659, -48.61702805680358352, 10.00000000000000888 ) ) ;
#18049=CARTESIAN_POINT ( 'NONE',  ( 24.31117675895931640, -6.336924832510081096, 2.705487332722515070 ) ) ;
#18053=EDGE_CURVE ( 'NONE', #4540, #20545, #707, .T. ) ;
#18054=CARTESIAN_POINT ( 'NONE',  ( 22.40957643201438998, 4.835774058222286342, -3.128480170401936711 ) ) ;
#18056=CARTESIAN_POINT ( 'NONE',  ( 25.43482567069144906, -3.911874351919522041, 4.043259094187231284 ) ) ;
#18060=CARTESIAN_POINT ( 'NONE',  ( 87.47045099524558509, -1.608924759093422807, 4.367130927193085377 ) ) ;
#18063=CARTESIAN_POINT ( 'NONE',  ( 24.75839165839662925, 3.019244830385916956, -3.350409272483306111 ) ) ;
#18069=CARTESIAN_POINT ( 'NONE',  ( 14.71635582635168049, -5.056528932363767659, -2.496255067347275869 ) ) ;
#18070=CARTESIAN_POINT ( 'NONE',  ( 34.33124084974205914, -1.490659953222954082, -5.564618457436417920 ) ) ;
#18074=ORIENTED_EDGE ( 'NONE', *, *, #31418, .F. ) ;
#18075=CARTESIAN_POINT ( 'NONE',  ( 33.46294586609511867, -3.082559428606642893, 5.429100025444929756 ) ) ;
#18076=CARTESIAN_POINT ( 'NONE',  ( 0.000000000000000000, 10.37661300689600097, 6.000000000000000000 ) ) ;
#18081=CARTESIAN_POINT ( 'NONE',  ( 36.88836814539537556, -3.352193696304970771, 5.910347166897455651 ) ) ;
#18082=CARTESIAN_POINT ( 'NONE',  ( 26.14529050879839289, -2.760665599016054905, 4.287002928775177857 ) ) ;
#18088=DIRECTION ( 'NONE',  ( -0.9999026450364576490, -0.01395351027862084224, 0.000000000000000000 ) ) ;
#18091=CARTESIAN_POINT ( 'NONE',  ( 24.30393741781215411, 2.735322053734381864, 3.908150415328090599 ) ) ;
#18092=CARTESIAN_POINT ( 'NONE',  ( 14.74962925723615825, 13.05063958598015184, 2.500338280337064845 ) ) ;
#18096=AXIS2_PLACEMENT_3D ( 'NONE', #31649, #19282, #25463 ) ;
#18097=CARTESIAN_POINT ( 'NONE',  ( 14.77500326541903952, -5.175625724643098557, -2.499997102511863911 ) ) ;
#18098=ORIENTED_EDGE ( 'NONE', *, *, #36948, .T. ) ;
#18100=CARTESIAN_POINT ( 'NONE',  ( 25.54817441638135023, -2.736180225144035028, -4.193808521246229049 ) ) ;
#18103=CARTESIAN_POINT ( 'NONE',  ( 21.85572174241494636, 3.841057816001869796, -4.459226767376585521 ) ) ;
#18105=CARTESIAN_POINT ( 'NONE',  ( 21.85643539959775694, 2.564233178479530917, 15.28924334870111146 ) ) ;
#18110=CARTESIAN_POINT ( 'NONE',  ( 87.10205511408864254, 0.5205621796347451591, 5.292648712017772539 ) ) ;
#18117=CARTESIAN_POINT ( 'NONE',  ( 28.67087680535204797, -4.024283280459782119, 4.110896467804376009 ) ) ;
#18118=CARTESIAN_POINT ( 'NONE',  ( 36.19525661438556341, -2.229558765483345528, -5.855543198900774016 ) ) ;
#18124=CARTESIAN_POINT ( 'NONE',  ( -70.01240559167840161, -45.92514165124313763, 5.930240575752830701 ) ) ;
#18128=CARTESIAN_POINT ( 'NONE',  ( 36.98735379331689899, -2.280088017890153473, 5.924094764607088948 ) ) ;
#18129=( BOUNDED_SURFACE ( )  B_SPLINE_SURFACE ( 3, 2, ( 
 ( #10476, #15700, #31563 ),
 ( #78, #37707, #12810 ),
 ( #13573, #22097, #3186 ),
 ( #6036, #28252, #19949 ) ),
 .UNSPECIFIED., .F., .F., .T. ) 
 B_SPLINE_SURFACE_WITH_KNOTS ( ( 4, 4 ),
 ( 3, 3 ),
 ( 0.1160236983739658390, 0.1317050650460910299 ),
 ( 0.1027166521410490529, 1.000000000000000000 ),
 .UNSPECIFIED. ) 
 GEOMETRIC_REPRESENTATION_ITEM ( )  RATIONAL_B_SPLINE_SURFACE ( (
 ( 0.9864974513313498061, 0.9342728350895400657, 1.000000000000000000),
 ( 0.9864974513313498061, 0.9342728350895400657, 1.000000000000000000),
 ( 0.9864974513313498061, 0.9342728350895399547, 1.000000000000000000),
 ( 0.9864974513313498061, 0.9342728350895399547, 1.000000000000000000) ) ) 
 REPRESENTATION_ITEM ( '' )  SURFACE ( )  );
#18134=B_SPLINE_CURVE_WITH_KNOTS ( 'NONE', 3,
 ( #26939, #23642, #32734, #14564, #4529, #36611, #8182, #23452, #20754, #4912 ),
 .UNSPECIFIED., .F., .F.,
 ( 4, 2, 2, 2, 4 ),
 ( 0.000000000000000000, 0.2500000000000000000, 0.5000000000000000000, 0.7500000000000000000, 1.000000000000000000 ),
 .UNSPECIFIED. ) ;
#18137=DIRECTION ( 'NONE',  ( -0.000000000000000000, 1.000000000000000000, -0.000000000000000000 ) ) ;
#18140=CARTESIAN_POINT ( 'NONE',  ( -79.15689149791292323, 11.46365244476452361, 5.697679923243769373 ) ) ;
#18141=ORIENTED_EDGE ( 'NONE', *, *, #3218, .F. ) ;
#18145=CARTESIAN_POINT ( 'NONE',  ( 21.72385588348585372, 6.222764755813646076, 3.231099798339156948 ) ) ;
#18147=LINE ( 'NONE', #11960, #26158 ) ;
#18153=CARTESIAN_POINT ( 'NONE',  ( 25.40382443007142399, 0.6807430875769404643, 4.599443498573071665 ) ) ;
#18160=CYLINDRICAL_SURFACE ( 'NONE', #33624, 1.500000000000001332 ) ;
#18162=CARTESIAN_POINT ( 'NONE',  ( 32.63594197759655913, -2.548278591510585667, -5.894033951951210604 ) ) ;
#18174=CARTESIAN_POINT ( 'NONE',  ( 36.98740879322385666, -2.280155673325318766, -5.924112469671126036 ) ) ;
#18182=LINE ( 'NONE', #30974, #37277 ) ;
#18184=CARTESIAN_POINT ( 'NONE',  ( 22.00903206384833055, 1.428713110540158038, -6.428340196499899406 ) ) ;
#18200=CARTESIAN_POINT ( 'NONE',  ( 24.08037749381573178, 3.357674872353649587, 3.169849549870835226 ) ) ;
#18203=CARTESIAN_POINT ( 'NONE',  ( -12.99139449055068241, 13.37661300689600097, 6.000000000000000000 ) ) ;
#18211=CARTESIAN_POINT ( 'NONE',  ( 22.68001568621454567, -4.050230952900990111, -7.789969220879865652 ) ) ;
#18216=ADVANCED_FACE ( 'NONE', ( #32807 ), #4595, .F. ) ;
#18217=CARTESIAN_POINT ( 'NONE',  ( -79.02496048640330173, 11.44822657882088457, -5.882923361518916927 ) ) ;
#18218=DIRECTION ( 'NONE',  ( 1.000000000000000000, 0.000000000000000000, 0.000000000000000000 ) ) ;
#18219=CARTESIAN_POINT ( 'NONE',  ( 36.44626315252003224, -1.730720475607963271, -5.729706151067262887 ) ) ;
#18228=CARTESIAN_POINT ( 'NONE',  ( 18.34140839124202316, 13.39279901796001049, -2.500000000000000000 ) ) ;
#18229=CARTESIAN_POINT ( 'NONE',  ( 37.20163862818894529, -2.760798311994886678, -5.998390365511268918 ) ) ;
#18230=CARTESIAN_POINT ( 'NONE',  ( 24.43632265556720284, 2.958562433187153395, -3.677099187153833437 ) ) ;
#18233=CARTESIAN_POINT ( 'NONE',  ( 33.66569764252319885, -3.445949192026814600, 5.444075323708291059 ) ) ;
#18236=CARTESIAN_POINT ( 'NONE',  ( 84.60690941119878516, 3.085063967761199066, 1.108375916024202379 ) ) ;
#18239=ORIENTED_EDGE ( 'NONE', *, *, #29119, .F. ) ;
#18240=DIRECTION ( 'NONE',  ( -1.000000000000000000, -1.165409145176970240E-16, 0.000000000000000000 ) ) ;
#18244=CIRCLE ( 'NONE', #36019, 24.28220113893567245 ) ;
#18249=CIRCLE ( 'NONE', #37337, 12.80480339192541628 ) ;
#18257=FACE_OUTER_BOUND ( 'NONE', #22578, .T. ) ;
#18258=CARTESIAN_POINT ( 'NONE',  ( 22.89983194485769502, 4.229321078703802250, -3.183991982619256422 ) ) ;
#18263=DIRECTION ( 'NONE',  ( -0.9999026450364576490, -0.01395351027862084224, 0.000000000000000000 ) ) ;
#18266=CARTESIAN_POINT ( 'NONE',  ( 85.39947451146549895, 1.536583868559685762, 5.410284084896357371 ) ) ;
#18267=CARTESIAN_POINT ( 'NONE',  ( 16.43736497953263864, 10.14549375742940640, 2.723904612540104075 ) ) ;
#18274=CARTESIAN_POINT ( 'NONE',  ( 14.68480434038803928, -5.054507705527442774, -2.495523734227267365 ) ) ;
#18279=CARTESIAN_POINT ( 'NONE',  ( 37.04537786116272713, -2.801074063609814147, 5.988225179720371827 ) ) ;
#18282=CARTESIAN_POINT ( 'NONE',  ( 86.13511395365257783, 1.606676384832600224, -4.558527568769633831 ) ) ;
#18284=ORIENTED_EDGE ( 'NONE', *, *, #1888, .F. ) ;
#18286=CARTESIAN_POINT ( 'NONE',  ( 36.13391060751988704, -1.528180889880398352, 5.641554834256164774 ) ) ;
#18287=CARTESIAN_POINT ( 'NONE',  ( 18.12002341025573315, -2.855556945250876666, 3.034465906229363963 ) ) ;
#18290=EDGE_LOOP ( 'NONE', ( #35419, #8861 ) ) ;
#18299=CARTESIAN_POINT ( 'NONE',  ( 21.84524191181414210, 2.598441008144188213, 5.474373194479982274 ) ) ;
#18300=CARTESIAN_POINT ( 'NONE',  ( 32.12397651727874148, 0.2264795177381662139, 4.744950101384926455 ) ) ;
#18309=CARTESIAN_POINT ( 'NONE',  ( 24.20993443650717936, 2.833309178738531386, -3.852635856680939774 ) ) ;
#18312=CARTESIAN_POINT ( 'NONE',  ( 21.85643539959778181, 2.105182337828026995, -13.78739850581801996 ) ) ;
#18317=CARTESIAN_POINT ( 'NONE',  ( 88.63860240521751166, -1.205360666695063365, 1.162049942889349818 ) ) ;
#18321=CARTESIAN_POINT ( 'NONE',  ( 15.59010151301636604, -3.705400104462427624, 2.635672183462121954 ) ) ;
#18322=CARTESIAN_POINT ( 'NONE',  ( 21.58863023475808873, 7.202558683720228672, -2.923977588977705544 ) ) ;
#18324=CARTESIAN_POINT ( 'NONE',  ( 20.42702919835091535, 3.672993461847502417, -3.394529954607447220 ) ) ;
#18331=CARTESIAN_POINT ( 'NONE',  ( 37.17917179609320755, -2.754412960886113204, 6.000950219249740591 ) ) ;
#18334=EDGE_CURVE ( 'NONE', #10306, #11412, #21248, .T. ) ;
#18345=CARTESIAN_POINT ( 'NONE',  ( 8.290806648384990041, 0.000000000000000000, -2.500000000000000000 ) ) ;
#18347=EDGE_LOOP ( 'NONE', ( #12278, #25536, #6974, #33585 ) ) ;
#18348=CARTESIAN_POINT ( 'NONE',  ( 24.65197495220076007, 2.989504840433797828, 3.507439046191596521 ) ) ;
#18350=DIRECTION ( 'NONE',  ( -0.000000000000000000, -0.000000000000000000, -1.000000000000000000 ) ) ;
#18351=ADVANCED_FACE ( 'NONE', ( #30517 ), #40174, .T. ) ;
#18353=AXIS2_PLACEMENT_3D ( 'NONE', #6176, #37857, #15425 ) ;
#18355=VERTEX_POINT ( 'NONE', #30935 ) ;
#18368=DIRECTION ( 'NONE',  ( -1.000000000000000000, 0.000000000000000000, 0.000000000000000000 ) ) ;
#18370=CARTESIAN_POINT ( 'NONE',  ( 33.61282307965942806, -4.196488527906213406, -4.700131347630155609 ) ) ;
#18374=CARTESIAN_POINT ( 'NONE',  ( 25.98198111045553205, 0.8794612723162963386, -4.427497433388436932 ) ) ;
#18380=CARTESIAN_POINT ( 'NONE',  ( 30.81598109780163952, 0.5927272948842338129, -4.684903830278420500 ) ) ;
#18382=LINE ( 'NONE', #15092, #30146 ) ;
#18383=FACE_OUTER_BOUND ( 'NONE', #28308, .T. ) ;
#18390=CARTESIAN_POINT ( 'NONE',  ( 24.08254445156938317, 2.354971793711281958, -4.219079743025244689 ) ) ;
#18396=CARTESIAN_POINT ( 'NONE',  ( 87.68638643695580015, -2.222987235672965411, -2.753905389729575326 ) ) ;
#18405=EDGE_CURVE ( 'NONE', #18458, #5730, #10896, .T. ) ;
#18410=LINE ( 'NONE', #18203, #26940 ) ;
#18416=CARTESIAN_POINT ( 'NONE',  ( 22.32844273176644379, 5.552903595841022444, -4.279453667248723114 ) ) ;
#18418=CARTESIAN_POINT ( 'NONE',  ( -72.17678919972044582, 5.298235119234846913, 9.922868473773599263 ) ) ;
#18419=CARTESIAN_POINT ( 'NONE',  ( 37.17104416159511970, -2.975766693752441405, 5.995325537273664018 ) ) ;
#18421=CARTESIAN_POINT ( 'NONE',  ( -81.79890681550139675, 10.46299657128043492, 0.6911394749367770762 ) ) ;
#18422=CARTESIAN_POINT ( 'NONE',  ( 32.90341074813867550, -3.215396174707138677, -5.341771038058501730 ) ) ;
#18423=CARTESIAN_POINT ( 'NONE',  ( 37.10444278664265028, -3.126632674519886468, -5.976181500518823242 ) ) ;
#18425=CARTESIAN_POINT ( 'NONE',  ( -4.224659823956008253, -51.67615071827237472, 6.000000000000000000 ) ) ;
#18432=CARTESIAN_POINT ( 'NONE',  ( 36.87286983558979614, -2.097983711965031528, -5.866507389336803158 ) ) ;
#18433=CARTESIAN_POINT ( 'NONE',  ( 24.58590238555413876, 2.979194303875008387, -3.570749183279829264 ) ) ;
#18436=CARTESIAN_POINT ( 'NONE',  ( 35.50430187872925103, -1.785329816699790184, 5.747703001598215344 ) ) ;
#18439=CARTESIAN_POINT ( 'NONE',  ( 13.52694889643372278, 17.29870644234688370, 2.500000000000000000 ) ) ;
#18440=CARTESIAN_POINT ( 'NONE',  ( 88.51539661956502414, -1.738042312505858389, 3.005881034771096250 ) ) ;
#18444=CARTESIAN_POINT ( 'NONE',  ( 37.02167662054689146, -2.764188933150113048, -5.984526027905666901 ) ) ;
#18446=CARTESIAN_POINT ( 'NONE',  ( 24.63695973801421957, 2.986857212966991248, 3.523430893224142935 ) ) ;
#18458=VERTEX_POINT ( 'NONE', #3555 ) ;
#18463=CARTESIAN_POINT ( 'NONE',  ( -71.92837670882107659, -20.91513571952110340, 9.949874371066202983 ) ) ;
#18465=CARTESIAN_POINT ( 'NONE',  ( 24.35951259229402055, 3.143687006796874517, -3.365150753154290353 ) ) ;
#18466=EDGE_LOOP ( 'NONE', ( #33310, #32274, #38006, #20459 ) ) ;
#18468=CARTESIAN_POINT ( 'NONE',  ( 25.22633673370294360, -3.172752697882940343, -5.351597462314125586 ) ) ;
#18472=CARTESIAN_POINT ( 'NONE',  ( 86.86785128967072467, -0.4505172232112327757, -5.755800129507335328 ) ) ;
#18478=CARTESIAN_POINT ( 'NONE',  ( 23.83742322420201276, -3.141359013241465714, -3.807232997737503677 ) ) ;
#18482=CARTESIAN_POINT ( 'NONE',  ( 36.79712590745128864, -2.556887556061694600, 5.949479458347596506 ) ) ;
#18483=CARTESIAN_POINT ( 'NONE',  ( 85.88709644997106807, 1.885261416588465799, 4.127327262050844325 ) ) ;
#18488=CARTESIAN_POINT ( 'NONE',  ( 22.09655393983083371, -2.652383328716616973, 3.655099668123841905 ) ) ;
#18489=CARTESIAN_POINT ( 'NONE',  ( -17.69482985384421880, -29.56993018339339940, -6.000000000000000000 ) ) ;
#18490=CARTESIAN_POINT ( 'NONE',  ( 21.58863023475808873, 7.202558683720228672, -2.923977588977705544 ) ) ;
#18492=VERTEX_POINT ( 'NONE', #28852 ) ;
#18493=B_SPLINE_CURVE_WITH_KNOTS ( 'NONE', 3,
 ( #27779, #5969, #18934, #12544, #18510, #34404, #2906, #6591, #15638, #37645, #11918, #27985, #9450, #40532, #12340, #22032, #34609, #12747, #3323, #24913, #37449, #15842, #27585, #206, #25324, #40137, #37048, #8834, #21418, #7377, #32318, #6785, #19742, #3926, #16440, #25722, #38066, #13351, #19935, #38663, #16833, #38458, #25926, #28609, #31909, #35414, #4117, #20135, #10262, #3519, #417, #35011, #12956, #3721, #22443, #13161, #32125, #26132, #1024, #19339 ),
 .UNSPECIFIED., .F., .F.,
 ( 4, 1, 2, 2, 1, 1, 1, 1, 2, 2, 1, 1, 1, 1, 1, 2, 2, 1, 1, 1, 1, 2, 2, 1, 1, 1, 1, 1, 2, 2, 1, 1, 1, 1, 1, 1, 2, 2, 1, 1, 1, 1, 1, 2, 4 ),
 ( 0.000000000000000000, 0.03125000000000305311, 0.03515625000000274780, 0.03906250000000244249, 0.04687500000000294209, 0.05468750000000344169, 0.05859375000000369149, 0.06054687500000378170, 0.06152343750000379557, 0.06250000000000380251, 0.09374999999998534506, 0.1093749999999761024, 0.1171874999999714534, 0.1210937499999693440, 0.1230468749999680672, 0.1240234374999676509, 0.1249999999999672345, 0.1874999999999666656, 0.2187499999999664990, 0.2343749999999664158, 0.2421874999999664158, 0.2460937499999664158, 0.2499999999999664158, 0.3124999999999670264, 0.3437499999999674150, 0.3593749999999675815, 0.3671874999999676925, 0.3710937499999676370, 0.3730468749999676370, 0.3749999999999675815, 0.4062499999999664158, 0.4218749999999655831, 0.4296874999999649170, 0.4335937499999643063, 0.4355468749999643063, 0.4365234374999645839, 0.4370117187499647504, 0.4374999999999649170, 0.4687499999999821254, 0.4843749999999903411, 0.4921874999999944489, 0.4960937499999965583, 0.4980468749999982792, 0.4990234374999991118, 0.5000000000000000000 ),
 .UNSPECIFIED. ) ;
#18495=CARTESIAN_POINT ( 'NONE',  ( 27.68906107752918189, -4.318180587071351439, -3.785118428133491530 ) ) ;
#18496=EDGE_CURVE ( 'NONE', #16084, #30583, #39167, .T. ) ;
#18499=EDGE_CURVE ( 'NONE', #36144, #8080, #39308, .T. ) ;
#18504=CARTESIAN_POINT ( 'NONE',  ( 24.12638665588002596, 2.663754577735522489, 3.995026624097451240 ) ) ;
#18510=CARTESIAN_POINT ( 'NONE',  ( 86.47917723929778333, 1.220208172167279503, -4.908343648090710332 ) ) ;
#18514=CARTESIAN_POINT ( 'NONE',  ( 23.07119635075321185, 3.097555360989402651, -4.080821451665009647 ) ) ;
#18517=CARTESIAN_POINT ( 'NONE',  ( 21.85643539959773207, -2.612013071670181041, -15.99649826491319971 ) ) ;
#18523=CARTESIAN_POINT ( 'NONE',  ( 86.62997685915109969, 1.050822881766228845, -5.316720303788503799 ) ) ;
#18524=ORIENTED_EDGE ( 'NONE', *, *, #449, .F. ) ;
#18526=CARTESIAN_POINT ( 'NONE',  ( 14.93019310335909111, -6.111523010399976918, 2.531807211659590884 ) ) ;
#18529=CARTESIAN_POINT ( 'NONE',  ( 36.44800439370845169, -2.352474353827100018, -5.894990602592409701 ) ) ;
#18532=VERTEX_POINT ( 'NONE', #29256 ) ;
#18537=ORIENTED_EDGE ( 'NONE', *, *, #19124, .T. ) ;
#18538=CARTESIAN_POINT ( 'NONE',  ( 33.88294556138480118, -0.6033199263786843680, 5.261213554215595778 ) ) ;
#18543=CARTESIAN_POINT ( 'NONE',  ( -77.51841857730454421, -6.230424868427139273, -7.532757448271641287 ) ) ;
#18546=EDGE_LOOP ( 'NONE', ( #24527, #20605, #39976, #24621, #26907, #30733, #13107, #33968 ) ) ;
#18549=ORIENTED_EDGE ( 'NONE', *, *, #38202, .T. ) ;
#18550=CARTESIAN_POINT ( 'NONE',  ( 24.71585255522903779, 3.004271553411825835, 3.424932163101386706 ) ) ;
#18558=CARTESIAN_POINT ( 'NONE',  ( 14.86212623557473478, 12.07207427411234768, -2.525992259579474375 ) ) ;
#18568=CARTESIAN_POINT ( 'NONE',  ( 33.81722006525239266, -4.984950771528167124, -3.153948780582495726 ) ) ;
#18569=EDGE_CURVE ( 'NONE', #25263, #833, #24700, .T. ) ;
#18573=CARTESIAN_POINT ( 'NONE',  ( 21.73547365326574621, 0.2723378343146318215, -8.960011461284089762 ) ) ;
#18578=CARTESIAN_POINT ( 'NONE',  ( 29.42001906605359451, 1.119432858802278830, -4.432475847736385255 ) ) ;
#18579=CARTESIAN_POINT ( 'NONE',  ( 8.290806648384990041, 0.000000000000000000, 6.000000000000000000 ) ) ;
#18586=ADVANCED_FACE ( 'NONE', ( #16670 ), #22881, .T. ) ;
#18587=CARTESIAN_POINT ( 'NONE',  ( 21.44690707717986911, 7.928456536348717165, 2.757011952239331265 ) ) ;
#18599=DIRECTION ( 'NONE',  ( -0.000000000000000000, 1.000000000000000000, -0.000000000000000000 ) ) ;
#18602=CARTESIAN_POINT ( 'NONE',  ( 22.38252468730212996, 4.953197636376286184, 3.028858097227504320 ) ) ;
#18609=EDGE_CURVE ( 'NONE', #4341, #13150, #27824, .T. ) ;
#18614=CARTESIAN_POINT ( 'NONE',  ( 21.85643539959774273, 9.255709152629782110, 0.01215589129642568461 ) ) ;
#18617=CARTESIAN_POINT ( 'NONE',  ( -72.46955098809822005, 6.128517033932898705, 9.881631157665120568 ) ) ;
#18618=LINE ( 'NONE', #31205, #14778 ) ;
#18622=CARTESIAN_POINT ( 'NONE',  ( 33.45661454515796862, -3.832864999374546944, -5.089924726100075958 ) ) ;
#18624=CARTESIAN_POINT ( 'NONE',  ( 14.67649090451648597, 13.02133489615250106, 2.497019376560389414 ) ) ;
#18626=CARTESIAN_POINT ( 'NONE',  ( 29.78968071384544203, -3.771415970051185784, 4.475279941939479755 ) ) ;
#18632=CARTESIAN_POINT ( 'NONE',  ( 17.33476859172393603, 14.29741483272972147, -2.500000000000000000 ) ) ;
#18634=CARTESIAN_POINT ( 'NONE',  ( 25.95728207872785731, 0.9011556877583806191, -4.428986979826762038 ) ) ;
#18636=CARTESIAN_POINT ( 'NONE',  ( 24.54108476865473776, 2.742666202680888343, -3.872715312010981847 ) ) ;
#18639=CARTESIAN_POINT ( 'NONE',  ( 37.07071770796867582, -2.906269623872106855, 5.992180075661026173 ) ) ;
#18640=LINE ( 'NONE', #21342, #12558 ) ;
#18643=CARTESIAN_POINT ( 'NONE',  ( 88.47081344899795852, -1.206222823704210301, -3.524641158899461058 ) ) ;
#18648=CARTESIAN_POINT ( 'NONE',  ( 24.61222844760713002, 2.982919474122702308, 3.547505255288157855 ) ) ;
#18658=VERTEX_POINT ( 'NONE', #22025 ) ;
#18666=CARTESIAN_POINT ( 'NONE',  ( 33.89631951754260797, -5.457875755526142569, -0.7132651481052724174 ) ) ;
#18667=CARTESIAN_POINT ( 'NONE',  ( 24.01772313286779337, 3.314519433455826558, -3.335196132849951312 ) ) ;
#18672=CARTESIAN_POINT ( 'NONE',  ( 24.14839210154553584, 1.598524049810922998, 6.350534879451781300 ) ) ;
#18673=EDGE_CURVE ( 'NONE', #38156, #15393, #6710, .T. ) ;
#18674=CARTESIAN_POINT ( 'NONE',  ( -77.76488672280875392, -5.012270680665758427, -8.924360589981601422 ) ) ;
#18675=AXIS2_PLACEMENT_3D ( 'NONE', #8218, #5358, #21209 ) ;
#18676=FACE_OUTER_BOUND ( 'NONE', #31610, .T. ) ;
#18679=CARTESIAN_POINT ( 'NONE',  ( 87.89980060869044109, -1.794189136469996004, 3.743635721206352684 ) ) ;
#18683=CARTESIAN_POINT ( 'NONE',  ( 14.77500326541903952, -5.175625724643098557, -2.499997102511863911 ) ) ;
#18688=CARTESIAN_POINT ( 'NONE',  ( 86.00054146471580907, 0.2529338399765344580, 5.999804812770356932 ) ) ;
#18691=CARTESIAN_POINT ( 'NONE',  ( 32.77907637591459888, -0.9333423657278323571, 5.322365652056097574 ) ) ;
#18697=CARTESIAN_POINT ( 'NONE',  ( 20.92112565569648552, 4.582337785983522593, 2.646877878247182903 ) ) ;
#18699=CARTESIAN_POINT ( 'NONE',  ( 18.14764728852392750, -2.851772390853231531, 3.038777280519134649 ) ) ;
#18703=CARTESIAN_POINT ( 'NONE',  ( 27.06227200975126124, -4.553918775559605336, -3.575370272941529315 ) ) ;
#18704=VECTOR ( 'NONE', #32389, 1000.000000000000000 ) ;
#18705=ORIENTED_EDGE ( 'NONE', *, *, #28783, .F. ) ;
#18710=CARTESIAN_POINT ( 'NONE',  ( 24.26828315858369933, 2.497494390861238145, 4.073910292191768256 ) ) ;
#18711=CARTESIAN_POINT ( 'NONE',  ( 35.58747779558025570, -1.229805145029287727, 5.504146291393874790 ) ) ;
#18722=CARTESIAN_POINT ( 'NONE',  ( 23.93748849625432129, 2.937348812402350795, -3.838641491431229902 ) ) ;
#18725=AXIS2_PLACEMENT_3D ( 'NONE', #18579, #40403, #19209 ) ;
#18726=CARTESIAN_POINT ( 'NONE',  ( 21.85643539959774273, -9.053501261307662418, 13.64238141129353110 ) ) ;
#18733=CARTESIAN_POINT ( 'NONE',  ( 88.50738123939095203, -1.057966825106399389, -0.8062500484416172952 ) ) ;
#18735=EDGE_CURVE ( 'NONE', #561, #16288, #38615, .T. ) ;
#18738=CARTESIAN_POINT ( 'NONE',  ( 16.23297496238618720, -3.365206226087963159, 2.739004174318827367 ) ) ;
#18741=CARTESIAN_POINT ( 'NONE',  ( 35.87004182851519829, -2.084339523132501704, -5.804785566216419390 ) ) ;
#18743=CARTESIAN_POINT ( 'NONE',  ( 21.89858067459283575, 5.089326824990051179, 3.617611013575467105 ) ) ;
#18749=CARTESIAN_POINT ( 'NONE',  ( 35.36800336353066143, -3.790791895310993365, 5.512052037117470604 ) ) ;
#18752=CARTESIAN_POINT ( 'NONE',  ( 86.50956153430306017, -0.6400250991913265519, -5.705005027417270114 ) ) ;
#18757=CARTESIAN_POINT ( 'NONE',  ( -80.57566330002634913, -6.630847404920713117, -2.665206594670471940 ) ) ;
#18761=LINE ( 'NONE', #40175, #38951 ) ;
#18762=ORIENTED_EDGE ( 'NONE', *, *, #39866, .F. ) ;
#18763=CARTESIAN_POINT ( 'NONE',  ( 23.14338651803718250, 4.000357944295927837, 3.156986160450860446 ) ) ;
#18770=CARTESIAN_POINT ( 'NONE',  ( -71.12603986806550438, -45.62685002856374439, 5.997522800198533233 ) ) ;
#18772=CARTESIAN_POINT ( 'NONE',  ( 14.98826240343326965, 12.12410137783581199, -2.538583708695383745 ) ) ;
#18781=CARTESIAN_POINT ( 'NONE',  ( 31.64923038865762805, -3.528005414130610529, -5.019302312848182623 ) ) ;
#18785=CARTESIAN_POINT ( 'NONE',  ( 22.30416999533203892, 0.2663055805526909903, -7.088243610313228693 ) ) ;
#18792=EDGE_CURVE ( 'NONE', #28485, #15211, #8549, .T. ) ;
#18794=CARTESIAN_POINT ( 'NONE',  ( 37.19502771478310166, -2.749426064116375468, -6.000945458054299131 ) ) ;
#18815=CARTESIAN_POINT ( 'NONE',  ( 21.82816986786027158, 5.980044178900067564, 3.126748918376258235 ) ) ;
#18817=CARTESIAN_POINT ( 'NONE',  ( 18.16951175210537883, -3.146849537680269648, 2.997227928983285494 ) ) ;
#18821=CARTESIAN_POINT ( 'NONE',  ( 24.72895772277339077, 0.6241560937809621512, 4.782015836530520758 ) ) ;
#18826=EDGE_CURVE ( 'NONE', #34290, #36144, #40583, .T. ) ;
#18832=CARTESIAN_POINT ( 'NONE',  ( 22.43090457150155004, 1.240285785788341810, -8.908344141805525140 ) ) ;
#18835=CARTESIAN_POINT ( 'NONE',  ( -73.09841737725705002, 0.2944336502508215769, 9.825022498446474017 ) ) ;
#18836=CARTESIAN_POINT ( 'NONE',  ( 35.83985725928805266, -3.722406797855700056, 5.627729815070630082 ) ) ;
#18839=CARTESIAN_POINT ( 'NONE',  ( -80.59506793348410270, 11.48890230165596194, -2.592577747312847958 ) ) ;
#18842=CARTESIAN_POINT ( 'NONE',  ( 25.73466472507932679, 2.638154739548788541, -3.516479417547335729 ) ) ;
#18845=CARTESIAN_POINT ( 'NONE',  ( 16.78011557480152760, 9.616836425704338609, 2.806367541052271708 ) ) ;
#18850=CARTESIAN_POINT ( 'NONE',  ( 21.86238218247489939, 0.3889561109544238948, -7.946803484597631417 ) ) ;
#18851=CARTESIAN_POINT ( 'NONE',  ( 30.79110773244140731, -3.772180204026406969, -4.560163372754496791 ) ) ;
#18852=CARTESIAN_POINT ( 'NONE',  ( 24.57886943115599365, 2.978281377686288867, -3.576560291590100693 ) ) ;
#18856=CARTESIAN_POINT ( 'NONE',  ( 32.81185505326144636, -0.8379172344137845174, 5.327481557411383406 ) ) ;
#18860=CARTESIAN_POINT ( 'NONE',  ( 86.54108089765607303, -0.3148381559440514010, -5.858094985366312457 ) ) ;
#18861=CARTESIAN_POINT ( 'NONE',  ( 35.94440725716257390, -2.118452061082618076, -5.816392089891535555 ) ) ;
#18863=CARTESIAN_POINT ( 'NONE',  ( 24.40553902836886735, 2.951342829192842299, 3.698142355126557757 ) ) ;
#18865=DIRECTION ( 'NONE',  ( 0.01395351027862084224, -0.9999026450364577601, 0.000000000000000000 ) ) ;
#18866=EDGE_LOOP ( 'NONE', ( #19328, #3007, #15648, #600 ) ) ;
#18879=EDGE_CURVE ( 'NONE', #5466, #39349, #15554, .T. ) ;
#18882=CARTESIAN_POINT ( 'NONE',  ( 27.16049945410617994, -4.514626814156768475, 3.607957147575535650 ) ) ;
#18886=CARTESIAN_POINT ( 'NONE',  ( 22.87953249933443800, 4.317477008691624540, -3.087559474757433531 ) ) ;
#18887=ORIENTED_EDGE ( 'NONE', *, *, #24394, .T. ) ;
#18893=CARTESIAN_POINT ( 'NONE',  ( -76.47431036836700002, -5.779992581808538255, -8.329558765771590600 ) ) ;
#18897=CARTESIAN_POINT ( 'NONE',  ( 87.47409246771869107, -1.962666243356603557, 3.672687813029068771 ) ) ;
#18898=CARTESIAN_POINT ( 'NONE',  ( -70.92837670882107659, 13.87661300689599742, 0.000000000000000000 ) ) ;
#18901=CARTESIAN_POINT ( 'NONE',  ( 22.06632471839147414, 4.214975381128987841, 2.277617108976539129 ) ) ;
#18907=CARTESIAN_POINT ( 'NONE',  ( 25.29651566011737529, 1.736446006507980089, 4.154531085941302493 ) ) ;
#18909=CIRCLE ( 'NONE', #24163, 12.80480339192541628 ) ;
#18910=CARTESIAN_POINT ( 'NONE',  ( 87.04213330793400871, 0.5878691963681530464, -4.891134986362597914 ) ) ;
#18911=ORIENTED_EDGE ( 'NONE', *, *, #16086, .F. ) ;
#18918=CARTESIAN_POINT ( 'NONE',  ( 28.09640073134533367, -4.183647163201285935, -3.920990555712708492 ) ) ;
#18924=CARTESIAN_POINT ( 'NONE',  ( 35.97450302262141264, -3.154424668010459953, 5.821089261960223027 ) ) ;
#18926=CARTESIAN_POINT ( 'NONE',  ( 22.26021987840845284, 2.688082151531064223, 4.954761472530542221 ) ) ;
#18927=CARTESIAN_POINT ( 'NONE',  ( 14.77222812468937363, 12.33286846116137347, 2.511961485181785747 ) ) ;
#18934=CARTESIAN_POINT ( 'NONE',  ( 86.69898499333136499, 0.9733096701313710408, -5.030742382222590514 ) ) ;
#18935=CARTESIAN_POINT ( 'NONE',  ( 21.85643539959776760, -15.11462368761991293, 2.500000000000000000 ) ) ;
#18939=CARTESIAN_POINT ( 'NONE',  ( 21.84823020783428760, 4.269274562117517213, -4.178901852297197017 ) ) ;
#18942=CARTESIAN_POINT ( 'NONE',  ( 21.85643539959780313, 0.8081825263151607430, -15.79083533483346535 ) ) ;
#18947=CARTESIAN_POINT ( 'NONE',  ( 87.66750401967712492, -0.1145768689462967616, 4.387407120178886899 ) ) ;
#18952=CARTESIAN_POINT ( 'NONE',  ( 15.57034054627223085, -3.673666129765767341, 2.635867821429580982 ) ) ;
#18953=CARTESIAN_POINT ( 'NONE',  ( 36.99252390190989104, -2.719198568494679780, -5.979976041101225270 ) ) ;
#18955=CARTESIAN_POINT ( 'NONE',  ( 21.95206253975293009, 4.960245780819739991, 3.632525366124041533 ) ) ;
#18958=CARTESIAN_POINT ( 'NONE',  ( 30.71037367896834880, -3.512617482052606821, 4.877620608057760876 ) ) ;
#18960=VERTEX_POINT ( 'NONE', #9578 ) ;
#18961=CARTESIAN_POINT ( 'NONE',  ( 37.00923632130533747, -2.250050275659773114, 5.913415034251472413 ) ) ;
#18966=CARTESIAN_POINT ( 'NONE',  ( 86.77891424509762430, -1.040114302260652046, -5.346981141011549532 ) ) ;
#18968=ORIENTED_EDGE ( 'NONE', *, *, #35263, .F. ) ;
#18969=CARTESIAN_POINT ( 'NONE',  ( 88.12997514058099569, -0.6340463821490202045, -2.468799945080301761 ) ) ;
#18970=EDGE_CURVE ( 'NONE', #8010, #11160, #23882, .T. ) ;
#18971=CARTESIAN_POINT ( 'NONE',  ( -71.80703402346622966, 3.441338441424772743, -9.961354656704822119 ) ) ;
#18972=CYLINDRICAL_SURFACE ( 'NONE', #20066, 1.000000000000000888 ) ;
#18979=CARTESIAN_POINT ( 'NONE',  ( 22.42121470216353174, 4.796581755807473257, 3.154605090790354005 ) ) ;
#18987=CARTESIAN_POINT ( 'NONE',  ( 14.88717023490364966, 12.58473342882037471, -2.513050065054561522 ) ) ;
#18990=CARTESIAN_POINT ( 'NONE',  ( 19.12106624447652337, 7.213790669980742365, -3.190702850821951486 ) ) ;
#18999=FACE_OUTER_BOUND ( 'NONE', #533, .T. ) ;
#19001=CARTESIAN_POINT ( 'NONE',  ( 29.52748857962093965, -2.713093490715668743, -5.368793458836177201 ) ) ;
#19009=CARTESIAN_POINT ( 'NONE',  ( 37.09088143372432711, -3.108852245844890394, -5.978546864269264738 ) ) ;
#19012=CARTESIAN_POINT ( 'NONE',  ( 23.82967770391586626, -2.761398267376460769, -3.925595547265982255 ) ) ;
#19016=VECTOR ( 'NONE', #20813, 1000.000000000000000 ) ;
#19018=DIRECTION ( 'NONE',  ( 1.000000000000000000, 8.966158204770716457E-16, 0.000000000000000000 ) ) ;
#19025=CARTESIAN_POINT ( 'NONE',  ( 22.99364181696555676, 3.589457867690851067, 3.733328102171712626 ) ) ;
#19028=EDGE_CURVE ( 'NONE', #25150, #25263, #26052, .T. ) ;
#19031=CARTESIAN_POINT ( 'NONE',  ( 21.98812987590129708, 5.622928254491678324, 3.083847952653145708 ) ) ;
#19038=CARTESIAN_POINT ( 'NONE',  ( 24.69442438258014860, 0.6739242910027807287, 4.791210749312426742 ) ) ;
#19042=VECTOR ( 'NONE', #32426, 1000.000000000000000 ) ;
#19044=CARTESIAN_POINT ( 'NONE',  ( -70.92837670882107659, -23.80776546975053520, -10.00000000000000888 ) ) ;
#19045=CARTESIAN_POINT ( 'NONE',  ( 21.85643539959775694, 2.837881715527333260, -11.82040581148825353 ) ) ;
#19047=CARTESIAN_POINT ( 'NONE',  ( -75.23145188694429919, 8.172688008897852185, 9.065593416914579095 ) ) ;
#19048=DIRECTION ( 'NONE',  ( -0.000000000000000000, -0.000000000000000000, -1.000000000000000000 ) ) ;
#19053=CARTESIAN_POINT ( 'NONE',  ( 32.00641903142002320, -3.049359518210221776, -5.201773786605959238 ) ) ;
#19054=CARTESIAN_POINT ( 'NONE',  ( 37.01057800680626286, -2.248353986704187513, -5.912806876547849200 ) ) ;
#19055=FACE_OUTER_BOUND ( 'NONE', #1457, .T. ) ;
#19056=CARTESIAN_POINT ( 'NONE',  ( 17.79089637503647126, 8.596792681990928386, 2.958187967343824720 ) ) ;
#19061=CARTESIAN_POINT ( 'NONE',  ( 21.97109001347866553, 0.9630426953691740843, -7.010656934984691446 ) ) ;
#19066=CARTESIAN_POINT ( 'NONE',  ( 36.94063378041538215, -3.101443124462082146, 5.970284356405101356 ) ) ;
#19069=CARTESIAN_POINT ( 'NONE',  ( 86.22674662394152278, 0.2046669357502599595, -6.014203425234573963 ) ) ;
#19070=CARTESIAN_POINT ( 'NONE',  ( 24.97750119118845546, 3.110153433881029272, 2.920260296092602292 ) ) ;
#19072=CARTESIAN_POINT ( 'NONE',  ( 24.66036887970934544, 2.991013199203838901, 3.498539802152044853 ) ) ;
#19086=CARTESIAN_POINT ( 'NONE',  ( 28.09351773336840452, -4.184899630424881778, 3.919764035321353646 ) ) ;
#19089=CARTESIAN_POINT ( 'NONE',  ( 23.74582114624947238, 3.564727581926975475, -3.175216399458318683 ) ) ;
#19096=DIRECTION ( 'NONE',  ( 0.000000000000000000, -0.000000000000000000, -1.000000000000000000 ) ) ;
#19099=CARTESIAN_POINT ( 'NONE',  ( 85.08782340246310127, 1.754895396694989840, 5.093632142551737907 ) ) ;
#19103=CARTESIAN_POINT ( 'NONE',  ( 22.06908225159077119, 4.294879054371497418, -1.925114753942556156 ) ) ;
#19109=CARTESIAN_POINT ( 'NONE',  ( 85.58452164909124349, 1.000110208193303540, 5.791573931091940075 ) ) ;
#19111=CARTESIAN_POINT ( 'NONE',  ( 33.46269705087502899, -3.085794937887296641, 5.429061191812215803 ) ) ;
#19113=CARTESIAN_POINT ( 'NONE',  ( 86.62997685915109969, 1.050822881766228845, -5.316720303788503799 ) ) ;
#19116=CARTESIAN_POINT ( 'NONE',  ( 23.38715862913678478, 3.561327236325438683, 3.087504282192082616 ) ) ;
#19118=CARTESIAN_POINT ( 'NONE',  ( -69.62722026347231008, -46.36434999406230872, 9.915139134996609371 ) ) ;
#19122=CARTESIAN_POINT ( 'NONE',  ( -71.86802756984693019, 3.923644143335089929, 9.956082279489690379 ) ) ;
#19123=ORIENTED_EDGE ( 'NONE', *, *, #1516, .T. ) ;
#19124=EDGE_CURVE ( 'NONE', #13553, #22791, #25640, .T. ) ;
#19125=B_SPLINE_CURVE_WITH_KNOTS ( 'NONE', 3,
 ( #28174, #5600, #23908, #30308, #36282, #12530, #8254, #18140, #1712, #8057, #4990, #36482, #5394, #20826, #33422, #5192, #2120, #14638, #36680, #8462, #21046, #804, #4104, #13547, #196, #6973, #6578, #19122, #6370, #3310, #28805, #12732, #22829, #29200, #1014, #3506, #10051, #16429, #38448, #25508, #13149, #606, #9854, #19732, #25312, #38054, #3708, #32113, #22431, #25709, #37843, #28597, #7171, #15831, #38251, #35401, #31488, #28386, #16231, #23031, #12942, #9647, #31690, #32307, #29002, #34798, #34998, #16616 ),
 .UNSPECIFIED., .F., .F.,
 ( 4, 2, 2, 2, 2, 2, 2, 2, 2, 2, 2, 2, 2, 2, 2, 2, 2, 2, 2, 2, 2, 2, 2, 2, 2, 2, 2, 2, 2, 2, 2, 2, 2, 4 ),
 ( 0.0006286237102968045840, 0.003159057492149853694, 0.004424274383076385458, 0.005689491274002918091, 0.006954708164929450723, 0.008219925055855984222, 0.009485141946782512518, 0.01075035883770904428, 0.01201557572863557605, 0.01328079261956210608, 0.01454600951048863958, 0.01581122640141517308, 0.01707644329234170311, 0.01834166018326823661, 0.01960687707419476664, 0.02087209396512130014, 0.02340252774697436366, 0.02466774463790090063, 0.02593296152882743760, 0.02656556997429069394, 0.02719817841975395722, 0.02846339531068046991, 0.02909600375614372972, 0.02972861220160698606, 0.03099382909253349874, 0.03162643753799675161, 0.03225904598346000102, 0.03352426287438650676, 0.03478947976531301250, 0.03605469665623952519, 0.03731991354716603093, 0.03858513043809252974, 0.03985034732901904242, 0.04111556421994554816 ),
 .UNSPECIFIED. ) ;
#19128=CARTESIAN_POINT ( 'NONE',  ( 21.82789562172892417, 2.051186498413608561, 6.030864959255196389 ) ) ;
#19130=ORIENTED_EDGE ( 'NONE', *, *, #32052, .F. ) ;
#19133=VECTOR ( 'NONE', #148, 1000.000000000000000 ) ;
#19140=CARTESIAN_POINT ( 'NONE',  ( 22.60925884027456334, 3.558685826784935280, -4.008354383335261950 ) ) ;
#19141=ORIENTED_EDGE ( 'NONE', *, *, #18569, .F. ) ;
#19144=CARTESIAN_POINT ( 'NONE',  ( 21.85643539959776760, 9.193408351192362105, 7.099988578988766008 ) ) ;
#19148=CARTESIAN_POINT ( 'NONE',  ( 86.17769677085827595, 1.483769024673816661, 5.380928644057212828 ) ) ;
#19153=CARTESIAN_POINT ( 'NONE',  ( 21.52218790455891906, -2.808060335668637997, 3.561660395461073048 ) ) ;
#19154=CARTESIAN_POINT ( 'NONE',  ( 36.89719978986997972, -3.002184996989889054, -5.965098407995004237 ) ) ;
#19163=CARTESIAN_POINT ( 'NONE',  ( 32.01954582267668314, -3.753399427551567413, 4.807335171585498834 ) ) ;
#19166=CARTESIAN_POINT ( 'NONE',  ( 34.63535154135784211, -0.7851648049891344350, 5.278750410354886569 ) ) ;
#19169=ORIENTED_EDGE ( 'NONE', *, *, #22150, .F. ) ;
#19179=CARTESIAN_POINT ( 'NONE',  ( 22.24260148052792729, 5.041501173538935454, 3.209353097046206305 ) ) ;
#19185=CARTESIAN_POINT ( 'NONE',  ( -72.42837670882107659, -47.11702805680359063, 5.809475019311127753 ) ) ;
#19187=CARTESIAN_POINT ( 'NONE',  ( 15.05162924821635251, 12.14958264902990059, -2.534429217488545216 ) ) ;
#19190=B_SPLINE_CURVE_WITH_KNOTS ( 'NONE', 3,
 ( #15752, #34108, #28099, #123, #18419, #15335, #40653, #27496, #3233, #40436, #5882, #28305, #24402, #31007, #37759, #36960, #12455, #25024, #12245, #25230, #24819, #21937, #37361, #37561, #21323, #22148, #9568, #9356, #2812, #18836, #27687, #34511, #27889, #6287 ),
 .UNSPECIFIED., .F., .F.,
 ( 4, 2, 1, 1, 2, 2, 2, 1, 1, 2, 1, 2, 2, 1, 2, 1, 2, 2, 1, 2, 4 ),
 ( 0.8213160790108455789, 0.8227120471435722671, 0.8241080152762988442, 0.8268999515417521096, 0.8296918878072053749, 0.8300408798403869914, 0.8303898718735686080, 0.8310878559399325072, 0.8324838240726603056, 0.8436515691344798062, 0.8464435053999349590, 0.8478394735326628684, 0.8492354416653907778, 0.8548193141963014163, 0.8659870592581228044, 0.8715709317890331098, 0.8743628680544878184, 0.8771548043199426381, 0.8883225493817656915, 0.9106580395054132415, 1.000000000000000000 ),
 .UNSPECIFIED. ) ;
#19198=CARTESIAN_POINT ( 'NONE',  ( 17.20447520187076762, 12.11625420413208332, 2.499999999999993339 ) ) ;
#19199=CARTESIAN_POINT ( 'NONE',  ( 30.06379901557190237, -4.186058752285889639, 3.090730270791094636 ) ) ;
#19205=PLANE ( 'NONE',  #2631 ) ;
#19207=CARTESIAN_POINT ( 'NONE',  ( 33.45777346496446825, -3.169730459255029054, -5.428292747153331099 ) ) ;
#19208=CARTESIAN_POINT ( 'NONE',  ( 21.58554896752337982, 4.069564431507699531, -3.350826899357332689 ) ) ;
#19209=DIRECTION ( 'NONE',  ( -0.000000000000000000, 0.000000000000000000, -1.000000000000000000 ) ) ;
#19210=B_SPLINE_CURVE_WITH_KNOTS ( 'NONE', 5,
 ( #4377, #35275, #7043, #29481, #10720, #25990, #10329, #19610 ),
 .UNSPECIFIED., .F., .F.,
 ( 6, 2, 6 ),
 ( 0.000000000000000000, 0.5000000000000000000, 1.000000000000000000 ),
 .UNSPECIFIED. ) ;
#19212=CARTESIAN_POINT ( 'NONE',  ( 15.19569296197379238, -3.822826931744748968, -2.578053414575811608 ) ) ;
#19214=CARTESIAN_POINT ( 'NONE',  ( -79.81169712350360612, 10.44897077626513671, 6.725963864478613274 ) ) ;
#19216=FACE_OUTER_BOUND ( 'NONE', #14395, .T. ) ;
#19219=ORIENTED_EDGE ( 'NONE', *, *, #13709, .T. ) ;
#19225=CARTESIAN_POINT ( 'NONE',  ( 24.38892444693420458, 2.847891321149697230, 3.812990230678215742 ) ) ;
#19237=CARTESIAN_POINT ( 'NONE',  ( 24.72106036938118478, 0.6348158216212017591, 4.784554241740610614 ) ) ;
#19244=ORIENTED_EDGE ( 'NONE', *, *, #13349, .T. ) ;
#19245=CARTESIAN_POINT ( 'NONE',  ( 22.40307219844260800, 2.196575021783337522, 8.487454310335619923 ) ) ;
#19247=EDGE_LOOP ( 'NONE', ( #23485, #8389, #39410, #14966 ) ) ;
#19248=CARTESIAN_POINT ( 'NONE',  ( -75.48351715386579031, 8.403134493634572877, 10.29384773356716565 ) ) ;
#19249=CARTESIAN_POINT ( 'NONE',  ( 23.58564635679343269, 0.4093974991330989188, -5.530654786722362104 ) ) ;
#19253=CARTESIAN_POINT ( 'NONE',  ( 32.89832779772925875, -3.752711978480219646, -5.048536920064313982 ) ) ;
#19254=CARTESIAN_POINT ( 'NONE',  ( 36.87105087205511467, -2.087304334115438031, -5.864227613858936650 ) ) ;
#19256=CARTESIAN_POINT ( 'NONE',  ( 16.45636466660662833, 9.968736736387965536, 2.757778904987983726 ) ) ;
#19258=CARTESIAN_POINT ( 'NONE',  ( 30.67349724481533002, -3.593355625737403525, 4.777428303402127874 ) ) ;
#19261=EDGE_CURVE ( 'NONE', #36144, #31580, #14678, .T. ) ;
#19262=EDGE_CURVE ( 'NONE', #14452, #25263, #24160, .T. ) ;
#19264=CARTESIAN_POINT ( 'NONE',  ( 21.76310852954332020, 0.8497392545002346864, -7.746649034779642840 ) ) ;
#19265=CARTESIAN_POINT ( 'NONE',  ( 35.35174707496273072, -1.118750166776470989, -5.447475926327616236 ) ) ;
#19272=CARTESIAN_POINT ( 'NONE',  ( 86.75210013534866960, -0.2795847087395720298, -5.842668109216860195 ) ) ;
#19274=CARTESIAN_POINT ( 'NONE',  ( 24.75830837035764276, 3.019210359990082804, 3.350572556515618583 ) ) ;
#19282=DIRECTION ( 'NONE',  ( -0.000000000000000000, 0.000000000000000000, 1.000000000000000000 ) ) ;
#19289=CARTESIAN_POINT ( 'NONE',  ( 27.32683644248853483, -4.450517831252136070, 3.663591729240187611 ) ) ;
#19290=CARTESIAN_POINT ( 'NONE',  ( 21.85643539959779957, -14.30241103581959727, -6.272691714111175543 ) ) ;
#19291=CARTESIAN_POINT ( 'NONE',  ( 22.62733628673683128, 4.569048702858772515, -3.101284368409240155 ) ) ;
#19294=ORIENTED_EDGE ( 'NONE', *, *, #9827, .T. ) ;
#19298=CARTESIAN_POINT ( 'NONE',  ( -78.36124264143398932, -5.233282719009260120, -8.391784592071982019 ) ) ;
#19299=CYLINDRICAL_SURFACE ( 'NONE', #35360, 10.00000000000000888 ) ;
#19302=CARTESIAN_POINT ( 'NONE',  ( 87.65251942239244443, -2.181810347267220340, 2.926837865475490297 ) ) ;
#19309=CARTESIAN_POINT ( 'NONE',  ( 21.52001214132182483, -3.049911746754888409, -3.476945207078641076 ) ) ;
#19314=CARTESIAN_POINT ( 'NONE',  ( 20.42491269841142554, 3.667755154276754137, 3.394199623604145177 ) ) ;
#19315=CARTESIAN_POINT ( 'NONE',  ( 87.97568001472090771, -0.4607347734944167716, -3.153239710520575390 ) ) ;
#19323=CARTESIAN_POINT ( 'NONE',  ( 11.29080664838498826, -10.90558813203967148, -6.000000000000000000 ) ) ;
#19328=ORIENTED_EDGE ( 'NONE', *, *, #35184, .T. ) ;
#19333=CARTESIAN_POINT ( 'NONE',  ( 25.64976342364274586, 1.736051923866335223, 4.267932205033374338 ) ) ;
#19339=CARTESIAN_POINT ( 'NONE',  ( 86.46043323462474461, 1.241262327860113590, 4.894917242394325463 ) ) ;
#19343=CARTESIAN_POINT ( 'NONE',  ( 24.12346661364753686, 3.039791896184803832, -3.681378513681969000 ) ) ;
#19344=ORIENTED_EDGE ( 'NONE', *, *, #16956, .T. ) ;
#19348=CARTESIAN_POINT ( 'NONE',  ( 21.85643539959775339, 6.533355437427212919, 10.99619876466361212 ) ) ;
#19349=CARTESIAN_POINT ( 'NONE',  ( 21.86297326093951199, 3.431109414793612533, 3.921173740588492329 ) ) ;
#19352=CARTESIAN_POINT ( 'NONE',  ( 87.69705646362149309, -0.3167607505441215610, 5.204154330927820205 ) ) ;
#19355=CARTESIAN_POINT ( 'NONE',  ( 14.85462441431243796, -6.141020992384870425, 2.524821418939259932 ) ) ;
#19356=CARTESIAN_POINT ( 'NONE',  ( 37.00353525545608591, -2.736192746824828603, 5.981694629132673136 ) ) ;
#19359=CARTESIAN_POINT ( 'NONE',  ( 31.44233202302301677, -3.758924007052948824, 4.692007276047764464 ) ) ;
#19361=CARTESIAN_POINT ( 'NONE',  ( 25.29740619394358703, 1.738824998010557676, -4.154670075282512975 ) ) ;
#19362=CARTESIAN_POINT ( 'NONE',  ( 14.77500745536057813, -5.175466302041957789, 2.500000552286355759 ) ) ;
#19363=B_SPLINE_CURVE_WITH_KNOTS ( 'NONE', 3,
 ( #33942, #34358, #3278, #6543 ),
 .UNSPECIFIED., .F., .F.,
 ( 4, 4 ),
 ( 0.000000000000000000, 1.000000000000000000 ),
 .UNSPECIFIED. ) ;
#19369=CARTESIAN_POINT ( 'NONE',  ( 29.58564408153181091, -3.738900761003516315, 4.503399178519281065 ) ) ;
#19370=ORIENTED_EDGE ( 'NONE', *, *, #7055, .T. ) ;
#19372=CARTESIAN_POINT ( 'NONE',  ( 37.10400457017786380, -3.125854874071246847, 5.976292952369103517 ) ) ;
#19376=CARTESIAN_POINT ( 'NONE',  ( -17.27251170661583402, -8.656638842136340273, 6.000000000000000000 ) ) ;
#19379=VERTEX_POINT ( 'NONE', #12420 ) ;
#19381=EDGE_CURVE ( 'NONE', #34269, #23464, #31372, .T. ) ;
#19382=LINE ( 'NONE', #1070, #31131 ) ;
#19384=CARTESIAN_POINT ( 'NONE',  ( 22.67359053832636917, 4.412626292741369305, 3.229231584030726854 ) ) ;
#19386=CIRCLE ( 'NONE', #10805, 7.744449365083023729 ) ;
#19391=CARTESIAN_POINT ( 'NONE',  ( 16.78263025183486334, 9.614103373516703854, -2.806744980977545101 ) ) ;
#19399=CARTESIAN_POINT ( 'NONE',  ( -4.444218661349752963, -35.94265729135299381, -2.500000000000000000 ) ) ;
#19402=CARTESIAN_POINT ( 'NONE',  ( 21.85642290860490888, 10.16974183911659146, 2.500000000000000444 ) ) ;
#19403=CARTESIAN_POINT ( 'NONE',  ( 29.35164812155991854, -2.438811642646435018, -5.575705495130315548 ) ) ;
#19411=CARTESIAN_POINT ( 'NONE',  ( 36.58899555212334320, -2.079458374954772815, -5.884079940498502914 ) ) ;
#19415=CYLINDRICAL_SURFACE ( 'NONE', #5072, 24.28220113893567600 ) ;
#19419=CARTESIAN_POINT ( 'NONE',  ( 31.82339877122853622, -2.965063844033737794, 5.173209048694666023 ) ) ;
#19427=CARTESIAN_POINT ( 'NONE',  ( 30.84556462519947218, -3.521365950626897945, 4.867246454883694007 ) ) ;
#19428=CARTESIAN_POINT ( 'NONE',  ( 22.01069687017167098, 4.352078338492005649, 3.948474219383390160 ) ) ;
#19432=CARTESIAN_POINT ( 'NONE',  ( 24.75501771239566295, 3.017875978853254093, 3.356962914366536488 ) ) ;
#19436=ORIENTED_EDGE ( 'NONE', *, *, #6441, .T. ) ;
#19438=CARTESIAN_POINT ( 'NONE',  ( 24.74336839167079205, 0.5919242770734765013, 4.777722238485932138 ) ) ;
#19444=CIRCLE ( 'NONE', #1698, 10.00000000000000533 ) ;
#19446=VECTOR ( 'NONE', #14198, 1000.000000000000000 ) ;
#19449=CARTESIAN_POINT ( 'NONE',  ( 25.48218379196744721, -4.266488024150952185, 3.117641769822204090 ) ) ;
#19452=CARTESIAN_POINT ( 'NONE',  ( -77.08826645590907845, -4.719337535992750077, 7.895626637436674145 ) ) ;
#19453=CARTESIAN_POINT ( 'NONE',  ( 25.40538259160478063, 0.6392885239908961958, -4.601632460917159051 ) ) ;
#19456=DIRECTION ( 'NONE',  ( 0.000000000000000000, 1.000000000000000000, 0.000000000000000000 ) ) ;
#19458=CARTESIAN_POINT ( 'NONE',  ( 30.71159473002022722, -3.512327092394234018, -4.877982841742380948 ) ) ;
#19459=CARTESIAN_POINT ( 'NONE',  ( 27.81689091006495218, 1.845377269578770685, -3.904318808813068920 ) ) ;
#19461=CARTESIAN_POINT ( 'NONE',  ( 17.69936654701060874, 8.505593641349619816, 2.968812229095278088 ) ) ;
#19468=CARTESIAN_POINT ( 'NONE',  ( 22.22682478162485964, 0.9416584759426780415, -6.596347691557129522 ) ) ;
#19469=CARTESIAN_POINT ( 'NONE',  ( 29.51225972876092740, 1.208032713357963361, -4.232904474717664733 ) ) ;
#19470=DIRECTION ( 'NONE',  ( 1.000000000000000000, 0.000000000000000000, 0.000000000000000000 ) ) ;
#19471=ORIENTED_EDGE ( 'NONE', *, *, #8449, .T. ) ;
#19476=CARTESIAN_POINT ( 'NONE',  ( 85.51010218477300384, 1.603708918324822541, 5.381112834985590787 ) ) ;
#19480=CARTESIAN_POINT ( 'NONE',  ( -79.30159439629763085, 10.34987115379732536, -7.377286748778528747 ) ) ;
#19495=CARTESIAN_POINT ( 'NONE',  ( 21.85643539959776760, 1.710603452083953179E-15, 2.500000000000000000 ) ) ;
#19499=CARTESIAN_POINT ( 'NONE',  ( 33.87825334127423815, -5.339472581715918764, -1.692052827146944605 ) ) ;
#19500=CARTESIAN_POINT ( 'NONE',  ( 24.39586660158147779, 3.158670939509748976, -3.293463392983651872 ) ) ;
#19502=CARTESIAN_POINT ( 'NONE',  ( -69.92837670882107659, -20.78299143688747819, 9.949874371066202983 ) ) ;
#19505=DIRECTION ( 'NONE',  ( -0.9616058754224561245, 0.2744342186262705430, 0.000000000000000000 ) ) ;
#19506=CARTESIAN_POINT ( 'NONE',  ( -73.12711914256941270, 0.2882157670163680852, -9.814792072719024318 ) ) ;
#19508=CARTESIAN_POINT ( 'NONE',  ( -2.697268050091675118E-17, 3.729367930467589076, -6.000000000000000000 ) ) ;
#19510=CARTESIAN_POINT ( 'NONE',  ( 87.32347380307142259, -1.421525632644524251, -4.720772940814831564 ) ) ;
#19515=CARTESIAN_POINT ( 'NONE',  ( 14.91179222114675085, 11.91032444678283575, -2.533743837804387056 ) ) ;
#19519=CARTESIAN_POINT ( 'NONE',  ( 37.04629652946467644, -2.800754724101123472, 5.988368560126969165 ) ) ;
#19522=CARTESIAN_POINT ( 'NONE',  ( 87.43837438447430088, 0.1427924124619655843, -4.444214939316114332 ) ) ;
#19527=CARTESIAN_POINT ( 'NONE',  ( -62.92837670882106238, -23.80776546975053520, 6.000000000000000000 ) ) ;
#19529=CARTESIAN_POINT ( 'NONE',  ( 21.71185578408363881, 6.328645931448866335, 3.192210964217056191 ) ) ;
#19538=CARTESIAN_POINT ( 'NONE',  ( 22.99368205116111241, 2.291004117675890850, 4.722746232393920884 ) ) ;
#19554=CARTESIAN_POINT ( 'NONE',  ( 22.60213147365925934, 3.631766662821214187, -3.957887780529531163 ) ) ;
#19558=CARTESIAN_POINT ( 'NONE',  ( 21.85643539959774628, 5.695295784951009743, -9.764639101464164028 ) ) ;
#19559=CARTESIAN_POINT ( 'NONE',  ( 21.88804895127840311, 3.976982562632499274, 2.124131737554133537 ) ) ;
#19562=CARTESIAN_POINT ( 'NONE',  ( 87.20660408302002509, 0.2574974038930863407, -5.635807106906071340 ) ) ;
#19565=CARTESIAN_POINT ( 'NONE',  ( 15.53358838639597650, -3.613270961124078973, 2.630790167588612949 ) ) ;
#19566=CARTESIAN_POINT ( 'NONE',  ( 37.02143117275709727, -2.763783248133810044, 5.984487719841893316 ) ) ;
#19568=CARTESIAN_POINT ( 'NONE',  ( 36.63324149830979337, -3.079498397735149329, -5.923901332741634995 ) ) ;
#19576=CARTESIAN_POINT ( 'NONE',  ( 32.88849341148151240, -3.409024750725885955, 5.320318896896437444 ) ) ;
#19578=EDGE_LOOP ( 'NONE', ( #28395, #39374, #6189, #12247 ) ) ;
#19579=CARTESIAN_POINT ( 'NONE',  ( 25.73329116135044003, 2.636594892696300541, 3.521394832687038789 ) ) ;
#19583=FACE_OUTER_BOUND ( 'NONE', #18546, .T. ) ;
#19584=CARTESIAN_POINT ( 'NONE',  ( 86.00054146471580907, 0.2529338399765344580, 5.999804812770356932 ) ) ;
#19607=CARTESIAN_POINT ( 'NONE',  ( 86.80434382515846892, 0.8549656295913086179, -5.002690157204635391 ) ) ;
#19608=CARTESIAN_POINT ( 'NONE',  ( 29.92651255597534288, -3.613225851372795727, -4.302012675596341928 ) ) ;
#19610=CARTESIAN_POINT ( 'NONE',  ( 33.89725028478159174, -5.465908938576614418, 0.4877600842561391481 ) ) ;
#19611=CARTESIAN_POINT ( 'NONE',  ( 11.29080664838499182, -35.94265729135299381, 6.000000000000000000 ) ) ;
#19615=CARTESIAN_POINT ( 'NONE',  ( 36.46007995281161129, -3.391394755346535117, -5.869938052945382623 ) ) ;
#19622=CARTESIAN_POINT ( 'NONE',  ( 22.03648680630582746, -11.51106657129999356, -2.500000000000000000 ) ) ;
#19627=VECTOR ( 'NONE', #28520, 1000.000000000000000 ) ;
#19633=CARTESIAN_POINT ( 'NONE',  ( 24.36285579537860357, 2.875202204253215044, 3.793786480169491604 ) ) ;
#19643=ORIENTED_EDGE ( 'NONE', *, *, #38488, .T. ) ;
#19645=CARTESIAN_POINT ( 'NONE',  ( 21.79003266261817373, 0.2242721076120573753, 8.362678294596348039 ) ) ;
#19648=( BOUNDED_SURFACE ( )  B_SPLINE_SURFACE ( 3, 2, ( 
 ( #29315, #4606, #29710 ),
 ( #16537, #17135, #920 ),
 ( #22945, #7279, #23541 ),
 ( #19843, #20432, #15072 ),
 ( #24130, #30529, #29909 ),
 ( #2338, #11157, #36695 ),
 ( #14455, #24542, #39367 ),
 ( #30324, #21059, #2132 ),
 ( #27222, #33631, #40185 ),
 ( #8679, #37099, #27628 ),
 ( #39785, #8476, #5407 ),
 ( #20839, #33011, #5002 ),
 ( #8268, #33833, #14650 ),
 ( #17946, #23921, #14858 ),
 ( #4800, #2546, #17331 ),
 ( #30742, #23728, #1724 ),
 ( #14254, #36294, #27026 ),
 ( #11557, #26826, #27428 ) ),
 .UNSPECIFIED., .F., .F., .T. ) 
 B_SPLINE_SURFACE_WITH_KNOTS ( ( 4, 2, 2, 2, 2, 2, 2, 2, 4 ),
 ( 3, 3 ),
 ( -3.897706810085388440E-17, 9.268508998302566707E-05, 0.0001853701799660903112, 0.0003707403599322195995, 0.0005561105398983489691, 0.0006487956298814135997, 0.0006951381748729458607, 0.0007183094473687120455, 0.0007414807198644782302 ),
 ( 0.000000000000000000, 1.000000000000000000 ),
 .UNSPECIFIED. ) 
 GEOMETRIC_REPRESENTATION_ITEM ( )  RATIONAL_B_SPLINE_SURFACE ( (
 ( 1.000000000000000000, 0.9970051441236879031, 1.000000000000000000),
 ( 1.000000000000000000, 0.9970378225561581376, 1.000000000000000000),
 ( 1.000000000000000000, 0.9972394906898559563, 1.000000000000000000),
 ( 1.000000000000000000, 0.9976321421133419465, 1.000000000000000000),
 ( 1.000000000000000000, 0.9978422869890333224, 1.000000000000000000),
 ( 1.000000000000000000, 0.9984523809614584966, 1.000000000000000000),
 ( 1.000000000000000000, 0.9988360290112493489, 1.000000000000000000),
 ( 1.000000000000000000, 0.9994464665223562472, 1.000000000000000000),
 ( 1.000000000000000000, 0.9996736563026237254, 1.000000000000000000),
 ( 1.000000000000000000, 0.9998843893650831705, 1.000000000000000000),
 ( 1.000000000000000000, 0.9999333845000230037, 1.000000000000000000),
 ( 1.000000000000000000, 0.9999776760172924828, 1.000000000000000000),
 ( 1.000000000000000000, 0.9999875764423735713, 1.000000000000000000),
 ( 1.000000000000000000, 0.9999962119944856287, 1.000000000000000000),
 ( 1.000000000000000000, 0.9999980683705610440, 1.000000000000000000),
 ( 1.000000000000000000, 0.9999999292169973186, 1.000000000000000000),
 ( 1.000000000000000000, 0.9999996798682928567, 1.000000000000000000),
 ( 1.000000000000000000, 0.9999997033893416321, 1.000000000000000000) ) ) 
 REPRESENTATION_ITEM ( '' )  SURFACE ( )  );
#19654=CARTESIAN_POINT ( 'NONE',  ( 24.33615536228354514, 0.1518143133650739496, -6.924920736309362113 ) ) ;
#19657=CARTESIAN_POINT ( 'NONE',  ( -77.36554191947220716, -6.175991868022603803, 7.662488528983584679 ) ) ;
#19658=CARTESIAN_POINT ( 'NONE',  ( 24.11813158041969984, 0.4652598558864985967, -5.100767782630346581 ) ) ;
#19662=CARTESIAN_POINT ( 'NONE',  ( 35.83212964707659154, -3.727973511289250030, -5.624487930365151378 ) ) ;
#19663=CARTESIAN_POINT ( 'NONE',  ( 30.48436916548869391, -3.145932567401911850, -4.957248004276928910 ) ) ;
#19665=CARTESIAN_POINT ( 'NONE',  ( 16.29348332828302048, 9.833248505471146927, 2.749390151398705573 ) ) ;
#19670=CARTESIAN_POINT ( 'NONE',  ( 24.25735127829256399, 1.467485774236111373, -4.660622497933993635 ) ) ;
#19671=CARTESIAN_POINT ( 'NONE',  ( 33.56666239001700092, -0.3391249266082498326, -5.044679946851483798 ) ) ;
#19677=EDGE_CURVE ( 'NONE', #34818, #5866, #18618, .T. ) ;
#19679=CARTESIAN_POINT ( 'NONE',  ( 86.04767080185138184, 0.5164224212623146348, 6.001289606117265585 ) ) ;
#19682=CARTESIAN_POINT ( 'NONE',  ( -76.51636512074169616, 9.210593808855891851, -9.784462033820121363 ) ) ;
#19693=CARTESIAN_POINT ( 'NONE',  ( 24.21576457907998048, 2.660053767493973265, 3.985853741681663287 ) ) ;
#19697=CARTESIAN_POINT ( 'NONE',  ( 21.85643539959780313, -10.31987362501297056, 12.61309593674697993 ) ) ;
#19698=CARTESIAN_POINT ( 'NONE',  ( 23.42712317297381119, 3.762989615831232371, -3.173731162736729061 ) ) ;
#19699=ORIENTED_EDGE ( 'NONE', *, *, #30094, .T. ) ;
#19704=CARTESIAN_POINT ( 'NONE',  ( -72.84083785044238368, 2.619656753172959540, -9.875546965173446878 ) ) ;
#19706=DIRECTION ( 'NONE',  ( 0.000000000000000000, -0.000000000000000000, -1.000000000000000000 ) ) ;
#19708=CARTESIAN_POINT ( 'NONE',  ( 85.28844081106248609, 1.468752784057639094, 5.439171570854275828 ) ) ;
#19712=EDGE_CURVE ( 'NONE', #2537, #18532, #19190, .T. ) ;
#19718=DIRECTION ( 'NONE',  ( 0.000000000000000000, 0.000000000000000000, -1.000000000000000000 ) ) ;
#19721=CARTESIAN_POINT ( 'NONE',  ( 35.78615804230325637, -3.164549726578430811, 5.791693472641034290 ) ) ;
#19722=EDGE_CURVE ( 'NONE', #14346, #36231, #40045, .T. ) ;
#19724=CARTESIAN_POINT ( 'NONE',  ( 85.06715496341631422, 2.806258611057371066, -0.4571093354346482673 ) ) ;
#19725=CIRCLE ( 'NONE', #5939, 21.28220113893567245 ) ;
#19732=CARTESIAN_POINT ( 'NONE',  ( -75.07873864619844539, -4.847503269688606231, 9.099517967925462969 ) ) ;
#19737=CARTESIAN_POINT ( 'NONE',  ( 24.25000701045975404, 1.480808258834079183, 4.656548141442817368 ) ) ;
#19742=CARTESIAN_POINT ( 'NONE',  ( 85.14854983093479746, 2.714832032627191971, 0.8233776845609513950 ) ) ;
#19746=CARTESIAN_POINT ( 'NONE',  ( 23.42844204553037102, 3.310894996220114184, -3.716253240727860785 ) ) ;
#19747=EDGE_LOOP ( 'NONE', ( #15676, #30934, #22501, #8250 ) ) ;
#19750=CARTESIAN_POINT ( 'NONE',  ( 21.85643539959775694, 2.837881715527333260, -11.82040581148825353 ) ) ;
#19752=CARTESIAN_POINT ( 'NONE',  ( 18.14195397311783964, 13.68994309133305975, 3.806916816956696259 ) ) ;
#19755=CARTESIAN_POINT ( 'NONE',  ( 86.86561140461988373, 0.2703162379016064154, -5.930766725306959586 ) ) ;
#19758=CARTESIAN_POINT ( 'NONE',  ( 15.55097496540485302, -3.641916182646045996, 2.633503763738948233 ) ) ;
#19760=CARTESIAN_POINT ( 'NONE',  ( 30.51576791750731488, -0.1387227150358968375, -4.969121628799780588 ) ) ;
#19762=CARTESIAN_POINT ( 'NONE',  ( 84.09810771740265523, 3.020293266994594994, 0.2534269013960862016 ) ) ;
#19763=CARTESIAN_POINT ( 'NONE',  ( -73.56224669261729332, -0.9187133512700828009, 10.86667021741267369 ) ) ;
#19768=ADVANCED_FACE ( 'NONE', ( #932 ), #23150, .F. ) ;
#19772=CARTESIAN_POINT ( 'NONE',  ( 29.51363873213982103, -3.424872186366097360, 4.784073270833150815 ) ) ;
#19775=CARTESIAN_POINT ( 'NONE',  ( 20.91912723174414523, 4.580704557862071979, 2.655339189496692232 ) ) ;
#19778=CARTESIAN_POINT ( 'NONE',  ( 87.48590409800530665, -1.976339587909113016, 3.594369327898899513 ) ) ;
#19789=DIRECTION ( 'NONE',  ( -0.000000000000000000, -0.000000000000000000, 1.000000000000000000 ) ) ;
#19801=CARTESIAN_POINT ( 'NONE',  ( 24.20448666664697868, 2.666065671757310795, -3.984093550689149055 ) ) ;
#19805=CARTESIAN_POINT ( 'NONE',  ( 30.10774373291980766, -4.462292185204852046, -2.031966353365944666 ) ) ;
#19807=LINE ( 'NONE', #1292, #37332 ) ;
#19811=CARTESIAN_POINT ( 'NONE',  ( 36.29305064575918038, -2.016329881244163680, -5.862899224838821866 ) ) ;
#19812=DIRECTION ( 'NONE',  ( 0.000000000000000000, 1.000000000000000000, 0.000000000000000000 ) ) ;
#19816=CARTESIAN_POINT ( 'NONE',  ( 23.06591706423118637, -8.086835649431872497, -2.500000000000005773 ) ) ;
#19818=EDGE_CURVE ( 'NONE', #36134, #1678, #4222, .T. ) ;
#19821=CARTESIAN_POINT ( 'NONE',  ( 37.10281511974962854, -2.625417964323302211, 5.990186448831483546 ) ) ;
#19825=VERTEX_POINT ( 'NONE', #532 ) ;
#19828=CARTESIAN_POINT ( 'NONE',  ( 23.00813552179332788, 3.484112554442508003, 3.810651395707427724 ) ) ;
#19834=CARTESIAN_POINT ( 'NONE',  ( 21.71193631872560559, 6.329239510039562866, 3.192900200192605897 ) ) ;
#19835=FACE_OUTER_BOUND ( 'NONE', #33716, .T. ) ;
#19836=CARTESIAN_POINT ( 'NONE',  ( 16.86712048606784009, -3.293910290563445198, 2.810174632765468417 ) ) ;
#19839=CARTESIAN_POINT ( 'NONE',  ( 19.23826442257826841, -6.969287627455325485, -2.500000000000009326 ) ) ;
#19840=VERTEX_POINT ( 'NONE', #32230 ) ;
#19842=CARTESIAN_POINT ( 'NONE',  ( 21.98032544390349940, 0.2298825911022993052, 7.706387622467548937 ) ) ;
#19843=CARTESIAN_POINT ( 'NONE',  ( 14.62029201251024446, -4.585632647846321852, -2.500000000000095035 ) ) ;
#19845=ADVANCED_FACE ( 'NONE', ( #13067 ), #27552, .F. ) ;
#19848=CARTESIAN_POINT ( 'NONE',  ( 8.290806648384990041, -33.63722727088462250, -6.000000000000001776 ) ) ;
#19850=CARTESIAN_POINT ( 'NONE',  ( 23.92064240948634790, 4.179079982057642972, -0.5982227118658990372 ) ) ;
#19852=EDGE_LOOP ( 'NONE', ( #13517, #38850, #16383, #27673, #29733, #9429, #9792, #23033, #40144, #3727, #4033, #18911 ) ) ;
#19853=CARTESIAN_POINT ( 'NONE',  ( -80.19506747669507263, -6.650235582408308588, 3.780597760675498353 ) ) ;
#19857=CARTESIAN_POINT ( 'NONE',  ( 36.88765961127775483, -3.350445860750347560, -5.910858986277842675 ) ) ;
#19871=CARTESIAN_POINT ( 'NONE',  ( 84.36871573755720988, 2.689384369868815128, -2.914620128191189874 ) ) ;
#19873=ORIENTED_EDGE ( 'NONE', *, *, #5683, .T. ) ;
#19874=CARTESIAN_POINT ( 'NONE',  ( 26.55823958201730761, 1.660274760599077526, 4.322293138832669079 ) ) ;
#19879=CARTESIAN_POINT ( 'NONE',  ( 21.85643539959777115, -33.54387950140291963, 2.500000000000000000 ) ) ;
#19883=CARTESIAN_POINT ( 'NONE',  ( 33.89348300072561671, -5.437596492814196658, 0.9556765382706865486 ) ) ;
#19890=CARTESIAN_POINT ( 'NONE',  ( 21.85643539959779602, 6.788858854521340191, -12.70575755685024610 ) ) ;
#19896=CARTESIAN_POINT ( 'NONE',  ( 14.76364886281816702, -5.161460284205085181, -2.499999999999998668 ) ) ;
#19898=CARTESIAN_POINT ( 'NONE',  ( -72.17181076888959979, 5.281718996255664322, -9.923482759818879728 ) ) ;
#19908=CARTESIAN_POINT ( 'NONE',  ( 21.29222209659852538, 5.334569642440764703, -3.529564231148301090 ) ) ;
#19914=CARTESIAN_POINT ( 'NONE',  ( 33.46257264326497705, -3.087412692527623737, 5.429041774995859271 ) ) ;
#19917=CARTESIAN_POINT ( 'NONE',  ( 85.06055580697953644, 2.762169973306998205, -2.784126402610546780 ) ) ;
#19921=CARTESIAN_POINT ( 'NONE',  ( 88.07494619931479463, -0.5722352634876846089, -2.741974656063581595 ) ) ;
#19927=CARTESIAN_POINT ( 'NONE',  ( 20.40287464304303100, 10.75613383955523616, -2.500000000000000000 ) ) ;
#19929=CARTESIAN_POINT ( 'NONE',  ( 23.04464813533367007, 1.997931949779890193, 4.910482787407937089 ) ) ;
#19935=CARTESIAN_POINT ( 'NONE',  ( 85.36928332665556240, 2.466893693589887082, 2.452742180977539821 ) ) ;
#19939=CARTESIAN_POINT ( 'NONE',  ( 22.73709572080239028, 4.093838367243191279, -3.481645627490313810 ) ) ;
#19943=CARTESIAN_POINT ( 'NONE',  ( 21.85643539959777115, 3.923092093126210322, -11.21220060410217734 ) ) ;
#19944=CARTESIAN_POINT ( 'NONE',  ( 21.75859177104565489, 5.853256811527690395, 2.474032597377961856E-12 ) ) ;
#19947=CARTESIAN_POINT ( 'NONE',  ( 87.20660408302002509, 0.2574974038930863407, -5.635807106906071340 ) ) ;
#19949=CARTESIAN_POINT ( 'NONE',  ( 29.25459127448231911, -9.786627965178412936, 2.499999999999995115 ) ) ;
#19951=CARTESIAN_POINT ( 'NONE',  ( 14.83772866404364166, -6.147680757941134999, 2.522184428484549823 ) ) ;
#19953=CARTESIAN_POINT ( 'NONE',  ( 17.01156838727278497, -3.085974904712485589, -2.861464691806836491 ) ) ;
#19954=CARTESIAN_POINT ( 'NONE',  ( 36.64531717283165335, -2.463042617044940652, -5.925786033801909269 ) ) ;
#19962=VECTOR ( 'NONE', #21096, 1000.000000000000000 ) ;
#19966=CARTESIAN_POINT ( 'NONE',  ( 34.14231943393395596, -3.847370251764138604, 5.235623355854905014 ) ) ;
#19969=CARTESIAN_POINT ( 'NONE',  ( 87.46548545408306552, -1.950952776479559558, 3.668367378035980675 ) ) ;
#19974=ORIENTED_EDGE ( 'NONE', *, *, #40454, .T. ) ;
#19978=CARTESIAN_POINT ( 'NONE',  ( 24.37212372168754726, 2.938878590626362808, 3.724495982890795975 ) ) ;
#19991=DIRECTION ( 'NONE',  ( -1.000000000000000000, 0.000000000000000000, 0.000000000000000000 ) ) ;
#19992=VECTOR ( 'NONE', #15840, 1000.000000000000000 ) ;
#19998=CARTESIAN_POINT ( 'NONE',  ( 33.87650332550894916, -5.319205609767368337, 2.014658837789633949 ) ) ;
#20000=CARTESIAN_POINT ( 'NONE',  ( -69.92837670882107659, -20.78299143688747819, 9.949874371066202983 ) ) ;
#20005=CARTESIAN_POINT ( 'NONE',  ( 27.67015415078466845, 1.632010242488362239, -4.348995382990432645 ) ) ;
#20011=CARTESIAN_POINT ( 'NONE',  ( 22.03819786145127324, -11.49891975756862905, -2.500000000000000444 ) ) ;
#20014=CARTESIAN_POINT ( 'NONE',  ( 35.61922268405216130, -1.517313264732231826, 5.701820347972824443 ) ) ;
#20019=EDGE_LOOP ( 'NONE', ( #17314, #38105, #18239, #35835, #17929 ) ) ;
#20023=CARTESIAN_POINT ( 'NONE',  ( 84.68233004218363646, 2.293814140821111014, -4.096401400287722261 ) ) ;
#20028=ORIENTED_EDGE ( 'NONE', *, *, #39934, .T. ) ;
#20029=CARTESIAN_POINT ( 'NONE',  ( 21.71407365845957216, 6.310579482064422763, 3.199499156096070163 ) ) ;
#20031=AXIS2_PLACEMENT_3D ( 'NONE', #50, #31948, #22877 ) ;
#20037=CARTESIAN_POINT ( 'NONE',  ( 24.74144660671096929, 0.6009092516020706487, 4.778017222739464387 ) ) ;
#20049=CARTESIAN_POINT ( 'NONE',  ( 25.40259394636483137, -3.746514978370850457, -4.387842602613081233 ) ) ;
#20052=CARTESIAN_POINT ( 'NONE',  ( -76.75188302604665580, -5.916639119592683294, 8.138648572045363849 ) ) ;
#20053=CARTESIAN_POINT ( 'NONE',  ( 23.59259267867648191, 0.4263748119163079386, -5.522675619391560708 ) ) ;
#20055=AXIS2_PLACEMENT_3D ( 'NONE', #1851, #17657, #21180 ) ;
#20057=CARTESIAN_POINT ( 'NONE',  ( 21.79480611247224786, 6.321165038070731157, 2.729589078629726551 ) ) ;
#20059=CARTESIAN_POINT ( 'NONE',  ( 36.68492070182102083, -1.915863264778755237, -5.803701069252491962 ) ) ;
#20061=VECTOR ( 'NONE', #11820, 1000.000000000000000 ) ;
#20066=AXIS2_PLACEMENT_3D ( 'NONE', #35046, #25964, #9903 ) ;
#20069=( BOUNDED_SURFACE ( )  B_SPLINE_SURFACE ( 3, 2, ( 
 ( #31314, #431, #12559 ),
 ( #9462, #9677, #16257 ),
 ( #6399, #22856, #12971 ),
 ( #38279, #28829, #220 ) ),
 .UNSPECIFIED., .F., .F., .T. ) 
 B_SPLINE_SURFACE_WITH_KNOTS ( ( 4, 4 ),
 ( 3, 3 ),
 ( 0.000000000000000000, 0.0008754244208269470464 ),
 ( 0.000000000000000000, 1.000000000000000000 ),
 .UNSPECIFIED. ) 
 GEOMETRIC_REPRESENTATION_ITEM ( )  RATIONAL_B_SPLINE_SURFACE ( (
 ( 1.000000000000000000, 0.9970051441236887912, 1.000000000000000000),
 ( 1.000000000000000000, 0.9987001331027990370, 1.000000000000000000),
 ( 1.000000000000000000, 0.9999578578055167144, 1.000000000000000000),
 ( 1.000000000000000000, 1.000000000000000000, 1.000000000000000000) ) ) 
 REPRESENTATION_ITEM ( '' )  SURFACE ( )  );
#20072=CARTESIAN_POINT ( 'NONE',  ( 84.85978623402763787, 2.253055191119315737, -4.296636491436513161 ) ) ;
#20073=B_SPLINE_SURFACE_WITH_KNOTS ( 'NONE', 5, 3, ( 
 ( #38319, #22704, #35272, #19607, #13619, #26194, #3978, #29074, #38726, #35668, #39534, #17907, #29871, #39948, #30489, #20801, #2295, #33394, #4963, #20591, #10923, #26987, #39743, #14419, #11315, #39126, #11724, #14821, #23881, #33176, #36657, #4759, #11522, #36256, #1897, #30280, #29669, #32974, #8436, #30082, #17293, #36455, #39331, #8230, #14015, #35867, #27387, #7645 ),
 ( #5166, #20194, #17702, #14217, #2095, #32780, #1687, #14611, #36066, #23499, #27183, #24089, #26792, #21018, #20392, #33595, #11121, #4569, #5369, #23690, #17096, #1481, #26587, #8033, #7844, #17489, #24715, #21633, #37462, #33791, #37658, #18947, #34214, #217, #2919, #27790, #3336, #30704, #18733, #24926, #5984, #9460, #31107, #9258, #15853, #15440, #12556, #28410 ),
 ( #28000, #40543, #21838, #15652, #18523, #2510, #31312, #3135, #34415, #12354, #6188, #22046, #28198, #27595, #31512, #28, #25128, #21220, #24506, #34623, #30908, #37058, #6396, #24299, #36860, #8645, #11930, #5571, #18110, #15034, #37263, #40148, #8846, #21431, #34005, #5779, #18317, #2716, #15237, #40345, #12140, #9056, #1040, #12757, #22455, #32138, #31714, #9674 ),
 ( #19947, #10475, #832, #3938, #29029, #25336, #35225, #16847, #37870, #3530, #22259, #429, #16054, #35024, #633, #35426, #10276, #28625, #34827, #38079, #13174, #6603, #38678, #25734, #19148, #6798, #12969, #4326, #25535, #9881, #19352, #13363, #7393, #16455, #25938, #31924, #22657, #3732, #23056, #38277, #22854, #28827, #32526, #7195, #10073, #6997, #13572, #19562 ),
 ( #38472, #26144, #19755, #32333, #16642, #29227, #35621, #36406, #11265, #8386, #39685, #30027, #33125, #17437, #17854, #23638, #5320, #1243, #32728, #13779, #29623, #20148, #10872, #29818, #23829, #39478, #4524, #10671, #26538, #1630, #23252, #27134, #14169, #7596, #23448, #17044, #33544, #1437, #35818, #8177, #20343, #20749, #26347, #36013, #5114, #13970, #39073, #17650 ),
 ( #36205, #7791, #30231, #32922, #38880, #2045, #4713, #14559, #17246, #11469, #26741, #4905, #24037, #39280, #11068, #14365, #7984, #36608, #20963, #20540, #1842, #26933, #33953, #9408, #36810, #24874, #31057, #12086, #15600, #37212, #2868, #21996, #21585, #18679, #34573, #37612, #9005, #34167, #5933, #15391, #21789, #24660, #8595, #37413, #9209, #27947, #18472, #40489 ),
 ( #5728, #12301, #21173, #6347, #12507, #30435, #24453, #8792, #34367, #2245, #37010, #6137, #30651, #33738, #31264, #3081, #21374, #28152, #14984, #40706, #40097, #14766, #25082, #18266, #27338, #39898, #11672, #30858, #24246, #5518, #2665, #27743, #18060, #2463, #27544, #11878, #40296, #15184, #38227, #22407, #38633, #25286, #13313, #19510, #586, #4083, #25684, #32085 ),
 ( #7148, #23007, #26095, #10024, #22607, #35175, #3890, #10226, #13125, #37817, #25886, #38425, #16405, #6948, #28979, #16597, #22809, #22209, #13524, #783, #35379, #15809, #19099, #19708, #25483, #31668, #32283, #10432, #29179, #988, #6554, #28779, #35574, #18897, #19302, #31464, #28363, #3287, #176, #12712, #381, #9622, #34776, #3484, #16009, #28574, #12917, #38029 ) ),
 .UNSPECIFIED., .F., .T., .F.,
 ( 6, 2, 6 ),
 ( 4, 1, 1, 1, 1, 1, 1, 1, 1, 1, 1, 1, 1, 1, 1, 1, 1, 1, 1, 1, 1, 1, 1, 1, 1, 1, 1, 1, 1, 1, 1, 1, 1, 1, 1, 1, 1, 1, 1, 1, 1, 1, 1, 1, 1, 4 ),
 ( 0.000000000000000000, 0.5000000000000000000, 1.000000000000000000 ),
 ( 0.02319993227479018663, 0.02338707809474536645, 0.02357422391470053238, 0.02376136973465571220, 0.02401089749459594039, 0.02432280719452123083, 0.02469709883443158005, 0.02507139047434192580, 0.02557044599422238565, 0.02619426539407297347, 0.02694284867389366844, 0.02769143195371436342, 0.02844001523353506186, 0.02918859851335575684, 0.02993718179317645181, 0.03068576507299715025, 0.03143434835281785217, 0.03218293163263854367, 0.03293151491245924212, 0.03355533431230981606, 0.03405438983219027937, 0.03442868147210063207, 0.03480297311201098476, 0.03511488281193627520, 0.03536441057187650339, 0.03555155639183167626, 0.03573870221178684914, 0.03598822997172709121, 0.03630013967165238165, 0.03667443131156272740, 0.03704872295147307315, 0.03754777847135353647, 0.03817159787120411735, 0.03892018115102481579, 0.03966876443084551424, 0.04041734771066620574, 0.04141545875042713931, 0.04241356979018806594, 0.04341168082994899952, 0.04416026410976969102, 0.04490884738959038947, 0.04553266678944096341, 0.04603172230932142672, 0.04640601394923177248, 0.04678030558914212517, 0.04715459722905247786 ),
 .UNSPECIFIED. ) ;
#20074=CARTESIAN_POINT ( 'NONE',  ( -80.26960040814950048, 10.48563383736161114, -5.954513432128944572 ) ) ;
#20080=VECTOR ( 'NONE', #24045, 1000.000000000000000 ) ;
#20084=CARTESIAN_POINT ( 'NONE',  ( 36.96348058853109819, -2.193283099190300511, 5.898309123131363130 ) ) ;
#20086=CARTESIAN_POINT ( 'NONE',  ( -17.27251170661583402, -8.656638842136340273, 6.000000000000000000 ) ) ;
#20088=EDGE_CURVE ( 'NONE', #37655, #5466, #24580, .T. ) ;
#20091=CARTESIAN_POINT ( 'NONE',  ( 33.79284613923667990, -4.878148420886379455, -3.390896070728523615 ) ) ;
#20095=CARTESIAN_POINT ( 'NONE',  ( -72.17666250106589132, -0.4381958982661475765, -9.922884124630229508 ) ) ;
#20097=CARTESIAN_POINT ( 'NONE',  ( -17.69482985384421880, -29.56993018339339940, 6.000000000000000000 ) ) ;
#20109=CARTESIAN_POINT ( 'NONE',  ( 35.86903479493524571, -2.086569765857306358, 5.804628394271051484 ) ) ;
#20110=EDGE_CURVE ( 'NONE', #6415, #16350, #21934, .T. ) ;
#20111=AXIS2_PLACEMENT_3D ( 'NONE', #37313, #31156, #28462 ) ;
#20113=CARTESIAN_POINT ( 'NONE',  ( 84.82990711808488982, 3.023024660489734394, 1.086629044751433293 ) ) ;
#20119=CARTESIAN_POINT ( 'NONE',  ( -80.93510526298557295, 11.45401881227207497, 0.2075866020563601477 ) ) ;
#20120=CARTESIAN_POINT ( 'NONE',  ( 24.86584501937821301, -5.834624453299285030, -2.864450365913323360 ) ) ;
#20121=ORIENTED_EDGE ( 'NONE', *, *, #12229, .T. ) ;
#20127=CARTESIAN_POINT ( 'NONE',  ( -17.27251170661583402, -8.656638842136340273, 6.000000000000000000 ) ) ;
#20129=CARTESIAN_POINT ( 'NONE',  ( 24.10439548121549436, 0.6331765145075038959, 5.082944852415793413 ) ) ;
#20134=CARTESIAN_POINT ( 'NONE',  ( 63.05383694556373797, -7.271989087314214117, 6.000000000000000000 ) ) ;
#20135=CARTESIAN_POINT ( 'NONE',  ( 85.76501473881677384, 2.022389388904533902, 3.835323685118464443 ) ) ;
#20139=CARTESIAN_POINT ( 'NONE',  ( 22.68981863355961082, 4.343343972393600261, -3.284089849446835352 ) ) ;
#20143=CARTESIAN_POINT ( 'NONE',  ( 22.75155763331752112, -5.137713618528696458, -6.528071535057289765 ) ) ;
#20144=CARTESIAN_POINT ( 'NONE',  ( 21.83106932671411471, 5.061056560965798035, 3.908462188293328587 ) ) ;
#20145=CARTESIAN_POINT ( 'NONE',  ( 20.41154445963425701, 10.73873515079988294, 2.500000000000000444 ) ) ;
#20148=CARTESIAN_POINT ( 'NONE',  ( 85.36258410344761671, 2.204690851838579047, 4.549306268726941660 ) ) ;
#20152=CARTESIAN_POINT ( 'NONE',  ( 23.84450253662037866, -2.668400562688592714, 3.927909320949413807 ) ) ;
#20154=CARTESIAN_POINT ( 'NONE',  ( 35.78593763082197654, -3.161148606490439050, -5.791659072098707561 ) ) ;
#20156=CARTESIAN_POINT ( 'NONE',  ( 84.48228160770625550, 2.547494559575964157, -3.385513399219323372 ) ) ;
#20164=CARTESIAN_POINT ( 'NONE',  ( 36.49352434727311589, -3.559963790946740758, 5.796433071289773586 ) ) ;
#20165=CARTESIAN_POINT ( 'NONE',  ( 16.40512227804392609, -3.237279488405499617, 2.766814109507098163 ) ) ;
#20170=CARTESIAN_POINT ( 'NONE',  ( 86.05032028231427432, 0.1565332958781914807, 6.000000348367978908 ) ) ;
#20172=ORIENTED_EDGE ( 'NONE', *, *, #28208, .T. ) ;
#20174=DIRECTION ( 'NONE',  ( -0.000000000000000000, -1.000000000000000000, -0.000000000000000000 ) ) ;
#20175=EDGE_LOOP ( 'NONE', ( #17856, #25144, #37903, #25853, #2038 ) ) ;
#20180=CARTESIAN_POINT ( 'NONE',  ( 24.25095726714989297, 3.112089687977687369, 3.515329813937853043 ) ) ;
#20185=DIRECTION ( 'NONE',  ( 0.000000000000000000, 0.000000000000000000, 1.000000000000000000 ) ) ;
#20187=CARTESIAN_POINT ( 'NONE',  ( 23.19159090904956599, 2.549548122309488907, -4.431069449850736142 ) ) ;
#20189=CARTESIAN_POINT ( 'NONE',  ( 16.13271431945180723, 15.26109421794535059, -1.496401833041691720 ) ) ;
#20190=CARTESIAN_POINT ( 'NONE',  ( 24.38023270008697097, 2.574825574644751924, -4.011522969641340808 ) ) ;
#20192=DIRECTION ( 'NONE',  ( -0.000000000000000000, -0.000000000000000000, -1.000000000000000000 ) ) ;
#20194=CARTESIAN_POINT ( 'NONE',  ( 87.05466826895010968, 0.5737893332097195875, -5.097061431219924721 ) ) ;
#20195=CARTESIAN_POINT ( 'NONE',  ( 31.96905077431594933, -4.633974458378385286, -3.035954366531696369 ) ) ;
#20200=AXIS2_PLACEMENT_3D ( 'NONE', #21099, #40225, #12007 ) ;
#20201=CARTESIAN_POINT ( 'NONE',  ( -81.33601108014657655, -5.640736238038894790, -3.433968290496116182 ) ) ;
#20204=CARTESIAN_POINT ( 'NONE',  ( 34.13174693812651839, -3.213397211757874850, -5.533482607768558381 ) ) ;
#20213=CARTESIAN_POINT ( 'NONE',  ( 36.84686803492319029, -3.231021363853832540, 5.943776631324515058 ) ) ;
#20220=CARTESIAN_POINT ( 'NONE',  ( 86.14847104707970971, -0.02438626603933686729, -5.973875385969918739 ) ) ;
#20228=CARTESIAN_POINT ( 'NONE',  ( 24.05520612681470993, 3.340626845478275264, 3.238600984571303520 ) ) ;
#20230=CARTESIAN_POINT ( 'NONE',  ( 20.42004053729723978, -3.555855083337302158, -2.499999999979800158 ) ) ;
#20233=CARTESIAN_POINT ( 'NONE',  ( 24.12423001070950690, 0.5003150286851053563, 5.094044111947246378 ) ) ;
#20234=FACE_OUTER_BOUND ( 'NONE', #24419, .T. ) ;
#20242=CARTESIAN_POINT ( 'NONE',  ( 28.93850508814251299, -1.888738275646064668, -5.863986819262115624 ) ) ;
#20245=CARTESIAN_POINT ( 'NONE',  ( -75.89283711940969113, -3.900305280487442516, 10.11395962696834872 ) ) ;
#20246=CARTESIAN_POINT ( 'NONE',  ( 24.74436007370645285, 0.5872009258416482913, -4.777575718694301088 ) ) ;
#20247=AXIS2_PLACEMENT_3D ( 'NONE', #25788, #13415, #25582 ) ;
#20250=CARTESIAN_POINT ( 'NONE',  ( 36.49292402375851196, -3.557488610187057532, -5.797583871770345176 ) ) ;
#20258=CARTESIAN_POINT ( 'NONE',  ( 21.53656876454488156, 7.496978015852163502, 2.849741189840151456 ) ) ;
#20264=ORIENTED_EDGE ( 'NONE', *, *, #10593, .T. ) ;
#20265=CARTESIAN_POINT ( 'NONE',  ( 84.32222422711384979, 2.914578286995431977, 1.930349914595605343 ) ) ;
#20269=DIRECTION ( 'NONE',  ( 0.9594800004753906153, 0.2817767355331954326, 0.000000000000000000 ) ) ;
#20275=CARTESIAN_POINT ( 'NONE',  ( 36.86034836333212894, -2.080661969557957125, 5.862916021703864722 ) ) ;
#20282=CARTESIAN_POINT ( 'NONE',  ( 21.85643539959777470, 9.109670159223330899, 10.09094178405049647 ) ) ;
#20286=CARTESIAN_POINT ( 'NONE',  ( 14.66162177708395653, -4.890547631111535232, 2.500000000000003109 ) ) ;
#20287=CARTESIAN_POINT ( 'NONE',  ( -75.52298870755240046, -5.187903949434842232, -8.883779244834281386 ) ) ;
#20297=CARTESIAN_POINT ( 'NONE',  ( -69.92837670882109080, -0.6508471542538479815, 9.949874371066202983 ) ) ;
#20299=CARTESIAN_POINT ( 'NONE',  ( 15.11713524669251107, 11.51833089347275774, -2.565792583180644293 ) ) ;
#20303=CARTESIAN_POINT ( 'NONE',  ( 36.99348654919808155, -2.718276929309134449, 5.980126285492262994 ) ) ;
#20306=CARTESIAN_POINT ( 'NONE',  ( 88.66415851257785619, -1.234066499448195131, -0.8261491842984883816 ) ) ;
#20307=EDGE_CURVE ( 'NONE', #18355, #10861, #36914, .T. ) ;
#20314=CARTESIAN_POINT ( 'NONE',  ( -79.58467717747977588, 11.50090110917795450, -5.024625831181132263 ) ) ;
#20323=CARTESIAN_POINT ( 'NONE',  ( 26.46424199157858226, 1.161643656104778488, 4.368481250744165933 ) ) ;
#20327=CARTESIAN_POINT ( 'NONE',  ( 91.69672933337632514, -4.640393979863029372, 6.000000000000001776 ) ) ;
#20332=CARTESIAN_POINT ( 'NONE',  ( 22.45719325378483333, 4.667233400556632716, -3.240875079928056568 ) ) ;
#20337=CARTESIAN_POINT ( 'NONE',  ( 22.73811350958456501, -4.924115162416450531, 6.814090253401713149 ) ) ;
#20338=CARTESIAN_POINT ( 'NONE',  ( 21.88804895128980021, 3.976982562626299345, -2.124131737561591127 ) ) ;
#20339=CARTESIAN_POINT ( 'NONE',  ( 16.50401484676293506, 9.937674364320209008, 2.500000000000111466 ) ) ;
#20343=CARTESIAN_POINT ( 'NONE',  ( 88.55280947256005675, -1.781472883390815110, -2.828200999223334566 ) ) ;
#20350=AXIS2_PLACEMENT_3D ( 'NONE', #19399, #28457, #16101 ) ;
#20351=CARTESIAN_POINT ( 'NONE',  ( 15.20539192819301633, -3.834574542907454475, -2.579567172824699828 ) ) ;
#20352=CARTESIAN_POINT ( 'NONE',  ( 36.42048812037058525, -3.112390500302440355, -5.890696022654337227 ) ) ;
#20354=CARTESIAN_POINT ( 'NONE',  ( 84.11387586591480670, 3.001218439285060047, 0.7410103870498383483 ) ) ;
#20355=CARTESIAN_POINT ( 'NONE',  ( 28.97886027966445610, -3.943940219105989353, -4.212134838613624588 ) ) ;
#20363=CARTESIAN_POINT ( 'NONE',  ( 36.88795034744942569, -3.350989778144811471, 5.910704712194680965 ) ) ;
#20365=CARTESIAN_POINT ( 'NONE',  ( 33.45832265597695709, -3.170157842402876014, 5.428378461693221801 ) ) ;
#20369=VERTEX_POINT ( 'NONE', #30758 ) ;
#20370=DIRECTION ( 'NONE',  ( -0.000000000000000000, 0.000000000000000000, 1.000000000000000000 ) ) ;
#20372=FACE_OUTER_BOUND ( 'NONE', #27718, .T. ) ;
#20374=CARTESIAN_POINT ( 'NONE',  ( 23.41989428638003901, 3.663279710099765385, 3.339762963842272558 ) ) ;
#20382=CARTESIAN_POINT ( 'NONE',  ( 18.07512871310107982, -2.861803080523624754, -3.027459002956025103 ) ) ;
#20383=CARTESIAN_POINT ( 'NONE',  ( 22.17093972887607478, 4.944255074668806316, -3.666709369531458318 ) ) ;
#20385=CARTESIAN_POINT ( 'NONE',  ( 23.78275041547294677, 2.837768902955438932, -3.973267813322601150 ) ) ;
#20387=FACE_OUTER_BOUND ( 'NONE', #19247, .T. ) ;
#20392=CARTESIAN_POINT ( 'NONE',  ( 85.06715496341631422, 2.806258611057371066, -0.4571093354346482673 ) ) ;
#20393=CARTESIAN_POINT ( 'NONE',  ( 29.23504802441905071, -0.3867851007456850065, 5.903809272860179647 ) ) ;
#20398=ADVANCED_FACE ( 'NONE', ( #33226 ), #18129, .F. ) ;
#20399=VECTOR ( 'NONE', #27903, 1000.000000000000000 ) ;
#20400=CARTESIAN_POINT ( 'NONE',  ( -75.26792576154856818, -3.339667509723542427, -10.38202132129838162 ) ) ;
#20403=CARTESIAN_POINT ( 'NONE',  ( 35.91729403143805399, -1.971504941976118364, -5.812160415281375947 ) ) ;
#20411=CARTESIAN_POINT ( 'NONE',  ( 35.35512691508515104, -3.679868515684123320, 5.594709844209936556 ) ) ;
#20418=CARTESIAN_POINT ( 'NONE',  ( 84.63963357584157166, 2.348532213434630034, -3.962486329823844855 ) ) ;
#20423=CARTESIAN_POINT ( 'NONE',  ( 21.99062700448786600, 5.603250647612985524, 3.098096661096519266 ) ) ;
#20425=CARTESIAN_POINT ( 'NONE',  ( 17.93053216672853623, -3.172292528566667880, 2.962912945814812016 ) ) ;
#20429=ORIENTED_EDGE ( 'NONE', *, *, #21440, .T. ) ;
#20431=CARTESIAN_POINT ( 'NONE',  ( 21.78052297937427539, 0.2074298702781548209, 8.415602729882047939 ) ) ;
#20432=CARTESIAN_POINT ( 'NONE',  ( 14.68921137941172717, -4.582243837930176866, -2.500000000000645262 ) ) ;
#20436=CARTESIAN_POINT ( 'NONE',  ( 34.83208863909184316, -3.836908605833605712, -5.388068011310329197 ) ) ;
#20441=EDGE_LOOP ( 'NONE', ( #25753, #33758, #24335, #3206, #36285, #37757 ) ) ;
#20442=CARTESIAN_POINT ( 'NONE',  ( 26.92542807167190944, 1.449366069832211279, 5.022290288739529984 ) ) ;
#20444=VERTEX_POINT ( 'NONE', #4327 ) ;
#20446=CARTESIAN_POINT ( 'NONE',  ( 21.97771708808641478, 0.2279745448313108547, -7.713837705808137990 ) ) ;
#20450=CARTESIAN_POINT ( 'NONE',  ( 36.44423773317367932, -1.734327446880802093, -5.731973242487343079 ) ) ;
#20451=DIRECTION ( 'NONE',  ( 1.000000000000000000, 1.165409145176970240E-16, 0.000000000000000000 ) ) ;
#20455=CARTESIAN_POINT ( 'NONE',  ( -4.890026461918814071, -8.228598103685714525E-16, 2.500000000000000000 ) ) ;
#20459=ORIENTED_EDGE ( 'NONE', *, *, #19124, .F. ) ;
#20464=CARTESIAN_POINT ( 'NONE',  ( 85.50109956362166486, 1.391598633704343113, -5.555888502831813902 ) ) ;
#20477=CARTESIAN_POINT ( 'NONE',  ( 33.45749450797183044, -3.829747548865578555, 5.093667367007288505 ) ) ;
#20478=EDGE_LOOP ( 'NONE', ( #31439, #2472, #19873, #24686, #35001, #12526, #6696, #372 ) ) ;
#20480=CARTESIAN_POINT ( 'NONE',  ( 15.36714913374379599, 11.54288649379375009, -2.576984622127588054 ) ) ;
#20482=CARTESIAN_POINT ( 'NONE',  ( 21.85643539959776760, 7.606201961588627825, -9.696886732879795190 ) ) ;
#20483=ORIENTED_EDGE ( 'NONE', *, *, #1888, .T. ) ;
#20484=CARTESIAN_POINT ( 'NONE',  ( -78.64259192827009315, 10.18527460795026940, 8.122084567072173300 ) ) ;
#20486=CARTESIAN_POINT ( 'NONE',  ( 14.75755952713405428, -4.578576653438560129, 2.509474734851031119 ) ) ;
#20489=CARTESIAN_POINT ( 'NONE',  ( -77.68233785927705526, 11.14461418698115125, -7.385558889936151949 ) ) ;
#20493=DIRECTION ( 'NONE',  ( 1.000000000000000000, 5.786005779812646808E-17, 0.000000000000000000 ) ) ;
#20501=CARTESIAN_POINT ( 'NONE',  ( 29.10269789033915444, 0.3625583223530568500, 4.748577875832423523 ) ) ;
#20503=CARTESIAN_POINT ( 'NONE',  ( 88.00102923632725549, -0.4892082223494365611, 4.076460784956554839 ) ) ;
#20505=CARTESIAN_POINT ( 'NONE',  ( 33.61415416546452661, -1.222806787721765431, -5.452699737548062586 ) ) ;
#20511=CARTESIAN_POINT ( 'NONE',  ( -17.27251170661583402, -8.656638842136340273, -6.000000000000000000 ) ) ;
#20514=ORIENTED_EDGE ( 'NONE', *, *, #20917, .T. ) ;
#20516=DIRECTION ( 'NONE',  ( 1.000000000000000000, 0.000000000000000000, 0.000000000000000000 ) ) ;
#20519=CARTESIAN_POINT ( 'NONE',  ( 26.31986897742153886, 1.795161610767696203, 4.274183613285711836 ) ) ;
#20527=CARTESIAN_POINT ( 'NONE',  ( 20.40287464734031531, 10.75613383782063970, 2.500000000000000000 ) ) ;
#20530=CARTESIAN_POINT ( 'NONE',  ( 21.94264646427332366, 5.218753353571838893, -3.467988951643584006 ) ) ;
#20532=CARTESIAN_POINT ( 'NONE',  ( -71.05911450274722085, 0.2170085631127137149, 6.000000000000031974 ) ) ;
#20534=CARTESIAN_POINT ( 'NONE',  ( 22.59998850301547790, -2.767621054697568361, -8.672491381162554802 ) ) ;
#20535=CARTESIAN_POINT ( 'NONE',  ( 21.90687190820672470, 4.042035482290116555, 2.582324705332042310E-12 ) ) ;
#20540=CARTESIAN_POINT ( 'NONE',  ( 84.71993633203089757, 2.603525311087758531, 3.468835001793752593 ) ) ;
#20544=CARTESIAN_POINT ( 'NONE',  ( -81.28678620492023299, -5.643235788115313234, 3.601638239438431199 ) ) ;
#20545=VERTEX_POINT ( 'NONE', #14560 ) ;
#20547=CARTESIAN_POINT ( 'NONE',  ( 14.96457931905862004, -6.087096554337192877, -2.529921590516770458 ) ) ;
#20548=CARTESIAN_POINT ( 'NONE',  ( 37.04325894773570838, -2.892658674496945359, -5.987894472034057891 ) ) ;
#20550=CARTESIAN_POINT ( 'NONE',  ( 22.37006418220767046, 0.3113197332365596481, -6.949876465829976979 ) ) ;
#20552=ORIENTED_EDGE ( 'NONE', *, *, #27458, .F. ) ;
#20553=CARTESIAN_POINT ( 'NONE',  ( 36.99180085876906787, -2.719722283181335687, 5.979863192732237209 ) ) ;
#20558=ORIENTED_EDGE ( 'NONE', *, *, #28540, .F. ) ;
#20559=CARTESIAN_POINT ( 'NONE',  ( 23.38648198192572636, 3.560659895774239025, 3.090151982821246701 ) ) ;
#20566=ORIENTED_EDGE ( 'NONE', *, *, #25915, .F. ) ;
#20570=ORIENTED_EDGE ( 'NONE', *, *, #8811, .F. ) ;
#20571=CARTESIAN_POINT ( 'NONE',  ( 21.76873572098353549, 5.759726986437556207, 3.412036244753165359 ) ) ;
#20577=LINE ( 'NONE', #8425, #4866 ) ;
#20578=LINE ( 'NONE', #23487, #13083 ) ;
#20582=CARTESIAN_POINT ( 'NONE',  ( 23.35463534039838862, 2.791180645285405326, -4.165794450420091444 ) ) ;
#20591=CARTESIAN_POINT ( 'NONE',  ( 85.52484820210342775, 2.292155841932438154, 3.149942891487422791 ) ) ;
#20592=CARTESIAN_POINT ( 'NONE',  ( 28.29523375420085074, 1.184784106264966219, 4.843441543353563361 ) ) ;
#20595=CARTESIAN_POINT ( 'NONE',  ( -73.82579051696868078, -1.443931487737144304, -10.81507813807952090 ) ) ;
#20600=CARTESIAN_POINT ( 'NONE',  ( 36.83726977465116903, -2.495954238268284886, -5.955744879707230766 ) ) ;
#20605=ORIENTED_EDGE ( 'NONE', *, *, #20967, .T. ) ;
#20606=CARTESIAN_POINT ( 'NONE',  ( 36.98479848736133846, -3.196135743401947504, 5.957709319320976249 ) ) ;
#20613=PLANE ( 'NONE',  #26580 ) ;
#20615=CARTESIAN_POINT ( 'NONE',  ( 85.24784528485831459, 1.525343023627036221, -5.365780758369952608 ) ) ;
#20622=CARTESIAN_POINT ( 'NONE',  ( 22.38585600833290812, 4.919343847142990001, 3.067110144847137843 ) ) ;
#20629=CARTESIAN_POINT ( 'NONE',  ( 21.96835430550240531, 0.2152734445375746875, 7.743662324112909445 ) ) ;
#20643=CARTESIAN_POINT ( 'NONE',  ( 30.10774373291980766, -4.462292185204852046, -2.031966353365944666 ) ) ;
#20647=CARTESIAN_POINT ( 'NONE',  ( -80.58170359628198298, -5.694316091744713759, 2.641081141217533457 ) ) ;
#20648=CARTESIAN_POINT ( 'NONE',  ( 27.43026218121176996, 0.9933767425001067686, -4.487545422184641808 ) ) ;
#20651=CARTESIAN_POINT ( 'NONE',  ( -4.890026461918812295, -8.951974136083761024, -6.000000000000000000 ) ) ;
#20653=CARTESIAN_POINT ( 'NONE',  ( -70.92837670882107659, -23.80776546975053520, 0.000000000000000000 ) ) ;
#20654=CARTESIAN_POINT ( 'NONE',  ( 33.45079413477735386, -3.771336813828650936, -5.158274019676979627 ) ) ;
#20655=CARTESIAN_POINT ( 'NONE',  ( 8.290806648384990041, 0.000000000000000000, -6.000000000000000000 ) ) ;
#20671=EDGE_CURVE ( 'NONE', #3377, #18355, #16089, .T. ) ;
#20678=CARTESIAN_POINT ( 'NONE',  ( 28.96720929824785884, -3.478576898793518613, 4.535785375070108927 ) ) ;
#20681=CARTESIAN_POINT ( 'NONE',  ( 18.62546884766482336, 11.49410693564760244, -2.500000000000005773 ) ) ;
#20689=CARTESIAN_POINT ( 'NONE',  ( 14.78132966858819408, 12.96967853271529592, -2.500000000000170530 ) ) ;
#20690=CARTESIAN_POINT ( 'NONE',  ( 17.06909365960932234, 14.52075518970088019, 2.500000000000000000 ) ) ;
#20691=CARTESIAN_POINT ( 'NONE',  ( 21.85643539959775339, -6.841675198209371977, -12.88699694080538549 ) ) ;
#20693=CARTESIAN_POINT ( 'NONE',  ( -81.74866560783399905, 10.46844104627007610, 1.587951278892896001 ) ) ;
#20696=CARTESIAN_POINT ( 'NONE',  ( 14.77552075046116542, -5.164772903469535770, 2.499999999999999556 ) ) ;
#20697=CARTESIAN_POINT ( 'NONE',  ( -76.45633091588946684, 10.63030786891022217, -8.341557872600688484 ) ) ;
#20703=DIRECTION ( 'NONE',  ( 0.000000000000000000, 1.000000000000000000, 0.000000000000000000 ) ) ;
#20704=CARTESIAN_POINT ( 'NONE',  ( 31.23832812783138735, -0.3864266517737607876, 5.081894624805558536 ) ) ;
#20706=CARTESIAN_POINT ( 'NONE',  ( 87.89830269644372152, -0.3738208970565018441, 3.381280162731604033 ) ) ;
#20710=CARTESIAN_POINT ( 'NONE',  ( 36.63374877720352174, -3.081660063073488942, 5.923980505881594638 ) ) ;
#20715=CARTESIAN_POINT ( 'NONE',  ( 85.02283808163620904, 2.856037436078923797, 1.058370034767218248 ) ) ;
#20730=CARTESIAN_POINT ( 'NONE',  ( 22.20022480168698920, 0.7782003466350271292, 6.794645230738167285 ) ) ;
#20735=CARTESIAN_POINT ( 'NONE',  ( 87.04213330793392345, 0.5878691963682337596, -6.000000000000000000 ) ) ;
#20739=CARTESIAN_POINT ( 'NONE',  ( 24.19406260597309100, 3.095814450226969772, -3.579834043910485430 ) ) ;
#20743=CARTESIAN_POINT ( 'NONE',  ( 22.40307219844260800, 2.196575021783337522, 8.487454310335619923 ) ) ;
#20745=CARTESIAN_POINT ( 'NONE',  ( -70.92837670882107659, -42.37473357531882812, 0.000000000000000000 ) ) ;
#20746=VERTEX_POINT ( 'NONE', #27339 ) ;
#20749=CARTESIAN_POINT ( 'NONE',  ( 88.36457133188896762, -1.562442635866588381, -3.606418352999261945 ) ) ;
#20754=CARTESIAN_POINT ( 'NONE',  ( 24.57140847954032736, 3.461729712179683727, -1.987756385015271743 ) ) ;
#20755=CARTESIAN_POINT ( 'NONE',  ( 14.65343585136595550, -5.052488753627910611, -2.492953801041927431 ) ) ;
#20756=CARTESIAN_POINT ( 'NONE',  ( 33.46279134528099064, -3.082547165344575735, -5.429075908734783518 ) ) ;
#20758=CARTESIAN_POINT ( 'NONE',  ( 26.54498440466941389, 1.102037382031719526, -4.373732055846625499 ) ) ;
#20759=CARTESIAN_POINT ( 'NONE',  ( 29.67375726883929588, -3.794827553840666834, -4.437594031920679249 ) ) ;
#20761=CARTESIAN_POINT ( 'NONE',  ( 36.44579707039719096, -2.356748688111148127, 5.894646096405367963 ) ) ;
#20763=ORIENTED_EDGE ( 'NONE', *, *, #1468, .T. ) ;
#20765=CARTESIAN_POINT ( 'NONE',  ( 36.68630651783246321, -1.913378901653658204, 5.802382176530635149 ) ) ;
#20772=EDGE_CURVE ( 'NONE', #7067, #4105, #10278, .T. ) ;
#20775=EDGE_CURVE ( 'NONE', #40623, #6564, #17379, .T. ) ;
#20780=ORIENTED_EDGE ( 'NONE', *, *, #30305, .F. ) ;
#20781=CARTESIAN_POINT ( 'NONE',  ( 14.72813520417063948, -4.877442212653578579, 2.502183594662707122 ) ) ;
#20785=CARTESIAN_POINT ( 'NONE',  ( 23.89669137058255899, 3.224793199604093275, 3.569543781043807762 ) ) ;
#20790=CARTESIAN_POINT ( 'NONE',  ( 18.11716068014149883, -2.855953840192153592, -3.034019107959646799 ) ) ;
#20793=CARTESIAN_POINT ( 'NONE',  ( 22.69246715650346147, 2.749719814763217141, -4.568240441793316897 ) ) ;
#20794=VERTEX_POINT ( 'NONE', #40098 ) ;
#20795=CARTESIAN_POINT ( 'NONE',  ( 16.14043045949875577, 15.25506048169804352, 0.6630684997064625330 ) ) ;
#20796=FACE_OUTER_BOUND ( 'NONE', #30247, .T. ) ;
#20801=CARTESIAN_POINT ( 'NONE',  ( 85.13880989351328310, 2.725772392624387308, 0.2960746283792183853 ) ) ;
#20802=CARTESIAN_POINT ( 'NONE',  ( 31.27801355750085222, -2.827678977088778911, 5.603419278764796729 ) ) ;
#20803=CARTESIAN_POINT ( 'NONE',  ( -77.50871672188519312, -4.892925716637096301, -9.117663693479695297 ) ) ;
#20804=CARTESIAN_POINT ( 'NONE',  ( 15.14474440143671607, -4.106796728886147108, 2.560655039386400489 ) ) ;
#20806=CARTESIAN_POINT ( 'NONE',  ( 30.58590753052908440, 0.06668957243665377121, -4.980068611744779439 ) ) ;
#20813=DIRECTION ( 'NONE',  ( -0.000000000000000000, -0.000000000000000000, -1.000000000000000000 ) ) ;
#20816=CARTESIAN_POINT ( 'NONE',  ( 21.70417851619663097, 4.205083555597296296, 2.944929548107457329 ) ) ;
#20819=CARTESIAN_POINT ( 'NONE',  ( -70.92837670881976919, 0.2170085631237942680, 10.00000000000113154 ) ) ;
#20825=CARTESIAN_POINT ( 'NONE',  ( 85.60524239217707532, 0.9672249164365797069, -5.812461325880615703 ) ) ;
#20826=CARTESIAN_POINT ( 'NONE',  ( -76.56376567441922987, 10.68475264541021552, 8.270291949397417852 ) ) ;
#20827=DIRECTION ( 'NONE',  ( 0.000000000000000000, -0.000000000000000000, 1.000000000000000000 ) ) ;
#20831=CARTESIAN_POINT ( 'NONE',  ( 24.04940727412492762, 3.336460009922597614, 3.254743572800636642 ) ) ;
#20838=CARTESIAN_POINT ( 'NONE',  ( 21.96606689427578374, 0.2111432007872987293, 7.751452917624079397 ) ) ;
#20839=CARTESIAN_POINT ( 'NONE',  ( 14.73588997190238459, -5.111296489852609426, -2.499999999999999556 ) ) ;
#20840=VECTOR ( 'NONE', #20269, 1000.000000000000000 ) ;
#20844=ORIENTED_EDGE ( 'NONE', *, *, #911, .T. ) ;
#20849=PLANE ( 'NONE',  #5332 ) ;
#20852=CARTESIAN_POINT ( 'NONE',  ( 29.52151182519568096, -2.704869923190903691, 5.373754524306347591 ) ) ;
#20857=CARTESIAN_POINT ( 'NONE',  ( -81.48430623221383939, -5.632154720818524751, 2.883670397763604676 ) ) ;
#20858=CARTESIAN_POINT ( 'NONE',  ( 23.59114525325624001, 0.4240393697126918493, -5.524181805179797955 ) ) ;
#20864=CARTESIAN_POINT ( 'NONE',  ( 34.14194983325678834, -3.845064528984907692, -5.237895465648701787 ) ) ;
#20868=CARTESIAN_POINT ( 'NONE',  ( -71.68115880895459213, -48.41814739710035553, 5.953156766150077495 ) ) ;
#20873=CARTESIAN_POINT ( 'NONE',  ( 20.40287464734031531, 10.75613383782063970, 2.500000000000000000 ) ) ;
#20874=CARTESIAN_POINT ( 'NONE',  ( 24.52499130180415676, 2.224616344218060870, -4.186325811553068377 ) ) ;
#20880=AXIS2_PLACEMENT_3D ( 'NONE', #28353, #8995, #37604 ) ;
#20882=CARTESIAN_POINT ( 'NONE',  ( 85.50394501772831291, 1.137698216002840157, 5.721642786829533200 ) ) ;
#20884=EDGE_CURVE ( 'NONE', #5201, #16788, #5596, .T. ) ;
#20888=CARTESIAN_POINT ( 'NONE',  ( -70.92837670882107659, 13.87661300689599386, -6.000000000000002665 ) ) ;
#20894=CARTESIAN_POINT ( 'NONE',  ( 21.82633866793786837, 5.573670839087305318, -3.484773916741194189 ) ) ;
#20900=( BOUNDED_CURVE ( )  B_SPLINE_CURVE ( 3, ( #36861, #34216, #8646, #3682 ),
 .UNSPECIFIED., .F., .F. ) 
 B_SPLINE_CURVE_WITH_KNOTS ( ( 4, 4 ),
 ( 2.498091544796508412, 2.888912398447714747 ),
 .UNSPECIFIED. ) 
 CURVE ( )  GEOMETRIC_REPRESENTATION_ITEM ( )  RATIONAL_B_SPLINE_CURVE ( ( 1.000000000000000000, 0.9873120399594201846, 0.9873120399594201846, 1.000000000000000000 ) ) 
 REPRESENTATION_ITEM ( '' )  );
#20902=CARTESIAN_POINT ( 'NONE',  ( 18.84457505903907659, 12.88015104982928172, 2.500000000000000000 ) ) ;
#20903=CARTESIAN_POINT ( 'NONE',  ( 21.85643539959778892, 9.726370091839324772, -5.619754257929120200 ) ) ;
#20906=CARTESIAN_POINT ( 'NONE',  ( -81.10340860069513269, 10.50981427116896683, 4.150601545968553907 ) ) ;
#20907=CARTESIAN_POINT ( 'NONE',  ( 14.62026587516738552, -4.585255206722739452, 2.500000000000073275 ) ) ;
#20908=CARTESIAN_POINT ( 'NONE',  ( -75.34513397755924302, 8.292114957421363286, -9.011728519595546771 ) ) ;
#20912=CARTESIAN_POINT ( 'NONE',  ( 14.85267465595546277, 12.69378753320559561, 2.508660318056822991 ) ) ;
#20915=EDGE_CURVE ( 'NONE', #25549, #25150, #19386, .T. ) ;
#20917=EDGE_CURVE ( 'NONE', #8080, #28300, #38634, .T. ) ;
#20921=ORIENTED_EDGE ( 'NONE', *, *, #8070, .T. ) ;
#20924=CARTESIAN_POINT ( 'NONE',  ( 30.51710498034237773, -0.1346816457499544206, 4.969330309792167277 ) ) ;
#20931=CARTESIAN_POINT ( 'NONE',  ( 86.24939746029500043, 1.399093175074125783, 5.441570408720817653 ) ) ;
#20934=ORIENTED_EDGE ( 'NONE', *, *, #31116, .F. ) ;
#20940=CARTESIAN_POINT ( 'NONE',  ( 26.38284721815838907, 1.220606850701035917, 4.361609309555559477 ) ) ;
#20942=ORIENTED_EDGE ( 'NONE', *, *, #2031, .F. ) ;
#20948=CARTESIAN_POINT ( 'NONE',  ( 63.05383694556373797, -7.271989087314214117, -6.000000000000000000 ) ) ;
#20953=CARTESIAN_POINT ( 'NONE',  ( 24.70548837460795610, 3.001373608382478242, -3.440348275608817730 ) ) ;
#20957=CARTESIAN_POINT ( 'NONE',  ( 22.58802438714224081, -2.565763546402358486, 8.787087332313648247 ) ) ;
#20959=CARTESIAN_POINT ( 'NONE',  ( 21.04004186717268965, 8.045167201113928357, 2.500000000002262190 ) ) ;
#20963=CARTESIAN_POINT ( 'NONE',  ( 84.55403409623259847, 2.802886334004389024, 2.719422554281196280 ) ) ;
#20964=B_SPLINE_CURVE_WITH_KNOTS ( 'NONE', 3,
 ( #6982, #32124, #16630, #25520, #7376, #38457, #38263, #32512 ),
 .UNSPECIFIED., .F., .F.,
 ( 4, 2, 2, 4 ),
 ( 3.990099683909797064E-17, 0.0004307664291302241554, 0.0006461496436953162838, 0.0008615328582604084122 ),
 .UNSPECIFIED. ) ;
#20967=EDGE_CURVE ( 'NONE', #8713, #28414, #1636, .T. ) ;
#20969=CARTESIAN_POINT ( 'NONE',  ( 14.74324248891501554, -5.593081337125382468, -2.503816905324318665 ) ) ;
#20971=CARTESIAN_POINT ( 'NONE',  ( 35.86767921836906226, -2.089981252190320937, -5.804416823763172140 ) ) ;
#20973=CARTESIAN_POINT ( 'NONE',  ( 22.69170078865038320, 0.3323897375237238605, -6.389351011922190793 ) ) ;
#20977=FACE_OUTER_BOUND ( 'NONE', #28859, .T. ) ;
#20982=CARTESIAN_POINT ( 'NONE',  ( 30.88492579994572296, 0.7017300443915822639, 4.487230210454935531 ) ) ;
#20983=CARTESIAN_POINT ( 'NONE',  ( 18.12789740749335010, -2.854475511803001631, 3.035694833931636971 ) ) ;
#20984=CARTESIAN_POINT ( 'NONE',  ( 17.77531322304072603, -3.190942049385152135, -2.940571408766233130 ) ) ;
#20985=CARTESIAN_POINT ( 'NONE',  ( 14.77315594796472631, 13.19392823276517568, -2.499999999999998668 ) ) ;
#20986=ORIENTED_EDGE ( 'NONE', *, *, #32052, .T. ) ;
#20995=CARTESIAN_POINT ( 'NONE',  ( 21.88711032999522743, 3.208699644441221022, 3.395463446396979279 ) ) ;
#20997=CARTESIAN_POINT ( 'NONE',  ( 23.42598874491005034, 3.327995987485997897, 3.701944623341963503 ) ) ;
#20999=VECTOR ( 'NONE', #1534, 1000.000000000000000 ) ;
#21000=ADVANCED_FACE ( 'NONE', ( #13526 ), #15254, .F. ) ;
#21004=CARTESIAN_POINT ( 'NONE',  ( 17.03255388622768507, -3.044842113014305962, -2.864739986454959642 ) ) ;
#21008=CARTESIAN_POINT ( 'NONE',  ( 22.04800161786629431, 2.700078594769402152, -5.146687023986929788 ) ) ;
#21012=AXIS2_PLACEMENT_3D ( 'NONE', #39105, #17075, #5146 ) ;
#21018=CARTESIAN_POINT ( 'NONE',  ( 85.11099552155531001, 2.757014815357352155, -1.204572545719858834 ) ) ;
#21019=PLANE ( 'NONE',  #9628 ) ;
#21025=CARTESIAN_POINT ( 'NONE',  ( 15.15534889434650090, -4.116562409201322659, 2.560140338179660358 ) ) ;
#21028=CARTESIAN_POINT ( 'NONE',  ( 37.07067537406068425, -2.906362785499426060, -5.992173468430849859 ) ) ;
#21032=CARTESIAN_POINT ( 'NONE',  ( -70.92837670882107659, -23.80776546975053165, 0.000000000000000000 ) ) ;
#21033=VECTOR ( 'NONE', #22392, 1000.000000000000000 ) ;
#21036=CARTESIAN_POINT ( 'NONE',  ( 30.84889139629300558, 0.6455805249289596759, 4.592240215719487040 ) ) ;
#21045=CARTESIAN_POINT ( 'NONE',  ( 18.54789246542846470, 7.518219598317671171, 3.101245220341271036 ) ) ;
#21046=CARTESIAN_POINT ( 'NONE',  ( -73.59524413808043164, 8.148159543145636619, 9.640765774018305478 ) ) ;
#21048=VERTEX_POINT ( 'NONE', #39429 ) ;
#21052=CARTESIAN_POINT ( 'NONE',  ( 21.99994241389349980, 5.558807285328593473, 3.121874822124243387 ) ) ;
#21058=CARTESIAN_POINT ( 'NONE',  ( 21.73405496294427053, 0.2198986141765594815, 9.095395277813500101 ) ) ;
#21059=CARTESIAN_POINT ( 'NONE',  ( 14.69507384520581361, -4.883229594507451310, -2.499999999999376055 ) ) ;
#21064=CARTESIAN_POINT ( 'NONE',  ( 0.7201709579117279159, -51.60714625320436255, 2.500000000000000000 ) ) ;
#21068=CARTESIAN_POINT ( 'NONE',  ( 31.28551011801044268, -2.837290201336624129, -5.599793116354693012 ) ) ;
#21071=CARTESIAN_POINT ( 'NONE',  ( -80.68515367620979362, -6.621186074883498307, 2.228965439759364564 ) ) ;
#21072=CARTESIAN_POINT ( 'NONE',  ( 24.12565218530084366, 0.5136036009149196335, -5.092665358616495830 ) ) ;
#21074=LINE ( 'NONE', #21691, #1165 ) ;
#21079=FACE_BOUND ( 'NONE', #15062, .T. ) ;
#21080=CARTESIAN_POINT ( 'NONE',  ( 36.13131606425951503, -1.533108014538433039, -5.645148619362555742 ) ) ;
#21089=CARTESIAN_POINT ( 'NONE',  ( 22.81770739701413930, 1.428927919918285605, -5.507341944819657442 ) ) ;
#21093=AXIS2_PLACEMENT_3D ( 'NONE', #12668, #25242, #22771 ) ;
#21096=DIRECTION ( 'NONE',  ( 0.000000000000000000, 1.000000000000000000, 0.000000000000000000 ) ) ;
#21098=CARTESIAN_POINT ( 'NONE',  ( -70.53519588576141075, -48.57790317178756823, 9.993926770235830759 ) ) ;
#21099=CARTESIAN_POINT ( 'NONE',  ( 1.700390093233090871, -29.56993018339339940, 6.000000000000000000 ) ) ;
#21104=PLANE ( 'NONE',  #27792 ) ;
#21111=CARTESIAN_POINT ( 'NONE',  ( 17.73639088777611761, 11.88077751880594768, -2.499999999999990230 ) ) ;
#21114=CARTESIAN_POINT ( 'NONE',  ( 23.94692112590556832, 2.808164783556298616, 3.943894218810308328 ) ) ;
#21115=CARTESIAN_POINT ( 'NONE',  ( 17.35960385848256493, 14.27653579843486220, 2.500000000000000444 ) ) ;
#21117=CARTESIAN_POINT ( 'NONE',  ( 21.85643539959774273, 9.214175136349357587, -0.8338435668127727185 ) ) ;
#21121=CARTESIAN_POINT ( 'NONE',  ( 14.75290036705818508, -5.144397853053700231, 2.500000000000000444 ) ) ;
#21122=CARTESIAN_POINT ( 'NONE',  ( -74.02478150447711869, 6.647606516902553331, -9.563567244161919945 ) ) ;
#21127=CARTESIAN_POINT ( 'NONE',  ( 14.89578813002483670, 12.34317254588458468, 2.524919271954451094 ) ) ;
#21131=CARTESIAN_POINT ( 'NONE',  ( 16.38665980882106155, 15.06251823374549303, -2.500000000000000000 ) ) ;
#21133=CARTESIAN_POINT ( 'NONE',  ( 87.08948198750766778, 0.5346849121671046756, 4.856188771401600768 ) ) ;
#21134=CARTESIAN_POINT ( 'NONE',  ( 26.49611857872572784, 1.696983071862875336, -4.309887170283649205 ) ) ;
#21135=ORIENTED_EDGE ( 'NONE', *, *, #2009, .T. ) ;
#21138=CARTESIAN_POINT ( 'NONE',  ( 35.33522366009476912, -3.174037382202389512, 5.721314256408138732 ) ) ;
#21140=CARTESIAN_POINT ( 'NONE',  ( 85.55911739799610416, 1.969564878966352905, 4.951173091362058187 ) ) ;
#21154=CARTESIAN_POINT ( 'NONE',  ( 25.33366054371228770, 0.7754436759679742552, 4.607944210112060013 ) ) ;
#21165=CARTESIAN_POINT ( 'NONE',  ( 24.00944515006052171, 3.309123255076573678, -3.353452565180164324 ) ) ;
#21168=CARTESIAN_POINT ( 'NONE',  ( 24.43802896994273510, -0.4903351684736660387, 6.966919456710074954 ) ) ;
#21169=DIRECTION ( 'NONE',  ( 1.165409145176969993E-16, -1.000000000000000000, 0.000000000000000000 ) ) ;
#21173=CARTESIAN_POINT ( 'NONE',  ( 86.42495861400665547, -0.1300389677119091758, -5.942483626122943896 ) ) ;
#21178=CARTESIAN_POINT ( 'NONE',  ( 14.85208526505567050, -4.487224198574636169, -2.516407688438223822 ) ) ;
#21180=DIRECTION ( 'NONE',  ( -0.000000000000000000, 0.000000000000000000, -1.000000000000000000 ) ) ;
#21185=CARTESIAN_POINT ( 'NONE',  ( 85.52484820210342775, 2.292155841932438154, 3.149942891487422791 ) ) ;
#21186=VERTEX_POINT ( 'NONE', #18425 ) ;
#21189=CARTESIAN_POINT ( 'NONE',  ( 36.49369427451753722, -3.560799718971868089, 5.796041169543606486 ) ) ;
#21190=CARTESIAN_POINT ( 'NONE',  ( 19.68761177061032086, -2.696979717695116463, 3.279125982130457473 ) ) ;
#21191=CARTESIAN_POINT ( 'NONE',  ( 20.50705206718803808, -3.049029319690857776, -3.332098049053498823 ) ) ;
#21200=CARTESIAN_POINT ( 'NONE',  ( 14.77222811005485603, -4.461988841550141416, 2.511961482897715481 ) ) ;
#21202=CARTESIAN_POINT ( 'NONE',  ( 24.71742244748645945, 2.639037666618674116, 3.924515567304096120 ) ) ;
#21203=CARTESIAN_POINT ( 'NONE',  ( 21.33678673121765712, 8.399421056148055342, -2.668923178601029456 ) ) ;
#21205=ADVANCED_FACE ( 'NONE', ( #34320 ), #15059, .T. ) ;
#21209=DIRECTION ( 'NONE',  ( 0.000000000000000000, 0.000000000000000000, 1.000000000000000000 ) ) ;
#21210=CARTESIAN_POINT ( 'NONE',  ( 21.57378257072032213, -2.652646515802797200, -3.573508552700807250 ) ) ;
#21211=FACE_OUTER_BOUND ( 'NONE', #518, .T. ) ;
#21213=CARTESIAN_POINT ( 'NONE',  ( 22.03527598358551387, 3.722255905023069911, -4.359252203237127254 ) ) ;
#21215=CARTESIAN_POINT ( 'NONE',  ( 21.85643539959774273, 11.92045248574714300, 0.01447246376323708950 ) ) ;
#21220=CARTESIAN_POINT ( 'NONE',  ( 85.09863483756090830, 2.770898922293168809, 1.806811963633389695 ) ) ;
#21223=VECTOR ( 'NONE', #6421, 1000.000000000000000 ) ;
#21225=ORIENTED_EDGE ( 'NONE', *, *, #32206, .T. ) ;
#21226=CARTESIAN_POINT ( 'NONE',  ( 31.37373683152652148, -3.593601361316209886, 4.916934954046649153 ) ) ;
#21228=CARTESIAN_POINT ( 'NONE',  ( 36.63366809872980667, -3.081676326702182056, -5.923967914054548700 ) ) ;
#21231=CARTESIAN_POINT ( 'NONE',  ( -70.92837670882107659, -56.35932253828835314, 0.000000000000000000 ) ) ;
#21235=CARTESIAN_POINT ( 'NONE',  ( 30.81594338096673980, 0.5927415480317952401, 4.684896961509361191 ) ) ;
#21244=CARTESIAN_POINT ( 'NONE',  ( -73.55410448504031251, 8.091590788868597173, -9.651951412758178250 ) ) ;
#21248=LINE ( 'NONE', #18345, #36542 ) ;
#21252=CARTESIAN_POINT ( 'NONE',  ( 24.03985768575755344, 3.329662727276597511, 3.280238031040798141 ) ) ;
#21257=CARTESIAN_POINT ( 'NONE',  ( 24.05471417302198489, 3.308817292245012975, -3.187513558550173265 ) ) ;
#21260=CARTESIAN_POINT ( 'NONE',  ( 23.04769222910721993, 0.3307062739915670457, 5.968048623999395730 ) ) ;
#21266=CARTESIAN_POINT ( 'NONE',  ( 35.34196908527864878, -3.786851321365131806, -5.507838251830221132 ) ) ;
#21270=DIRECTION ( 'NONE',  ( 0.000000000000000000, 0.000000000000000000, 1.000000000000000000 ) ) ;
#21272=CARTESIAN_POINT ( 'NONE',  ( 29.46612689758034875, 1.430465584783186639, -3.840811867917949929 ) ) ;
#21276=CARTESIAN_POINT ( 'NONE',  ( 25.36727076954679916, 0.7411443615474921920, -4.603813888107473495 ) ) ;
#21280=FACE_OUTER_BOUND ( 'NONE', #33964, .T. ) ;
#21281=CARTESIAN_POINT ( 'NONE',  ( 35.16097584309888902, -1.161037321149452239, -5.517930166532758918 ) ) ;
#21284=DIRECTION ( 'NONE',  ( -0.000000000000000000, -0.000000000000000000, 1.000000000000000000 ) ) ;
#21290=CARTESIAN_POINT ( 'NONE',  ( 14.76475291679427393, -5.159125289594414632, -2.500001731999736077 ) ) ;
#21297=CARTESIAN_POINT ( 'NONE',  ( 87.88829317789571860, -2.466143857431153830, 1.215092630805642671 ) ) ;
#21306=CARTESIAN_POINT ( 'NONE',  ( 24.76343259005120601, 3.021619590193751925, 3.339778374755230317 ) ) ;
#21317=CARTESIAN_POINT ( 'NONE',  ( 22.36801796201435977, 4.217314093436514533, 3.697468194167767841 ) ) ;
#21320=CARTESIAN_POINT ( 'NONE',  ( 21.85643539959772497, -11.05315871940826078, 3.104450560420165317 ) ) ;
#21322=CARTESIAN_POINT ( 'NONE',  ( -79.46431696083011786, 10.38012969939556740, 7.168986771804887859 ) ) ;
#21323=CARTESIAN_POINT ( 'NONE',  ( 36.19706241022630877, -3.644680151509849253, 5.718849134531836853 ) ) ;
#21326=CARTESIAN_POINT ( 'NONE',  ( -73.53200420073510202, 5.707097961328267743, -10.87087679806554341 ) ) ;
#21327=DIRECTION ( 'NONE',  ( 0.000000000000000000, -0.000000000000000000, -1.000000000000000000 ) ) ;
#21328=CARTESIAN_POINT ( 'NONE',  ( 36.88849515942500545, -3.352853972477296995, -5.910143701334799715 ) ) ;
#21329=B_SPLINE_CURVE_WITH_KNOTS ( 'NONE', 3,
 ( #9182, #11849, #17614, #27104, #30827, #12050, #5904, #36777, #8560, #31030 ),
 .UNSPECIFIED., .F., .F.,
 ( 4, 2, 2, 2, 4 ),
 ( 0.001566336636202482176, 0.001957536639217857637, 0.002348736642233233314, 0.002739936645248608992, 0.003131136648263984669 ),
 .UNSPECIFIED. ) ;
#21331=CARTESIAN_POINT ( 'NONE',  ( 15.16924916808596357, 11.40858824471275312, 2.573926220994043224 ) ) ;
#21333=CARTESIAN_POINT ( 'NONE',  ( 29.36363007681232418, -3.858821234667521249, 4.337399626228677363 ) ) ;
#21336=CARTESIAN_POINT ( 'NONE',  ( 17.32389278323182680, 14.30653710295208647, -2.500000000000000000 ) ) ;
#21338=CARTESIAN_POINT ( 'NONE',  ( 24.53892863518501599, 2.743979168526681445, -3.872037506538268392 ) ) ;
#21341=CARTESIAN_POINT ( 'NONE',  ( 33.68675182762641640, -1.062721320211014175, 5.464030358509579521 ) ) ;
#21342=CARTESIAN_POINT ( 'NONE',  ( 0.6783104270758654186, -48.60743831809499227, 6.000000000000000000 ) ) ;
#21344=CARTESIAN_POINT ( 'NONE',  ( 88.25293897076788596, -0.9571425830051931705, -4.167473131139645126 ) ) ;
#21345=CARTESIAN_POINT ( 'NONE',  ( 31.28447350889217304, -0.4025536940246822737, -5.089096727550352917 ) ) ;
#21346=B_SPLINE_CURVE_WITH_KNOTS ( 'NONE', 3,
 ( #30562, #37333, #21290, #27659, #15306, #14681, #17975, #34284, #15099, #2372, #21500, #24368, #34077, #11587, #33463, #2993, #40620, #14890 ),
 .UNSPECIFIED., .F., .F.,
 ( 4, 2, 2, 2, 2, 2, 2, 2, 4 ),
 ( 0.000000000000000000, 2.302533481709740794E-05, 4.605066963419481588E-05, 9.210133926839220674E-05, 0.0001842026785367869614, 0.0003684053570735786390, 0.0005526080356103703437, 0.0006447093748787674971, 0.0007368107141471646505 ),
 .UNSPECIFIED. ) ;
#21349=CARTESIAN_POINT ( 'NONE',  ( -69.95454086882011779, -21.04534624052442382, 5.920661432671354696 ) ) ;
#21354=AXIS2_PLACEMENT_3D ( 'NONE', #18898, #3288, #32284 ) ;
#21356=ORIENTED_EDGE ( 'NONE', *, *, #6102, .F. ) ;
#21361=CARTESIAN_POINT ( 'NONE',  ( 14.77315594796471743, 13.19392823276620419, 2.499999999999996891 ) ) ;
#21368=CARTESIAN_POINT ( 'NONE',  ( 24.33330849205117374, 3.134806574687862391, -3.409030949822150713 ) ) ;
#21370=CARTESIAN_POINT ( 'NONE',  ( 24.76528640762570888, -1.939968142380837701, -6.533370004292007316 ) ) ;
#21372=CARTESIAN_POINT ( 'NONE',  ( 1.700390093233090871, -29.56993018339339940, -2.499999999999998668 ) ) ;
#21374=CARTESIAN_POINT ( 'NONE',  ( 84.24490603200722205, 3.007448030680667017, 1.128815683486722454 ) ) ;
#21383=DIRECTION ( 'NONE',  ( -0.000000000000000000, -1.000000000000000000, -0.000000000000000000 ) ) ;
#21384=CARTESIAN_POINT ( 'NONE',  ( 33.11740971841622638, -3.526206640162208750, -5.310590497510783159 ) ) ;
#21386=LINE ( 'NONE', #33962, #26003 ) ;
#21389=ORIENTED_EDGE ( 'NONE', *, *, #6381, .F. ) ;
#21392=CARTESIAN_POINT ( 'NONE',  ( 86.50262394474026451, 1.193871719766480100, -4.934721793127618383 ) ) ;
#21396=CARTESIAN_POINT ( 'NONE',  ( 36.44620324436766623, -1.730678941397710169, 5.729688724127439237 ) ) ;
#21398=CARTESIAN_POINT ( 'NONE',  ( 26.12357031956679876, -2.759746946588834682, 4.283612967940825911 ) ) ;
#21410=CARTESIAN_POINT ( 'NONE',  ( 23.67960553047068473, 2.561144650517011456, 4.199896394371767094 ) ) ;
#21411=CARTESIAN_POINT ( 'NONE',  ( 31.22136964576698404, 0.5681969411430533023, 4.564728438945290456 ) ) ;
#21414=VECTOR ( 'NONE', #6476, 1000.000000000000000 ) ;
#21418=CARTESIAN_POINT ( 'NONE',  ( 85.15434555589628474, 2.708321999268741731, -0.5844145583951695366 ) ) ;
#21421=CARTESIAN_POINT ( 'NONE',  ( 23.74549009334706540, 2.920879532582420168, -3.920752113660479932 ) ) ;
#21423=AXIS2_PLACEMENT_3D ( 'NONE', #7457, #16123, #28688 ) ;
#21425=CARTESIAN_POINT ( 'NONE',  ( 21.85643539959774273, -11.65679437655345474, 11.20963770477306554 ) ) ;
#21431=CARTESIAN_POINT ( 'NONE',  ( 88.21591849536395102, -0.7305820373589052563, 3.481732356799086769 ) ) ;
#21434=CARTESIAN_POINT ( 'NONE',  ( 31.37751630285753990, -3.642699559265466291, 4.877213502604051953 ) ) ;
#21436=CARTESIAN_POINT ( 'NONE',  ( 32.78155291855927089, -0.9262908896100177092, -5.322752176431207793 ) ) ;
#21439=ADVANCED_FACE ( 'NONE', ( #18383 ), #1958, .F. ) ;
#21440=EDGE_CURVE ( 'NONE', #3377, #40670, #33459, .T. ) ;
#21443=LINE ( 'NONE', #15248, #19016 ) ;
#21448=CARTESIAN_POINT ( 'NONE',  ( 34.60561289930970474, -0.8402221667057534482, 5.339566637150812589 ) ) ;
#21453=EDGE_LOOP ( 'NONE', ( #31927, #21923, #30170, #4103, #40526, #8142, #8509, #19370 ) ) ;
#21454=CARTESIAN_POINT ( 'NONE',  ( -71.92837670882107659, -65.19654454972992141, 5.916079783099617906 ) ) ;
#21461=CARTESIAN_POINT ( 'NONE',  ( 22.39063959453807939, 4.900407498310523025, 3.082520428777218324 ) ) ;
#21479=CARTESIAN_POINT ( 'NONE',  ( 31.96174557538834193, -4.583587016071825282, 3.235063174744643000 ) ) ;
#21480=FACE_OUTER_BOUND ( 'NONE', #22277, .T. ) ;
#21483=CARTESIAN_POINT ( 'NONE',  ( 23.60498067204314410, 0.4413003733997728495, -5.510345162601594460 ) ) ;
#21485=AXIS2_PLACEMENT_3D ( 'NONE', #22701, #29070, #19991 ) ;
#21491=CARTESIAN_POINT ( 'NONE',  ( 36.41841363650763697, -1.780316330609500675, -5.760878658093356641 ) ) ;
#21492=CARTESIAN_POINT ( 'NONE',  ( 30.87873567178753831, -3.511903919675081642, -4.882802410549687444 ) ) ;
#21500=CARTESIAN_POINT ( 'NONE',  ( 14.72811636034318639, -4.878256426182215222, -2.502161937363848843 ) ) ;
#21501=CARTESIAN_POINT ( 'NONE',  ( 23.52668297624172666, 2.287558078930879368, -4.447727279419068758 ) ) ;
#21507=CARTESIAN_POINT ( 'NONE',  ( 84.50243033367722489, 2.523019330700893903, 3.504063919878146027 ) ) ;
#21518=CARTESIAN_POINT ( 'NONE',  ( 21.98762963305790308, 5.627346946651078596, 3.080487669913397841 ) ) ;
#21520=VERTEX_POINT ( 'NONE', #28264 ) ;
#21522=CARTESIAN_POINT ( 'NONE',  ( 15.71701945473647655, 8.042377430118643034, -3.484701709439959494 ) ) ;
#21529=CARTESIAN_POINT ( 'NONE',  ( 21.85643539959774273, -6.858222381794880640, 10.60035608423801357 ) ) ;
#21531=CARTESIAN_POINT ( 'NONE',  ( -74.90361456537704044, 9.559336010372646797, 9.177345781745600561 ) ) ;
#21537=CARTESIAN_POINT ( 'NONE',  ( 35.36814664345466497, -3.792965548836813028, -5.510366441342056554 ) ) ;
#21543=CIRCLE ( 'NONE', #17565, 10.00000000000000888 ) ;
#21547=CARTESIAN_POINT ( 'NONE',  ( 30.98497569240768001, -3.765466457291608116, -4.599884699063723659 ) ) ;
#21549=CARTESIAN_POINT ( 'NONE',  ( 25.67913400440570015, 2.136453941815092961, -4.141921070930310478 ) ) ;
#21552=CARTESIAN_POINT ( 'NONE',  ( 36.82698429609488500, -3.168745687177260351, 5.951708789409448919 ) ) ;
#21555=CARTESIAN_POINT ( 'NONE',  ( 87.30391260081773908, -0.2898811470106905652, 5.673122884556256906 ) ) ;
#21556=CARTESIAN_POINT ( 'NONE',  ( 29.97939791730999914, 0.4010955892747467555, 5.210136963171234648 ) ) ;
#21557=CARTESIAN_POINT ( 'NONE',  ( 33.93672751689359757, -1.338894892125421565, -5.503045110504557691 ) ) ;
#21560=B_SPLINE_CURVE_WITH_KNOTS ( 'NONE', 5,
 ( #36781, #8564, #39869, #20931, #30627, #5288, #17825, #2433 ),
 .UNSPECIFIED., .F., .F.,
 ( 6, 2, 6 ),
 ( 0.000000000000000000, 0.5000000000000000000, 1.000000000000000000 ),
 .UNSPECIFIED. ) ;
#21561=VERTEX_POINT ( 'NONE', #24989 ) ;
#21562=CARTESIAN_POINT ( 'NONE',  ( 24.67496769583028993, 2.993954329345769771, 3.481334102667019259 ) ) ;
#21566=ORIENTED_EDGE ( 'NONE', *, *, #7909, .T. ) ;
#21568=CARTESIAN_POINT ( 'NONE',  ( 24.75839165839662925, 3.019244830385916956, -3.350409272483306111 ) ) ;
#21578=CARTESIAN_POINT ( 'NONE',  ( 23.42649477596276952, 3.757704045721736996, -3.184095338007110421 ) ) ;
#21581=CARTESIAN_POINT ( 'NONE',  ( 24.43246502961036626, -0.4583524411608039251, -6.968550363799582925 ) ) ;
#21582=CARTESIAN_POINT ( 'NONE',  ( -79.49313711070512056, -5.542708507839796184, -7.172005795361188873 ) ) ;
#21585=CARTESIAN_POINT ( 'NONE',  ( 87.67494654488285732, -1.518266458920173312, 4.408571129606221994 ) ) ;
#21586=DIRECTION ( 'NONE',  ( 0.000000000000000000, 1.000000000000000000, 0.000000000000000000 ) ) ;
#21590=DIRECTION ( 'NONE',  ( 0.000000000000000000, 1.000000000000000000, 0.000000000000000000 ) ) ;
#21591=CARTESIAN_POINT ( 'NONE',  ( 18.25124071569355877, -3.122163946110289245, -3.009088641841451306 ) ) ;
#21593=CARTESIAN_POINT ( 'NONE',  ( 20.42172546146963796, 3.659902873894464115, -3.393702178195764585 ) ) ;
#21597=CARTESIAN_POINT ( 'NONE',  ( 34.92873844507915493, -1.712022664174882358, 5.657872407722902786 ) ) ;
#21599=CARTESIAN_POINT ( 'NONE',  ( 85.18642856628412119, 2.672284839249654542, -1.189885989438959069 ) ) ;
#21600=ORIENTED_EDGE ( 'NONE', *, *, #5683, .F. ) ;
#21602=DIRECTION ( 'NONE',  ( 1.000000000000000000, 0.000000000000000000, 0.000000000000000000 ) ) ;
#21604=CARTESIAN_POINT ( 'NONE',  ( 16.51093427324735430, -3.201950870117511450, 2.783328630431367579 ) ) ;
#21607=CARTESIAN_POINT ( 'NONE',  ( 28.66920249112477848, -4.024975064351027143, -4.110187144531254333 ) ) ;
#21614=CARTESIAN_POINT ( 'NONE',  ( 23.93610855655161274, 2.571716072343740667, 4.117792848012141960 ) ) ;
#21615=CARTESIAN_POINT ( 'NONE',  ( 35.16676341537907291, -1.025548178550078626, 5.403050771363623994 ) ) ;
#21622=CARTESIAN_POINT ( 'NONE',  ( 8.290806648384990041, -25.50263309590217276, -6.000000000000001776 ) ) ;
#21625=CARTESIAN_POINT ( 'NONE',  ( 24.42172553482546959, 2.823060965057244243, -3.827932450290554733 ) ) ;
#21628=CARTESIAN_POINT ( 'NONE',  ( 21.85643539959777470, -5.354795180264900978, -13.61019886989645933 ) ) ;
#21633=CARTESIAN_POINT ( 'NONE',  ( 86.85660104221420852, 0.7962678431171816840, 5.176869783008884340 ) ) ;
#21635=EDGE_LOOP ( 'NONE', ( #29269, #6517 ) ) ;
#21636=CARTESIAN_POINT ( 'NONE',  ( 29.20850709934801159, 2.242166301403143880, -0.5075834600922535245 ) ) ;
#21638=CARTESIAN_POINT ( 'NONE',  ( 17.13439990770066856, -3.171075681061939822, 2.872495620988768206 ) ) ;
#21641=CARTESIAN_POINT ( 'NONE',  ( 33.46229367853198511, -3.089018271621291500, -5.428998235802485972 ) ) ;
#21643=CARTESIAN_POINT ( 'NONE',  ( -0.000000000000000000, 13.37661300689600097, -6.000000000000000000 ) ) ;
#21647=CARTESIAN_POINT ( 'NONE',  ( -70.92837670882107659, -45.61702805680359063, 6.000000000000002665 ) ) ;
#21650=CARTESIAN_POINT ( 'NONE',  ( 36.48451820331894169, -3.515659605614979810, 5.817203863836646782 ) ) ;
#21654=CARTESIAN_POINT ( 'NONE',  ( -71.90229890510927646, -0.5209448599347925590, 9.952588678376171671 ) ) ;
#21658=CARTESIAN_POINT ( 'NONE',  ( 88.37073220026057641, -0.9044761386004964709, -0.07382722449155432187 ) ) ;
#21664=CARTESIAN_POINT ( 'NONE',  ( 22.39423033477626745, 4.887851171428074792, 3.091777426714782617 ) ) ;
#21671=CARTESIAN_POINT ( 'NONE',  ( -72.23801069314184531, -46.35958874329211454, 5.855843091881858697 ) ) ;
#21675=EDGE_CURVE ( 'NONE', #28854, #37831, #4183, .T. ) ;
#21678=ORIENTED_EDGE ( 'NONE', *, *, #17819, .T. ) ;
#21684=PLANE ( 'NONE',  #22273 ) ;
#21685=CARTESIAN_POINT ( 'NONE',  ( 30.98800548345937855, -0.8519925708576415735, -5.886550247782252221 ) ) ;
#21686=PLANE ( 'NONE',  #4983 ) ;
#21689=CARTESIAN_POINT ( 'NONE',  ( 27.36544478893236487, 1.086804081426588242, -4.476750403029456926 ) ) ;
#21691=CARTESIAN_POINT ( 'NONE',  ( -0.000000000000000000, 13.37661300689600097, -2.500000000000000000 ) ) ;
#21692=DIRECTION ( 'NONE',  ( 0.000000000000000000, -0.000000000000000000, -1.000000000000000000 ) ) ;
#21694=CARTESIAN_POINT ( 'NONE',  ( -12.99139449055068596, 10.37661300689600097, 6.000000000000000000 ) ) ;
#21696=CARTESIAN_POINT ( 'NONE',  ( 36.99638130734812336, -3.220727926517238160, -5.952632950965317526 ) ) ;
#21715=CARTESIAN_POINT ( 'NONE',  ( 22.38233119875572186, 4.942362494773947290, 3.043640801607715218 ) ) ;
#21716=CIRCLE ( 'NONE', #3982, 9.804803391925412726 ) ;
#21719=ORIENTED_EDGE ( 'NONE', *, *, #13709, .F. ) ;
#21729=CARTESIAN_POINT ( 'NONE',  ( 21.85643539959777115, -1.513967970512005268, 12.69801924519992120 ) ) ;
#21731=CARTESIAN_POINT ( 'NONE',  ( -76.72287709695605429, 9.359952303362009118, 8.166909960842559713 ) ) ;
#21737=CARTESIAN_POINT ( 'NONE',  ( 36.13343955306980604, -1.529194832581077135, -5.642286574374616670 ) ) ;
#21741=CARTESIAN_POINT ( 'NONE',  ( 29.98495624012389982, -3.733826441308198962, 4.538579857738193724 ) ) ;
#21743=CARTESIAN_POINT ( 'NONE',  ( 17.33572800788162738, 14.29660996616593849, -2.500000000000000444 ) ) ;
#21744=CARTESIAN_POINT ( 'NONE',  ( 23.13463400706473649, 0.4140889092209439903, -5.868895817274544235 ) ) ;
#21745=CARTESIAN_POINT ( 'NONE',  ( 36.53420504795911938, -1.804924688322298909, -5.759860367675933013 ) ) ;
#21746=CARTESIAN_POINT ( 'NONE',  ( 26.91012592398995551, 1.445922882693422729, -4.391925638988915637 ) ) ;
#21749=CARTESIAN_POINT ( 'NONE',  ( 36.44546669202388500, -3.301925173002164815, 5.889632857546714284 ) ) ;
#21753=CARTESIAN_POINT ( 'NONE',  ( 85.43170627155664931, 2.122511629702291902, -4.702826977918449280 ) ) ;
#21755=CARTESIAN_POINT ( 'NONE',  ( 33.90241230359465874, -5.503808810968542353, 0.4955917775451662566 ) ) ;
#21756=CARTESIAN_POINT ( 'NONE',  ( 22.22893185000578953, 4.118675178843608897, 2.394718637401875405 ) ) ;
#21758=CARTESIAN_POINT ( 'NONE',  ( 25.10207142344970421, 2.436503095005564390, 4.015748850599299757 ) ) ;
#21775=B_SPLINE_SURFACE_WITH_KNOTS ( 'NONE', 5, 3, ( 
 ( #38018, #16199, #13512, #13114, #16394, #16786, #9819, #3878, #19890, #38215, #25672, #1185, #13720, #770, #32272, #35162, #26286, #6935, #22398, #38820, #38617, #10012, #19290, #13302, #10214, #29167, #28765, #22795, #35366, #7137, #19697, #4071, #16586, #975, #26082, #32867, #17384, #23775, #11411, #29965, #33275, #20282, #7932, #27278, #23387, #17588, #2188 ),
 ( #36352, #2402, #33066, #20903, #30169, #4850, #20482, #1777, #8119, #39846, #29758, #14508, #36550, #24192, #30384, #14306, #5465, #20691, #18005, #27083, #8328, #5258, #33489, #4655, #26682, #1572, #26876, #39628, #11613, #39217, #26481, #5056, #10811, #11210, #17798, #36752, #33686, #17190, #23978, #11006, #23590, #39009, #35954, #1990, #14104, #14706, #8537 ),
 ( #21117, #30594, #7735, #39420, #36154, #8737, #2609, #15541, #120, #28095, #19045, #40649, #36957, #11817, #24399, #3021, #28301, #15128, #9352, #9153, #37158, #37754, #21933, #34310, #31404, #24816, #21320, #40240, #12651, #25020, #27684, #21529, #25226, #2809, #9564, #21729, #24603, #12451, #3229, #6079, #8944, #12024, #12242, #30803, #31608, #18614, #14924 ),
 ( #34507, #22144, #5879, #18416, #34716, #6495, #37358, #31201, #31004, #27493, #18832, #40042, #15331, #37557, #33895, #6283, #5671, #18211, #34105, #27886, #40433, #6697, #13063, #31812, #26036, #22754, #35713, #16739, #16152, #38776, #9770, #25624, #318, #38570, #37965, #35516, #38169, #16544, #7489, #19245, #29323, #26244, #7286, #15944, #1140, #28716, #4026 ),
 ( #19850, #3431, #28921, #25424, #928, #3829, #32023, #9972, #25830, #23145, #19654, #22953, #35321, #22353, #34920, #3628, #527, #22552, #16347, #10572, #20049, #13674, #29124, #35115, #722, #12857, #28509, #19449, #13462, #10377, #13263, #38366, #10163, #32225, #7090, #32419, #4218, #32629, #26638, #30129, #32824, #35914, #23933, #17541, #39172, #26835, #17145 ),
 ( #4423, #29525, #14264, #38966, #8278, #14660, #27232, #29717, #36307, #1944, #36505, #10968, #39375, #26440, #20242, #33224, #17750, #5010, #36704, #14462, #13873, #1337, #10766, #20643, #5213, #4615, #27037, #11165, #14060, #39797, #39581, #23736, #20852, #1733, #23342, #1526, #30335, #11366, #23548, #36113, #2142, #20442, #11566, #8079, #7890, #33445, #24142 ),
 ( #33021, #29915, #7693, #8487, #16947, #4810, #17338, #12195, #15490, #21884, #11978, #24556, #6237, #28250, #2761, #27840, #37110, #21068, #24974, #18781, #8896, #37312, #39998, #31155, #3184, #2971, #33642, #21479, #40599, #24348, #15698, #28048, #5417, #34057, #12406, #36912, #30756, #8692, #37511, #40393, #12607, #34461, #33844, #74, #27442, #2558, #17956 ),
 ( #9306, #15080, #34263, #25173, #21272, #31358, #37705, #30540, #2350, #14869, #5622, #21685, #15287, #24765, #6034, #11767, #18162, #27640, #40197, #5830, #18370, #30957, #18568, #9109, #5285, #21755, #40068, #30193, #30622, #40265, #2837, #12269, #11436, #5697, #17822, #2212, #5082, #2013, #27517, #24001, #21556, #27914, #40460, #14731, #8762, #15155, #37182 ) ),
 .UNSPECIFIED., .F., .T., .F.,
 ( 6, 2, 6 ),
 ( 4, 1, 1, 1, 1, 1, 1, 1, 1, 1, 1, 1, 1, 1, 1, 1, 1, 1, 1, 1, 1, 1, 1, 1, 1, 1, 1, 1, 1, 1, 1, 1, 1, 1, 1, 1, 1, 1, 1, 1, 1, 1, 1, 1, 4 ),
 ( 0.000000000000000000, 0.5000000000000000000, 1.000000000000000000 ),
 ( -0.09263217477943377909, -0.08973741931757646395, -0.08732512309936206474, -0.08539528612479052594, -0.08394790839386186143, -0.08250053066293322468, -0.08105315293200456017, -0.07960577520107590954, -0.07815839747014724503, -0.07671101973921859440, -0.07478118276464705561, -0.07285134579007553068, -0.07092150881550399188, -0.06947413108457534126, -0.06802675335364669063, -0.06609691637907515183, -0.06416707940450361303, -0.06223724242993208117, -0.06030740545536053543, -0.05789510923714611540, -0.05548281301893168843, -0.05355297604436015657, -0.05162313906978862471, -0.04921084285157419774, -0.04631608738971689648, -0.04342133192785958135, -0.04052657646600228009, -0.03763182100414497189, -0.03521952478593055186, -0.03328968781135902000, -0.03184231008043036937, -0.03039493234950170833, -0.02846509537493017647, -0.02605279915671574950, -0.02364050293850132947, -0.02171066596392979067, -0.01978082898935825881, -0.01785099201478672001, -0.01592115504021518121, -0.01399131806564364588, -0.01157902184742922412, -0.008684266385571917657, -0.005789510923714612060, -0.002894755461857306030, 0.000000000000000000 ),
 .UNSPECIFIED. ) ;
#21777=CYLINDRICAL_SURFACE ( 'NONE', #8471, 9.804803391925412726 ) ;
#21780=CARTESIAN_POINT ( 'NONE',  ( 33.89795617549800255, -5.470764165105774346, -0.4365038096981310733 ) ) ;
#21781=CARTESIAN_POINT ( 'NONE',  ( 21.73635333206707543, 6.105328942885613230, -3.274543301268284523 ) ) ;
#21782=ORIENTED_EDGE ( 'NONE', *, *, #40033, .T. ) ;
#21784=CARTESIAN_POINT ( 'NONE',  ( 24.65869693034278143, -1.551691026114866201, -6.728867248637652843 ) ) ;
#21786=CARTESIAN_POINT ( 'NONE',  ( -80.35141725551916636, -6.644025400410976445, -3.371800178188818276 ) ) ;
#21789=CARTESIAN_POINT ( 'NONE',  ( 88.12503612275229159, -2.065192647045405838, -2.806263388478303256 ) ) ;
#21793=CARTESIAN_POINT ( 'NONE',  ( 21.53928041017985251, 7.378620751039662196, -0.9880446992327728273 ) ) ;
#21794=ORIENTED_EDGE ( 'NONE', *, *, #11986, .T. ) ;
#21796=CARTESIAN_POINT ( 'NONE',  ( 14.74464696855122980, -5.058300963987686139, -2.496493677045212856 ) ) ;
#21800=CARTESIAN_POINT ( 'NONE',  ( 27.40614744282377657, 0.9610282265797985835, 4.483790147270008575 ) ) ;
#21801=CARTESIAN_POINT ( 'NONE',  ( -70.92837670882107659, -56.35932253828835314, 6.000000000000002665 ) ) ;
#21802=VERTEX_POINT ( 'NONE', #37066 ) ;
#21804=DIRECTION ( 'NONE',  ( 0.000000000000000000, -0.000000000000000000, -1.000000000000000000 ) ) ;
#21811=AXIS2_PLACEMENT_3D ( 'NONE', #24897, #25305, #25504 ) ;
#21814=CARTESIAN_POINT ( 'NONE',  ( 33.46455515056310759, -3.089188617792877789, 5.429351193206847448 ) ) ;
#21816=CARTESIAN_POINT ( 'NONE',  ( 23.15206694985459634, 2.717029284607917372, 4.326704671169357752 ) ) ;
#21817=CARTESIAN_POINT ( 'NONE',  ( 36.08990603727164626, -1.513213400165028810, 5.635049790240730161 ) ) ;
#21822=CARTESIAN_POINT ( 'NONE',  ( -69.92837670882109080, -0.6506954850797312950, 5.916079783099628564 ) ) ;
#21823=FACE_OUTER_BOUND ( 'NONE', #39800, .T. ) ;
#21827=EDGE_LOOP ( 'NONE', ( #36771, #29625, #34799, #4704 ) ) ;
#21828=CARTESIAN_POINT ( 'NONE',  ( 23.25171722262629359, 3.194370665195247483, -3.902736047147622234 ) ) ;
#21831=CARTESIAN_POINT ( 'NONE',  ( 21.85643539959779957, -14.30241103581959727, -6.272691714111175543 ) ) ;
#21832=CARTESIAN_POINT ( 'NONE',  ( 17.10505430645456926, 14.50076029598319849, 3.172244300429228225 ) ) ;
#21833=VERTEX_POINT ( 'NONE', #23892 ) ;
#21834=AXIS2_PLACEMENT_3D ( 'NONE', #24790, #9326, #19018 ) ;
#21835=ORIENTED_EDGE ( 'NONE', *, *, #38488, .F. ) ;
#21836=CARTESIAN_POINT ( 'NONE',  ( 37.19747299874393320, -2.841585884120807481, 5.999818732555961098 ) ) ;
#21838=CARTESIAN_POINT ( 'NONE',  ( 86.99908277331161344, 0.6362256001576577225, -5.325422653610870860 ) ) ;
#21842=CARTESIAN_POINT ( 'NONE',  ( 14.80252671224570271, -4.520290230480198623, 2.514186659199406204 ) ) ;
#21844=CARTESIAN_POINT ( 'NONE',  ( 36.64694695204426722, -2.460141890980504620, -5.926040400264396268 ) ) ;
#21846=DIRECTION ( 'NONE',  ( 1.000000000000000000, 0.000000000000000000, 0.000000000000000000 ) ) ;
#21849=ORIENTED_EDGE ( 'NONE', *, *, #36261, .T. ) ;
#21851=CARTESIAN_POINT ( 'NONE',  ( 36.88753254950347582, -3.349785859984652614, 5.911062257491906280 ) ) ;
#21854=CARTESIAN_POINT ( 'NONE',  ( 86.43572624768425783, -0.5192074800720990480, -5.777013305174518720 ) ) ;
#21856=ORIENTED_EDGE ( 'NONE', *, *, #39341, .T. ) ;
#21858=CARTESIAN_POINT ( 'NONE',  ( -74.21080977438080595, 8.885293297773669607, -9.447016131426053676 ) ) ;
#21864=CARTESIAN_POINT ( 'NONE',  ( 24.36694571186475144, 3.146468230158969703, 3.351613297348657650 ) ) ;
#21873=CARTESIAN_POINT ( 'NONE',  ( 16.45937104885421931, 9.965318428467051959, -2.758229892786640214 ) ) ;
#21878=DIRECTION ( 'NONE',  ( -0.9999026450364576490, -0.01395351027862084224, 0.000000000000000000 ) ) ;
#21884=CARTESIAN_POINT ( 'NONE',  ( 28.96592479936138176, -0.01829609152130128036, -5.755841479376210934 ) ) ;
#21893=CARTESIAN_POINT ( 'NONE',  ( 33.04859423313239830, -0.2660396992994370491, -5.100192512784728294 ) ) ;
#21905=EDGE_CURVE ( 'NONE', #4105, #25100, #37725, .T. ) ;
#21918=CARTESIAN_POINT ( 'NONE',  ( 21.82942332946822361, 5.970316737997020340, 3.131952444615608844 ) ) ;
#21920=CARTESIAN_POINT ( 'NONE',  ( 18.42522192648813828, -3.123253340230073061, 3.033926698805842648 ) ) ;
#21922=EDGE_CURVE ( 'NONE', #9338, #23233, #38085, .T. ) ;
#21923=ORIENTED_EDGE ( 'NONE', *, *, #38805, .F. ) ;
#21925=CARTESIAN_POINT ( 'NONE',  ( 22.65837895044245798, 0.3099126875621054378, 6.437328739972214109 ) ) ;
#21933=CARTESIAN_POINT ( 'NONE',  ( 21.85643539959779957, -10.54057479330554159, -5.012605957032298498 ) ) ;
#21934=LINE ( 'NONE', #6284, #25299 ) ;
#21936=CARTESIAN_POINT ( 'NONE',  ( -72.92592677944759316, 1.059812494767570668, 9.858470738818239099 ) ) ;
#21937=CARTESIAN_POINT ( 'NONE',  ( 36.50792169068728299, -3.548421012104517658, 5.802103936190841083 ) ) ;
#21944=CARTESIAN_POINT ( 'NONE',  ( 21.74105148488215988, 4.237279870184942787, -2.792868468085587530 ) ) ;
#21947=CARTESIAN_POINT ( 'NONE',  ( 20.06265332725812556, 6.856321025424916726, 3.229911059913491478 ) ) ;
#21954=CARTESIAN_POINT ( 'NONE',  ( 23.14765463162058623, 0.4541928285590982606, -5.841642121512133023 ) ) ;
#21955=CARTESIAN_POINT ( 'NONE',  ( 29.53970505027308491, -3.873674039035061689, -4.297879082457085609 ) ) ;
#21956=CARTESIAN_POINT ( 'NONE',  ( 24.80520132849324710, 2.592517504530978290, -3.945774167130594812 ) ) ;
#21957=EDGE_LOOP ( 'NONE', ( #556, #18025, #30132, #14387, #20780, #39554, #24901 ) ) ;
#21961=CARTESIAN_POINT ( 'NONE',  ( 20.53310891050050557, 3.934803127027559189, 3.411086259235923457 ) ) ;
#21966=CARTESIAN_POINT ( 'NONE',  ( 86.86785128967072467, -0.4505172232112327757, -5.755800129507335328 ) ) ;
#21967=CARTESIAN_POINT ( 'NONE',  ( 35.63404480038042976, -3.169100885857628391, -5.767952522366300627 ) ) ;
#21969=CARTESIAN_POINT ( 'NONE',  ( 26.04389118395324587, 1.945336293897782287, 4.218032799664143795 ) ) ;
#21973=LINE ( 'NONE', #28339, #9719 ) ;
#21985=CARTESIAN_POINT ( 'NONE',  ( 24.80613193118815474, -5.883788488468095323, 2.846725823111817100 ) ) ;
#21986=CARTESIAN_POINT ( 'NONE',  ( -71.54191492143920073, -21.58360693942124797, 9.981599438687137393 ) ) ;
#21988=CARTESIAN_POINT ( 'NONE',  ( 21.71920171916170261, 6.265005891781191494, -3.215796620455622090 ) ) ;
#21992=CARTESIAN_POINT ( 'NONE',  ( -80.83685820618015327, -6.606126994342639946, -1.409722980286805427 ) ) ;
#21996=CARTESIAN_POINT ( 'NONE',  ( 87.44477293306643162, -1.228341977218806447, 4.926563918429203603 ) ) ;
#21998=ORIENTED_EDGE ( 'NONE', *, *, #22799, .T. ) ;
#22003=DIRECTION ( 'NONE',  ( -0.000000000000000000, 0.000000000000000000, 1.000000000000000000 ) ) ;
#22008=CARTESIAN_POINT ( 'NONE',  ( 36.79751133535093288, -2.556301215552558848, 5.949539613692945039 ) ) ;
#22009=EDGE_CURVE ( 'NONE', #40651, #25150, #9467, .T. ) ;
#22011=CARTESIAN_POINT ( 'NONE',  ( 87.46579090913228072, 0.1119968706995537605, 4.710562776971725540 ) ) ;
#22016=CARTESIAN_POINT ( 'NONE',  ( 14.71881405247904340, 13.02603684036817633, -2.499237524637579533 ) ) ;
#22018=CARTESIAN_POINT ( 'NONE',  ( 25.30743677325165208, -5.496855584100603487, -2.999765155844900555 ) ) ;
#22023=VERTEX_POINT ( 'NONE', #4136 ) ;
#22025=CARTESIAN_POINT ( 'NONE',  ( -62.92837670882106238, 13.37661300689599742, 6.000000000000000000 ) ) ;
#22026=CARTESIAN_POINT ( 'NONE',  ( 22.65299298941167550, 3.119508358272978121, 4.311559539158433374 ) ) ;
#22027=CARTESIAN_POINT ( 'NONE',  ( -12.99139449055068241, 13.37661300689600097, -2.500000000000000444 ) ) ;
#22032=CARTESIAN_POINT ( 'NONE',  ( 85.88576331275629627, 1.886758859582599479, -4.135933360337332942 ) ) ;
#22034=CARTESIAN_POINT ( 'NONE',  ( -71.92837670882107659, -20.78299143688747819, 5.916079783099617906 ) ) ;
#22037=CARTESIAN_POINT ( 'NONE',  ( 23.02787331254640790, 3.347463497797338761, -3.909392201422248192 ) ) ;
#22040=CARTESIAN_POINT ( 'NONE',  ( 21.85643539959774273, 10.29907807357824723, -3.463423532579224418 ) ) ;
#22042=ORIENTED_EDGE ( 'NONE', *, *, #13134, .F. ) ;
#22046=CARTESIAN_POINT ( 'NONE',  ( 85.25019696446999262, 2.600657147776545663, -2.704904232406868836 ) ) ;
#22050=CARTESIAN_POINT ( 'NONE',  ( 14.96872153645507630, -6.096775576253210538, 2.530506653653641802 ) ) ;
#22051=CARTESIAN_POINT ( 'NONE',  ( 36.79872796904915333, -2.554582093385345587, -5.949729498805945482 ) ) ;
#22054=DIRECTION ( 'NONE',  ( 1.682730792515357087E-16, -1.000000000000000000, 0.000000000000000000 ) ) ;
#22062=CARTESIAN_POINT ( 'NONE',  ( 30.88230511604370676, 0.6976464429761185526, 4.494867301746904076 ) ) ;
#22070=VECTOR ( 'NONE', #29007, 1000.000000000000000 ) ;
#22071=CARTESIAN_POINT ( 'NONE',  ( 88.35313037274487158, -0.8847049305017679055, 0.4761908919756944747 ) ) ;
#22072=CARTESIAN_POINT ( 'NONE',  ( -73.13897352737927804, -2.605432823423965871, -9.755499191730667263 ) ) ;
#22077=CARTESIAN_POINT ( 'NONE',  ( 22.64664158185920328, 4.505184941302465162, 3.155068566400609065 ) ) ;
#22086=CARTESIAN_POINT ( 'NONE',  ( 15.93752674114121071, 10.76136407783234361, -2.654679014335209253 ) ) ;
#22095=CARTESIAN_POINT ( 'NONE',  ( 27.76889013493211067, -0.3210463222110187531, 6.029547961152755597 ) ) ;
#22097=CARTESIAN_POINT ( 'NONE',  ( 25.22231346541800434, -5.090807757912027220, 2.500000000020063506 ) ) ;
#22101=CARTESIAN_POINT ( 'NONE',  ( -70.92837670882107659, -39.37473357531882101, 0.000000000000000000 ) ) ;
#22105=CARTESIAN_POINT ( 'NONE',  ( 35.70151715991190855, -1.358511810577603063, -5.583808527359176210 ) ) ;
#22108=CARTESIAN_POINT ( 'NONE',  ( 14.60824295769313963, -5.049561965150513920, -2.486367633875753658 ) ) ;
#22112=B_SPLINE_CURVE_WITH_KNOTS ( 'NONE', 3,
 ( #20477, #16260, #32144, #40612, #16853, #29435, #25945, #38479, #26352, #23258, #9318, #12417, #29235, #23060, #16647, #19359, #7399, #1043, #31930, #34473, #35625, #1247, #38884, #24988, #32338, #3737, #28832, #31168 ),
 .UNSPECIFIED., .F., .F.,
 ( 4, 2, 2, 1, 1, 1, 2, 2, 2, 2, 1, 1, 1, 2, 2, 2, 4 ),
 ( 0.000000000000000000, 0.1250000000000915101, 0.1875000000001351974, 0.2187500000001550426, 0.2343750000001629530, 0.2421875000001669220, 0.2460937500001669498, 0.2500000000001669775, 0.3750000000001321165, 0.4375000000001147415, 0.4687500000001080247, 0.4843750000001036948, 0.4921875000001015299, 0.4960937500001013634, 0.5000000000001012523, 0.7500000000000506262, 1.000000000000000000 ),
 .UNSPECIFIED. ) ;
#22114=CARTESIAN_POINT ( 'NONE',  ( 21.97379874220277429, -12.00982949064745320, 2.500000000000000444 ) ) ;
#22118=FACE_BOUND ( 'NONE', #28227, .T. ) ;
#22124=CARTESIAN_POINT ( 'NONE',  ( 23.73727407787542987, 2.939497050369670017, 3.908896929995592018 ) ) ;
#22129=CARTESIAN_POINT ( 'NONE',  ( 23.43597607405129679, 3.793424526424878263, 3.103042028786229700 ) ) ;
#22136=CARTESIAN_POINT ( 'NONE',  ( 24.12362351582647335, 0.5386221531753900837, 5.092127627954526226 ) ) ;
#22144=CARTESIAN_POINT ( 'NONE',  ( 22.31814515643556263, 6.191369071892208531, -1.397765879422002033 ) ) ;
#22146=ORIENTED_EDGE ( 'NONE', *, *, #15774, .F. ) ;
#22147=CARTESIAN_POINT ( 'NONE',  ( -76.51899586397401265, 9.210917537453957138, 9.782013801987098134 ) ) ;
#22148=CARTESIAN_POINT ( 'NONE',  ( 36.12715512229904391, -3.661643169911928730, 5.700734919021059888 ) ) ;
#22150=EDGE_CURVE ( 'NONE', #31898, #9007, #35783, .T. ) ;
#22153=CARTESIAN_POINT ( 'NONE',  ( 32.01236844922196667, -2.960126844666696844, -5.202702337194527793 ) ) ;
#22154=CARTESIAN_POINT ( 'NONE',  ( 33.68512006240106871, -3.841534318799366687, -5.136340396096415795 ) ) ;
#22158=CARTESIAN_POINT ( 'NONE',  ( -61.24591834330252027, 3.729367930467589076, -2.500000000000000000 ) ) ;
#22162=CARTESIAN_POINT ( 'NONE',  ( 25.85639891750619412, 1.591965851834448165, -4.299200647184679092 ) ) ;
#22163=CARTESIAN_POINT ( 'NONE',  ( 21.85643539959776760, 1.710603452083953179E-15, -2.500000000000000000 ) ) ;
#22170=CARTESIAN_POINT ( 'NONE',  ( 34.76605832449826750, -3.465236551535387566, 5.619590712300242430 ) ) ;
#22174=CARTESIAN_POINT ( 'NONE',  ( 84.58609069645564205, 2.764543530557054041, -2.886136738505205912 ) ) ;
#22175=CARTESIAN_POINT ( 'NONE',  ( 36.06197813380387629, -3.149146827136996674, -5.834741868653807728 ) ) ;
#22176=ORIENTED_EDGE ( 'NONE', *, *, #18496, .T. ) ;
#22177=CARTESIAN_POINT ( 'NONE',  ( 24.39369049594943206, 2.947980553390389780, 3.706541376397575860 ) ) ;
#22183=B_SPLINE_SURFACE_WITH_KNOTS ( 'NONE', 5, 3, ( 
 ( #9051, #27591, #15848, #5977, #28405, #24293, #2913, #6183, #12551, #2711, #15233, #37653, #18942, #34208, #18517, #27786, #11719, #15646, #9455, #40341, #27994, #30698, #21831, #34617, #34410, #36856, #12134, #31307, #15028, #21425, #40142, #18726, #31103, #3331, #25122, #24501, #6392, #18105, #33999, #8640, #3129, #5564, #28193, #5775, #24921, #21215, #11924 ),
 ( #21, #33786, #22040, #37053, #12349, #15433, #40538, #37456, #31508, #2504, #8839, #18312, #30902, #24711, #37259, #9252, #21628, #425, #16843, #35220, #25331, #25729, #35422, #38672, #7387, #34823, #827, #12964, #25530, #213, #37866, #22653, #6598, #16638, #23051, #35616, #38075, #3933, #10271, #32327, #19348, #6991, #19144, #28617, #13359, #26140, #25934 ),
 ( #22256, #9669, #31709, #29024, #13568, #9876, #7190, #19558, #22450, #19943, #19750, #32134, #29222, #10471, #3525, #38467, #22849, #32522, #4125, #28823, #4321, #16449, #12753, #1034, #35019, #16049, #6794, #31917, #3728, #16252, #627, #13170, #38273, #10068, #1432, #39680, #29814, #39473, #38874, #26533, #5110, #13965, #11064, #11259, #1838, #26736, #7980 ),
 ( #23634, #39272, #17645, #30225, #29425, #14162, #10666, #26930, #1626, #17241, #39067, #36201, #8382, #4901, #8173, #20534, #35813, #7588, #17038, #20143, #10866, #33120, #11463, #24031, #2040, #14359, #23443, #17433, #23246, #14555, #20337, #23825, #36401, #27130, #20957, #32723, #30021, #4518, #7787, #20743, #1239, #36008, #33333, #29615, #32916, #36604, #33540 ),
 ( #5313, #4708, #13774, #26342, #14761, #12081, #24242, #34363, #40702, #25076, #14980, #21581, #27942, #21784, #21370, #24657, #11668, #5514, #18468, #15596, #2863, #34568, #15387, #39894, #27332, #36805, #40484, #31260, #18056, #12297, #34162, #11872, #37608, #24870, #37409, #6133, #27738, #21168, #2458, #28148, #18672, #27540, #17849, #33948, #30431, #33734, #24449 ),
 ( #2241, #5724, #30854, #2661, #15180, #6448, #38320, #22902, #9725, #3979, #3780, #31763, #32376, #16498, #28873, #25988, #19403, #19001, #34873, #35470, #19608, #37918, #16107, #19805, #38125, #7242, #16304, #19199, #10117, #38520, #679, #3579, #22306, #6845, #25379, #13621, #13220, #26195, #22095, #25786, #29075, #10325, #478, #13017, #4174, #16690, #31975 ),
 ( #9513, #13413, #29277, #25580, #22705, #28461, #32182, #1089, #882, #34670, #9927, #31561, #12808, #28672, #6649, #3384, #35273, #15900, #268, #22509, #35073, #7040, #20195, #35669, #33177, #32580, #30083, #32781, #11122, #2096, #1290, #11317, #20802, #1898, #10523, #23883, #10718, #39332, #20393, #32975, #23691, #20592, #17490, #4964, #4375, #38926, #13827 ),
 ( #36456, #23297, #14612, #4760, #23102, #23500, #14420, #8231, #5167, #16897, #36257, #35868, #7646, #38727, #7438, #17294, #29477, #26988, #33395, #17703, #4570, #1688, #8034, #26396, #39535, #30281, #19998, #17097, #14218, #29670, #1482, #14016, #29872, #26588, #39127, #10924, #36067, #7845, #26793, #40346, #8437, #24090, #36658, #15238, #379, #27388, #21636 ) ),
 .UNSPECIFIED., .F., .T., .F.,
 ( 6, 2, 6 ),
 ( 4, 1, 1, 1, 1, 1, 1, 1, 1, 1, 1, 1, 1, 1, 1, 1, 1, 1, 1, 1, 1, 1, 1, 1, 1, 1, 1, 1, 1, 1, 1, 1, 1, 1, 1, 1, 1, 1, 1, 1, 1, 1, 1, 1, 4 ),
 ( 0.000000000000000000, 0.5000000000000000000, 1.000000000000000000 ),
 ( -0.09263217477943377909, -0.08973741931757646395, -0.08732512309936206474, -0.08539528612479052594, -0.08394790839386186143, -0.08250053066293322468, -0.08105315293200456017, -0.07960577520107590954, -0.07815839747014724503, -0.07671101973921859440, -0.07478118276464705561, -0.07285134579007553068, -0.07092150881550399188, -0.06947413108457534126, -0.06802675335364669063, -0.06609691637907515183, -0.06416707940450361303, -0.06223724242993208117, -0.06030740545536053543, -0.05789510923714611540, -0.05548281301893168843, -0.05355297604436015657, -0.05162313906978862471, -0.04921084285157419774, -0.04631608738971689648, -0.04342133192785958135, -0.04052657646600228009, -0.03763182100414497189, -0.03521952478593055186, -0.03328968781135902000, -0.03184231008043036937, -0.03039493234950170833, -0.02846509537493017647, -0.02605279915671574950, -0.02364050293850132947, -0.02171066596392979067, -0.01978082898935825881, -0.01785099201478672001, -0.01592115504021518121, -0.01399131806564364588, -0.01157902184742922412, -0.008684266385571917657, -0.005789510923714612060, -0.002894755461857306030, 0.000000000000000000 ),
 .UNSPECIFIED. ) ;
#22188=CARTESIAN_POINT ( 'NONE',  ( 14.66504043345067032, 12.84305297963125270, 2.500000000000000000 ) ) ;
#22199=CARTESIAN_POINT ( 'NONE',  ( 21.99661976377250738, 5.574053075156116144, -3.114055112780370838 ) ) ;
#22206=CARTESIAN_POINT ( 'NONE',  ( -79.87304265776585055, -6.650848427980711186, -4.489763987400060330 ) ) ;
#22209=CARTESIAN_POINT ( 'NONE',  ( 84.21365554304541945, 2.879787869890822360, 1.939519519617897592 ) ) ;
#22213=CARTESIAN_POINT ( 'NONE',  ( 24.90937036835209639, 3.542633436675763026, 0.6500615448964709442 ) ) ;
#22217=CARTESIAN_POINT ( 'NONE',  ( 85.57702991149881200, 1.013049332619667009, 5.784095605458488443 ) ) ;
#22218=CARTESIAN_POINT ( 'NONE',  ( 20.42385195123408081, 3.665137036896844336, 3.394034068352853151 ) ) ;
#22220=CARTESIAN_POINT ( 'NONE',  ( 87.15505355144220800, 0.4610318193416703680, -5.246243280819175681 ) ) ;
#22223=CARTESIAN_POINT ( 'NONE',  ( -61.57369240569498459, -49.47615685354814019, 3.769463484964754141 ) ) ;
#22225=CARTESIAN_POINT ( 'NONE',  ( -70.73088139374260663, -45.62685287453590632, 9.998512938616805457 ) ) ;
#22230=EDGE_CURVE ( 'NONE', #25100, #4684, #2351, .T. ) ;
#22232=CARTESIAN_POINT ( 'NONE',  ( 0.7201709579117279159, -51.60714625320436255, -6.000000000000000000 ) ) ;
#22233=ORIENTED_EDGE ( 'NONE', *, *, #38073, .F. ) ;
#22236=B_SPLINE_CURVE_WITH_KNOTS ( 'NONE', 3,
 ( #24724, #2932, #31117, #27803, #5996, #37279 ),
 .UNSPECIFIED., .F., .F.,
 ( 4, 2, 4 ),
 ( 0.000000000000000000, 0.0004173165775082530657, 0.0008346331550165061314 ),
 .UNSPECIFIED. ) ;
#22237=CARTESIAN_POINT ( 'NONE',  ( 36.65031935333231417, -3.107300908937615347, 5.926566745047386675 ) ) ;
#22238=CARTESIAN_POINT ( 'NONE',  ( 22.26980982591663505, 1.689402514127164912, 5.821894515090187738 ) ) ;
#22239=CARTESIAN_POINT ( 'NONE',  ( 36.60019281065275720, -1.851694985322541287, 5.780171978738543714 ) ) ;
#22241=ORIENTED_EDGE ( 'NONE', *, *, #13990, .F. ) ;
#22252=CARTESIAN_POINT ( 'NONE',  ( 21.84320482927419604, 4.475403957759267470, -4.050769160178117723 ) ) ;
#22256=CARTESIAN_POINT ( 'NONE',  ( 21.85643539959774273, 9.214175136349357587, -0.8338435668127727185 ) ) ;
#22259=CARTESIAN_POINT ( 'NONE',  ( 85.23697547898807159, 2.562304445728192714, -3.499295437968926947 ) ) ;
#22260=ORIENTED_EDGE ( 'NONE', *, *, #36036, .T. ) ;
#22263=CARTESIAN_POINT ( 'NONE',  ( 18.24487163080560492, -2.878841870252593527, 3.053951490511794375 ) ) ;
#22264=CARTESIAN_POINT ( 'NONE',  ( 36.19390568488644533, -2.232540992349622222, -5.855332353680082313 ) ) ;
#22270=CARTESIAN_POINT ( 'NONE',  ( 30.76274491791073018, -3.760333558979258139, 4.555209097832164211 ) ) ;
#22272=CARTESIAN_POINT ( 'NONE',  ( 33.45655213939275541, -3.830548352551304880, 5.092536695668412605 ) ) ;
#22273=AXIS2_PLACEMENT_3D ( 'NONE', #12405, #27639, #9512 ) ;
#22277=EDGE_LOOP ( 'NONE', ( #15921, #32348, #7152, #4880 ) ) ;
#22278=CARTESIAN_POINT ( 'NONE',  ( 87.80056509578477630, -0.2640373850900027408, -3.668630654083185672 ) ) ;
#22279=CARTESIAN_POINT ( 'NONE',  ( -80.92837670882107659, 2.429809908903242555, -12.50000000000000000 ) ) ;
#22280=LINE ( 'NONE', #454, #16264 ) ;
#22281=ORIENTED_EDGE ( 'NONE', *, *, #17136, .T. ) ;
#22284=ORIENTED_EDGE ( 'NONE', *, *, #16004, .T. ) ;
#22285=CARTESIAN_POINT ( 'NONE',  ( 22.04813532460007863, 5.340643346204053898, 3.227846874785398779 ) ) ;
#22293=CARTESIAN_POINT ( 'NONE',  ( 15.30597500999765259, 11.49007520356607692, -2.585737325345484727 ) ) ;
#22300=ADVANCED_FACE ( 'NONE', ( #19583, #37680 ), #7018, .T. ) ;
#22305=CARTESIAN_POINT ( 'NONE',  ( 18.79220209723194301, 6.725183318188751258, 3.484773800353550222 ) ) ;
#22306=CARTESIAN_POINT ( 'NONE',  ( 29.52151182519568096, -2.704869923190903691, 5.373754524306347591 ) ) ;
#22312=CARTESIAN_POINT ( 'NONE',  ( 11.29080664838498826, -10.90558813203967148, -2.500000000000000000 ) ) ;
#22314=CARTESIAN_POINT ( 'NONE',  ( 34.77014988848376476, -3.601456801931015139, -5.565767284829528094 ) ) ;
#22315=CARTESIAN_POINT ( 'NONE',  ( -69.42837670882107659, -47.11702805680359063, 9.886859966642603581 ) ) ;
#22319=CARTESIAN_POINT ( 'NONE',  ( -81.75358215887496272, 10.46790825574969119, 1.500190250375194712 ) ) ;
#22325=ORIENTED_EDGE ( 'NONE', *, *, #22395, .F. ) ;
#22332=CARTESIAN_POINT ( 'NONE',  ( 22.63675764000105772, 3.280949574944325153, 4.200075021517235108 ) ) ;
#22337=CARTESIAN_POINT ( 'NONE',  ( 21.99022176547038399, 5.605367161166800116, 3.096869486298271745 ) ) ;
#22341=CARTESIAN_POINT ( 'NONE',  ( -70.92837670882107659, -56.35932253828836025, 0.000000000000000000 ) ) ;
#22344=CARTESIAN_POINT ( 'NONE',  ( 22.01703001042701757, 0.2566429920367864215, 7.603351845833338452 ) ) ;
#22350=ADVANCED_FACE ( 'NONE', ( #25761 ), #18972, .F. ) ;
#22353=CARTESIAN_POINT ( 'NONE',  ( 24.65869693034278143, -1.551691026114866201, -6.728867248637652843 ) ) ;
#22356=CARTESIAN_POINT ( 'NONE',  ( -76.30046984573570512, 10.53876514546700527, 8.436514736823731653 ) ) ;
#22357=CARTESIAN_POINT ( 'NONE',  ( 27.44646592037410215, 0.9065689399580380003, -4.490082820797807628 ) ) ;
#22360=CARTESIAN_POINT ( 'NONE',  ( -80.91149519099745646, 11.45826392489275136, -0.9973769203057932797 ) ) ;
#22361=CIRCLE ( 'NONE', #20350, 12.73502530973474300 ) ;
#22362=CARTESIAN_POINT ( 'NONE',  ( 30.73690320840939094, -3.644613918395323893, -4.722495812001631599 ) ) ;
#22363=CARTESIAN_POINT ( 'NONE',  ( 32.06850821402472462, 0.2517114437988486331, -4.728941223353197998 ) ) ;
#22364=PLANE ( 'NONE',  #40014 ) ;
#22365=CARTESIAN_POINT ( 'NONE',  ( 15.85770990068897568, 10.71461798967161627, 2.668183247020202042 ) ) ;
#22370=CARTESIAN_POINT ( 'NONE',  ( 29.68316414800138858, 1.144177792258728843, -4.265623084207747162 ) ) ;
#22373=B_SPLINE_CURVE_WITH_KNOTS ( 'NONE', 3,
 ( #9949, #32603, #3605, #19427, #34899, #35494, #1116, #13648, #16131, #7263, #29503, #28695, #38752, #7465, #26220, #37944, #10546, #22532, #26015, #7063, #4005, #506, #31998, #13041 ),
 .UNSPECIFIED., .F., .F.,
 ( 4, 2, 2, 2, 2, 2, 2, 2, 2, 2, 2, 4 ),
 ( 0.000000000000000000, 0.1249999999999756028, 0.1874999999999667211, 0.2187499999999662770, 0.2499999999999658051, 0.3749999999999674150, 0.3906249999999655831, 0.4062499999999636957, 0.4374999999999693578, 0.4999999999999727995, 0.7499999999999863443, 1.000000000000000000 ),
 .UNSPECIFIED. ) ;
#22376=AXIS2_PLACEMENT_3D ( 'NONE', #12693, #27724, #8774 ) ;
#22378=CARTESIAN_POINT ( 'NONE',  ( 85.17963886742116131, 2.035184340541872139, -4.783483324554544502 ) ) ;
#22380=VERTEX_POINT ( 'NONE', #16278 ) ;
#22381=CARTESIAN_POINT ( 'NONE',  ( 24.37965766804015288, 2.942655792175109308, 3.717632330914962147 ) ) ;
#22382=DIRECTION ( 'NONE',  ( 1.000000000000000000, 0.000000000000000000, 0.000000000000000000 ) ) ;
#22390=DIRECTION ( 'NONE',  ( -0.000000000000000000, -1.000000000000000000, -0.000000000000000000 ) ) ;
#22392=DIRECTION ( 'NONE',  ( -0.000000000000000000, -0.000000000000000000, 1.000000000000000000 ) ) ;
#22395=EDGE_CURVE ( 'NONE', #28485, #34557, #27932, .T. ) ;
#22398=CARTESIAN_POINT ( 'NONE',  ( 21.85643539959778536, -9.383538770078029501, -13.42257110913290141 ) ) ;
#22399=CARTESIAN_POINT ( 'NONE',  ( 22.19935042935221858, 5.213326102501693704, -3.111963524547389781 ) ) ;
#22407=CARTESIAN_POINT ( 'NONE',  ( 88.05006142693602555, -2.316660831613085225, -1.868938639203592489 ) ) ;
#22414=CARTESIAN_POINT ( 'NONE',  ( 24.75830837035764276, 3.019210359990082804, 3.350572556515618583 ) ) ;
#22417=CARTESIAN_POINT ( 'NONE',  ( 37.04329737603605111, -2.892586564141972350, 5.987900469699707351 ) ) ;
#22419=CARTESIAN_POINT ( 'NONE',  ( 85.49511565994269802, 2.325552844478905090, -3.343772400554256397 ) ) ;
#22420=VERTEX_POINT ( 'NONE', #858 ) ;
#22422=CARTESIAN_POINT ( 'NONE',  ( 14.77500745536057813, -5.175466302041957789, 2.500000552286355759 ) ) ;
#22424=CARTESIAN_POINT ( 'NONE',  ( -69.42837670882106238, -47.01908264895750023, 9.886859966642600028 ) ) ;
#22431=CARTESIAN_POINT ( 'NONE',  ( -76.50596395675130168, -5.795592924334072471, 8.309263729044971569 ) ) ;
#22435=CARTESIAN_POINT ( 'NONE',  ( 22.24790050656625695, 1.172224622543360129, 6.341858785536460985 ) ) ;
#22439=AXIS2_PLACEMENT_3D ( 'NONE', #28380, #21804, #21602 ) ;
#22443=CARTESIAN_POINT ( 'NONE',  ( 86.40625215706664619, 1.302121085762450114, 4.853768006845460725 ) ) ;
#22447=CARTESIAN_POINT ( 'NONE',  ( 23.19876663987166054, 3.510391698098890956, -3.664004875277358408 ) ) ;
#22450=CARTESIAN_POINT ( 'NONE',  ( 21.85643539959779602, 4.838159542671753854, -10.55000746994157979 ) ) ;
#22451=CARTESIAN_POINT ( 'NONE',  ( 21.85643539961850479, 4.025506921146978279, 3.384544483176039620 ) ) ;
#22452=ORIENTED_EDGE ( 'NONE', *, *, #19028, .F. ) ;
#22455=CARTESIAN_POINT ( 'NONE',  ( 87.65094362820954643, -0.09597545124639318692, -4.742286025697146634 ) ) ;
#22460=CARTESIAN_POINT ( 'NONE',  ( 17.10475337451625322, -3.043619170508630400, 2.876008462753611994 ) ) ;
#22461=CARTESIAN_POINT ( 'NONE',  ( 31.71966209317523422, -0.5565497988919112515, -5.157018431203386655 ) ) ;
#22469=CARTESIAN_POINT ( 'NONE',  ( 28.74930798315838132, -3.747080672683058555, 4.540790173945463692 ) ) ;
#22472=CARTESIAN_POINT ( 'NONE',  ( 37.10898288256137079, -2.404723019174210830, 5.951907613904549699 ) ) ;
#22489=CARTESIAN_POINT ( 'NONE',  ( 23.42158288118685050, 3.688889536555259419, 3.302951128627464872 ) ) ;
#22498=CARTESIAN_POINT ( 'NONE',  ( 19.86836432286185783, 6.624182616967236648, -3.307336789426305934 ) ) ;
#22501=ORIENTED_EDGE ( 'NONE', *, *, #1551, .T. ) ;
#22503=FACE_OUTER_BOUND ( 'NONE', #4773, .T. ) ;
#22508=CARTESIAN_POINT ( 'NONE',  ( 18.26922817967627921, 11.64739335993193947, 2.499999999999998668 ) ) ;
#22509=CARTESIAN_POINT ( 'NONE',  ( 31.64923038865762805, -3.528005414130610529, -5.019302312848182623 ) ) ;
#22515=CARTESIAN_POINT ( 'NONE',  ( 36.78040056622536014, -2.229284608445112781, -5.922136277988401254 ) ) ;
#22521=CARTESIAN_POINT ( 'NONE',  ( 22.23218040091930092, -10.39938183745549694, -2.500000000000000000 ) ) ;
#22522=CARTESIAN_POINT ( 'NONE',  ( 21.87789367320688072, -13.40669691499416061, 2.499999999999999556 ) ) ;
#22524=B_SPLINE_SURFACE_WITH_KNOTS ( 'NONE', 5, 3, ( 
 ( #36759, #1581, #14112, #17805, #30390, #33692, #36965, #11015, #8744, #21328, #39226, #36160, #33073, #4857, #39426, #29971, #1786, #11216, #9573, #18219, #2616, #31211, #9781, #40441, #28311, #25031, #12250, #15340, #24822, #15550, #6505, #37166, #21944, #3240 ),
 ( #34517, #22154, #37566, #27895, #5887, #3032, #8951, #37976, #28104, #33903, #5677, #9361, #129, #34726, #37367, #9163, #19054, #328, #40659, #12461, #21737, #30811, #37767, #31617, #34318, #6294, #12033, #15757, #15956, #15135, #18842, #27691, #6088, #12660 ),
 ( #18622, #31412, #25236, #3440, #21537, #28518, #12868, #25433, #40247, #24611, #34115, #18423, #31011, #2816, #22560, #13074, #1150, #35125, #38578, #16958, #13472, #38786, #26252, #13684, #6903, #32636, #22764, #32428, #31823, #19459, #10581, #32033, #4036, #4225 ),
 ( #16749, #4431, #29331, #34928, #13269, #23153, #25636, #3840, #9981, #35720, #936, #13881, #7496, #16357, #29534, #28726, #28931, #19254, #20059, #16162, #1347, #732, #35526, #26448, #38178, #38975, #22363, #6706, #3637, #538, #25839, #22960, #16553, #29131 ),
 ( #38373, #10174, #35330, #7099, #10384, #19662, #32236, #26047, #7296, #19857, #8289, #10976, #14069, #2153, #36517, #4818, #5021, #36121, #5225, #20450, #27451, #27242, #11378, #23557, #24154, #26843, #39383, #1955, #33651, #11175, #17760, #10774, #23353, #23746 ),
 ( #23943, #36714, #20864, #14881, #33456, #32834, #7701, #20250, #39593, #8497, #7901, #30347, #17553, #33028, #5427, #14473, #14673, #11578, #1743, #14274, #21080, #17966, #33236, #30139, #36317, #35924, #39809, #30552, #8087, #27047, #29725, #2363, #4626, #17153 ),
 ( #20654, #1536, #26648, #39182, #17347, #29925, #37521, #40402, #27850, #8907, #21696, #19009, #15502, #18794, #31166, #5635, #18174, #27649, #30766, #21491, #12206, #22105, #34682, #12616, #12415, #24568, #24778, #8701, #25183, #30966, #9316, #6246, #37714, #31570 ),
 ( #2568, #2772, #40610, #9521, #40205, #15911, #34275, #24360, #37323, #34471, #6457, #3395, #33854, #24986, #11988, #37119, #40007, #36923, #6044, #15090, #15708, #11779, #21281, #34067, #2984, #21893, #31368, #18380, #18578, #5842, #15298, #3192, #9120, #28262 ),
 ( #86, #28060, #35281, #22314, #9934, #29283, #25389, #19615, #4181, #12815, #37928, #25793, #4383, #35082, #22908, #32189, #6857, #22515, #19411, #10126, #1097, #31773, #16508, #38530, #26204, #32387, #16312, #7449, #22714, #20005, #3987, #28680, #19208, #7248 ),
 ( #3788, #28880, #29084, #10529, #689, #35476, #28470, #277, #13227, #7048, #31984, #13632, #34883, #38326, #887, #13420, #25996, #10336, #6657, #19811, #38733, #9735, #16697, #23109, #3589, #16114, #35676, #490, #32586, #13024, #25589, #38133, #39134, #36074 ),
 ( #27193, #4767, #30286, #11128, #26596, #17498, #33403, #8042, #10931, #29678, #14227, #32788, #21028, #23698, #33601, #29487, #20600, #11325, #17707, #7851, #20403, #2102, #24095, #39338, #36266, #32983, #16908, #20806, #14617, #17302, #33184, #35874, #26993, #39751 ),
 ( #29880, #36461, #20204, #23510, #4579, #39540, #4971, #8444, #11528, #1489, #36663, #23307, #1693, #13834, #23890, #10725, #8236, #26800, #30095, #1297, #17106, #26403, #38932, #5176, #7653, #14023, #1904, #14424, #27799, #40350, #5991, #28006, #24935, #12361 ),
 ( #21641, #8651, #24513, #37468, #5376, #40155, #2928, #5578, #21228, #9264, #31113, #11939, #12147, #30711, #40549, #15040, #22051, #21844, #18529, #18118, #18741, #34422, #15447, #2516, #31318, #21436, #34012, #37269, #28203, #5786, #6196, #17915, #30497, #18324 ),
 ( #3140, #15657, #35, #9465, #12562, #27393, #2305, #14828, #34221, #25132, #27601, #37664, #24720, #37064, #39957, #11730, #9065, #24305, #15243, #36870, #8853, #33799, #30914, #2722, #433, #4134, #22461, #7201, #28833, #3535, #35232, #10284, #25742, #28630 ),
 ( #34831, #25340, #13371, #6607, #10080, #29237, #38283, #22859, #38480, #25946, #19154, #16649, #35028, #3942, #3340, #31721, #35431, #16061, #16261, #16463, #7002, #31931, #13179, #12973, #25542, #643, #3738, #19760, #32341, #34629, #19361, #15860, #32145, #6806 ),
 ( #1045, #223, #38083, #31517, #29035, #28417, #13579, #9885, #19568, #38685, #37874, #26153, #10482, #6402, #18953, #12763, #22666, #839, #9681, #22264, #23645, #4914, #1850, #30035, #29437, #23260, #26354, #26545, #36212, #36412, #35827, #39692, #17253, #7401 ),
 ( #20756, #30238, #16855, #7992, #7602, #20154, #23062, #14372, #1250, #32736, #38886, #39083, #20548, #8184, #4531, #35627, #29826, #19954, #7799, #17445, #33347, #2053, #13787, #33132, #17054, #29630, #32536, #4335, #4719, #10679, #39484, #5123, #17656, #1444 ),
 ( #26942, #13976, #10880, #36022, #1639, #23454, #14566, #20352, #32931, #14178, #11273, #26748, #39287, #11075, #23837, #27140, #8397, #2674, #27955, #36613, #20971, #8801, #28160, #18070, #5941, #15193, #30660, #33747, #2469, #33961, #24884, #14776, #40304, #21593 ) ),
 .UNSPECIFIED., .F., .F., .F.,
 ( 6, 5, 2, 5, 6 ),
 ( 4, 1, 1, 1, 1, 1, 1, 1, 1, 1, 1, 1, 1, 1, 1, 1, 1, 1, 1, 1, 1, 1, 1, 1, 1, 1, 1, 1, 1, 1, 1, 4 ),
 ( -0.01000000000000000021, 0.000000000000000000, 0.5000000000000000000, 1.000000000000000000, 1.010000000000000009 ),
 ( 0.000000000000000000, 0.0006830978666945804927, 0.001366195733389160985, 0.001935443955634644784, 0.002390842533431031345, 0.002732391466778321971, 0.003017015577901063870, 0.003244714866799257909, 0.003387026922360628425, 0.003500876566809725445, 0.003586263800146547668, 0.003671651033483370324, 0.003757038266820192981, 0.003842425500157015204, 0.003956275144606112223, 0.004098587200167483173, 0.004269361666841127619, 0.004497060955739321658, 0.004781685066862063557, 0.005123234000209354183, 0.005578632578005740528, 0.006147880800251224326, 0.006830978666945805577, 0.007514076533640385962, 0.008424873689233159518, 0.009563370133724125380, 0.01092956586711328788, 0.01229576160050244865, 0.01411735591168799576, 0.01639434880066993269, 0.01912674026744825076, 0.02185913173422657577 ),
 .UNSPECIFIED. ) ;
#22532=CARTESIAN_POINT ( 'NONE',  ( 30.73821809742792510, -3.303287531218632278, 4.965085915138678807 ) ) ;
#22533=CARTESIAN_POINT ( 'NONE',  ( 23.77293744817952970, 2.857359405969741584, 3.961609048350384743 ) ) ;
#22535=AXIS2_PLACEMENT_3D ( 'NONE', #6868, #28690, #700 ) ;
#22538=CARTESIAN_POINT ( 'NONE',  ( 23.75094394727146252, 3.570271603488096801, 3.156956672783068019 ) ) ;
#22545=CARTESIAN_POINT ( 'NONE',  ( 23.07526676296097179, 0.3585942713019621975, 5.936990365695360872 ) ) ;
#22552=CARTESIAN_POINT ( 'NONE',  ( 25.11613067079463590, -2.903500246237137983, -5.705645831387469613 ) ) ;
#22555=CARTESIAN_POINT ( 'NONE',  ( -73.74378307871597826, -3.485633296868869468, 9.598859659615810003 ) ) ;
#22556=CARTESIAN_POINT ( 'NONE',  ( 27.44318568885298504, 0.9300194081793810019, -4.489570861336245500 ) ) ;
#22559=CARTESIAN_POINT ( 'NONE',  ( 30.76389835349712243, -3.760085712427588600, -4.556058237597376603 ) ) ;
#22560=CARTESIAN_POINT ( 'NONE',  ( 37.17658989031565397, -2.564865607421146887, -5.981013799454680147 ) ) ;
#22562=CARTESIAN_POINT ( 'NONE',  ( 17.10386648299642687, 9.264936115020711682, 2.854956177116559690 ) ) ;
#22563=FACE_OUTER_BOUND ( 'NONE', #21453, .T. ) ;
#22568=CARTESIAN_POINT ( 'NONE',  ( 23.56275793004198249, 1.092801103661935391, -5.226603514420215646 ) ) ;
#22569=CARTESIAN_POINT ( 'NONE',  ( 29.64729738269542381, 1.157578426279490147, -4.258750744271380562 ) ) ;
#22573=EDGE_CURVE ( 'NONE', #5350, #15998, #10816, .T. ) ;
#22575=CARTESIAN_POINT ( 'NONE',  ( 21.76158391687864579, 5.855790371669074901, -3.369038255546072946 ) ) ;
#22576=CARTESIAN_POINT ( 'NONE',  ( 84.31734228151684363, 3.084090681639994003, 0.3216814846013044127 ) ) ;
#22578=EDGE_LOOP ( 'NONE', ( #7829, #40031, #29484, #19699 ) ) ;
#22579=CARTESIAN_POINT ( 'NONE',  ( 27.41857586891900667, 1.095318458406062456, 4.485729903744793745 ) ) ;
#22595=CARTESIAN_POINT ( 'NONE',  ( 33.78796187971178000, -4.855747518448159994, -3.446936011855299853 ) ) ;
#22596=CARTESIAN_POINT ( 'NONE',  ( 22.62429625317078674, 4.579493676427568438, -3.091892255925898336 ) ) ;
#22597=VERTEX_POINT ( 'NONE', #31438 ) ;
#22603=CARTESIAN_POINT ( 'NONE',  ( -72.89750464017865283, 3.404720670759703527, -9.864174393176885047 ) ) ;
#22607=CARTESIAN_POINT ( 'NONE',  ( 85.86655237490620607, 0.5075193453549979861, -5.999391133436077439 ) ) ;
#22610=CARTESIAN_POINT ( 'NONE',  ( 22.06611006309120171, 4.208718600211970973, -2.305420481420197731 ) ) ;
#22611=CARTESIAN_POINT ( 'NONE',  ( 33.61618589921860689, -1.223535437620471011, 5.453016838738055760 ) ) ;
#22619=CARTESIAN_POINT ( 'NONE',  ( 34.13625311161768394, -3.134515127487323749, 5.534185905105376335 ) ) ;
#22622=CARTESIAN_POINT ( 'NONE',  ( 88.25065740119208613, -0.7696024251930051463, 2.713887439742028285 ) ) ;
#22627=CARTESIAN_POINT ( 'NONE',  ( -69.47662317642280527, -46.72710078822078827, 9.894078484842815158 ) ) ;
#22632=LINE ( 'NONE', #22232, #10358 ) ;
#22638=CARTESIAN_POINT ( 'NONE',  ( 21.81293742820567871, 1.745484945909191676, 6.400703180478840792 ) ) ;
#22650=CARTESIAN_POINT ( 'NONE',  ( 23.90047232000282662, 3.021372428902185714, -3.777954186841565587 ) ) ;
#22653=CARTESIAN_POINT ( 'NONE',  ( 21.85643539959774273, -7.955861821551272861, 12.12136874776577322 ) ) ;
#22654=CARTESIAN_POINT ( 'NONE',  ( 21.86870537174298335, 3.698784010477664808, -3.388912068454548621 ) ) ;
#22657=CARTESIAN_POINT ( 'NONE',  ( 88.87549651282381546, -1.666836616135117799, 1.222388837546040330 ) ) ;
#22661=CARTESIAN_POINT ( 'NONE',  ( 15.05324942562365464, -4.021369621152198981, 2.555821655718428342 ) ) ;
#22664=CARTESIAN_POINT ( 'NONE',  ( 36.94849503072852315, -2.665731531992193926, 5.973104270911074209 ) ) ;
#22666=CARTESIAN_POINT ( 'NONE',  ( 36.79757171488110146, -2.556340929038857901, -5.949549037378906391 ) ) ;
#22668=CARTESIAN_POINT ( 'NONE',  ( 84.10560360838722715, 3.011181495113149698, -0.2494236887672163505 ) ) ;
#22674=CARTESIAN_POINT ( 'NONE',  ( 31.98929602146294116, -3.342055116537107295, 5.177998144997084218 ) ) ;
#22678=CARTESIAN_POINT ( 'NONE',  ( 23.38377539308148201, 3.557990533569439506, 3.100742785337903928 ) ) ;
#22681=CARTESIAN_POINT ( 'NONE',  ( 87.09538489576669917, -1.473322093048123005, -4.746830818090543858 ) ) ;
#22694=VECTOR ( 'NONE', #39815, 1000.000000000000000 ) ;
#22697=CARTESIAN_POINT ( 'NONE',  ( 16.37661538275509443, 9.897519661642579791, -2.762364919055407597 ) ) ;
#22701=CARTESIAN_POINT ( 'NONE',  ( -12.99139449055068241, -10.90558813203967148, 6.000000000000000000 ) ) ;
#22704=CARTESIAN_POINT ( 'NONE',  ( 87.00441857019603731, 0.6302321798448609069, -4.918210918608230564 ) ) ;
#22705=CARTESIAN_POINT ( 'NONE',  ( 28.10206848396558499, 1.736549293047330300, -3.980455106513370200 ) ) ;
#22713=CARTESIAN_POINT ( 'NONE',  ( 0.000000000000000000, 10.37661300689600097, 2.500000000000000000 ) ) ;
#22714=CARTESIAN_POINT ( 'NONE',  ( 29.34601568743050493, 0.9961685670913987822, -4.626954042955691015 ) ) ;
#22715=LINE ( 'NONE', #31985, #23319 ) ;
#22718=CARTESIAN_POINT ( 'NONE',  ( -81.20922607448022745, 10.50636700977107196, 3.841544977761441437 ) ) ;
#22720=CARTESIAN_POINT ( 'NONE',  ( 21.94901396481228417, -12.22285702164925958, -2.500000000000000000 ) ) ;
#22732=CARTESIAN_POINT ( 'NONE',  ( 23.45399895271802748, 3.179065097157539821, 3.819164652932915072 ) ) ;
#22738=CARTESIAN_POINT ( 'NONE',  ( 23.43551384144531369, 3.792528780310672865, 3.105475544838504298 ) ) ;
#22744=CARTESIAN_POINT ( 'NONE',  ( 24.12522002703219570, 0.5066050462473785654, 5.093085906072658986 ) ) ;
#22754=CARTESIAN_POINT ( 'NONE',  ( 22.82155563815204502, -7.011124981618892527, 0.5620805258418327677 ) ) ;
#22757=CARTESIAN_POINT ( 'NONE',  ( -79.24449270190245898, -6.613341267620478803, 5.568385975749495564 ) ) ;
#22764=CARTESIAN_POINT ( 'NONE',  ( 32.06915089713219658, 0.2527768776864406375, -4.727205254402804258 ) ) ;
#22771=DIRECTION ( 'NONE',  ( 1.000000000000000000, 0.000000000000000000, 0.000000000000000000 ) ) ;
#22772=CARTESIAN_POINT ( 'NONE',  ( 25.04937939002015668, 1.718265418675629652, -4.340997593773719743 ) ) ;
#22773=CARTESIAN_POINT ( 'NONE',  ( 35.50970222813752031, -1.197800581197451031, -5.486251443588301413 ) ) ;
#22778=CARTESIAN_POINT ( 'NONE',  ( 86.17157777234386629, 0.6269314577163517255, 5.990399513018050293 ) ) ;
#22783=VECTOR ( 'NONE', #24976, 1000.000000000000000 ) ;
#22791=VERTEX_POINT ( 'NONE', #2271 ) ;
#22792=CARTESIAN_POINT ( 'NONE',  ( 25.62749773886924842, 1.970388730450938430, 4.206188844162269014 ) ) ;
#22795=CARTESIAN_POINT ( 'NONE',  ( 21.85643539959776760, -14.20048109512665135, 6.697783101734796851 ) ) ;
#22796=CARTESIAN_POINT ( 'NONE',  ( 22.38767867107881671, 4.911711129367581918, -3.073573574929423735 ) ) ;
#22799=EDGE_CURVE ( 'NONE', #15995, #12484, #14794, .T. ) ;
#22800=ORIENTED_EDGE ( 'NONE', *, *, #22230, .F. ) ;
#22805=CARTESIAN_POINT ( 'NONE',  ( -71.81742943715566696, 1.311122306527585213, -9.960446608825028747 ) ) ;
#22809=CARTESIAN_POINT ( 'NONE',  ( 84.13636243568421946, 2.973867306686137191, 1.134085816324387430 ) ) ;
#22813=CIRCLE ( 'NONE', #8308, 12.80480339192541628 ) ;
#22820=CARTESIAN_POINT ( 'NONE',  ( 30.51641733573469040, -0.1366954951678319985, 4.969222986220390048 ) ) ;
#22822=CARTESIAN_POINT ( 'NONE',  ( 87.25792211136258913, 0.3454849704027515567, -4.698443967043519187 ) ) ;
#22829=CARTESIAN_POINT ( 'NONE',  ( -71.98686916902434518, 0.1712994517134147909, 9.947269908901157365 ) ) ;
#22836=CARTESIAN_POINT ( 'NONE',  ( 21.79934511777053174, 1.490787985410582994, 6.749058457536040834 ) ) ;
#22845=CARTESIAN_POINT ( 'NONE',  ( 24.11137768457082942, 2.995069816642412786, -3.734747807212182913 ) ) ;
#22848=ORIENTED_EDGE ( 'NONE', *, *, #29344, .F. ) ;
#22849=CARTESIAN_POINT ( 'NONE',  ( 21.85643539959777470, -4.742028430345498258, -11.91557605213902882 ) ) ;
#22850=CARTESIAN_POINT ( 'NONE',  ( 21.66074814249151714, 7.048403176780774437, 2.215087588513221758E-12 ) ) ;
#22854=CARTESIAN_POINT ( 'NONE',  ( 88.65680102019307185, -1.418189719613276223, -2.767552868364703045 ) ) ;
#22856=CARTESIAN_POINT ( 'NONE',  ( 14.68773611674814283, 12.90757323260954514, 2.500000034667914761 ) ) ;
#22857=CARTESIAN_POINT ( 'NONE',  ( 31.37338404834114769, -3.012165633454263247, 5.102973367540887928 ) ) ;
#22859=CARTESIAN_POINT ( 'NONE',  ( 36.42081795466733496, -3.114981983614129035, -5.890747501273418507 ) ) ;
#22861=CARTESIAN_POINT ( 'NONE',  ( 84.92084393738451809, 1.980781149894611959, 4.774541556935223419 ) ) ;
#22863=CARTESIAN_POINT ( 'NONE',  ( -74.68562510149382661, -2.717749937412478722, 10.59137344923616375 ) ) ;
#22868=CARTESIAN_POINT ( 'NONE',  ( 32.90341992358483481, -3.215921544857364811, 5.341772469908477206 ) ) ;
#22871=CARTESIAN_POINT ( 'NONE',  ( 37.10938198393888854, -2.404265875854591172, 5.951784697920204259 ) ) ;
#22874=DIRECTION ( 'NONE',  ( 0.000000000000000000, 0.000000000000000000, -1.000000000000000000 ) ) ;
#22877=DIRECTION ( 'NONE',  ( 0.000000000000000000, 0.000000000000000000, -1.000000000000000000 ) ) ;
#22881=CYLINDRICAL_SURFACE ( 'NONE', #35278, 15.73502530973474478 ) ;
#22888=ORIENTED_EDGE ( 'NONE', *, *, #11586, .F. ) ;
#22891=CYLINDRICAL_SURFACE ( 'NONE', #15039, 27.95745752244933868 ) ;
#22895=B_SPLINE_CURVE_WITH_KNOTS ( 'NONE', 3,
 ( #34601, #24485, #18092, #30685, #34195, #27772, #37041, #18927 ),
 .UNSPECIFIED., .F., .F.,
 ( 4, 2, 2, 4 ),
 ( -2.215204784179636180E-05, 0.0001932311667254880505, 0.0004086143812927724899, 0.0008393808104273412602 ),
 .UNSPECIFIED. ) ;
#22902=CARTESIAN_POINT ( 'NONE',  ( 27.13744335700502219, 0.8961374054434056990, -5.485310518450965844 ) ) ;
#22908=CARTESIAN_POINT ( 'NONE',  ( 37.10285757261533490, -2.625508518994315477, -5.990196095338164106 ) ) ;
#22913=CARTESIAN_POINT ( 'NONE',  ( 21.90967695140060201, -12.75691164195780303, -2.500000000000000444 ) ) ;
#22916=CARTESIAN_POINT ( 'NONE',  ( 30.84950422756433142, -2.934832344082245026, 5.021209251427320552 ) ) ;
#22918=CARTESIAN_POINT ( 'NONE',  ( 30.74493630087459906, 0.4681640684078945958, 4.860621472976927038 ) ) ;
#22925=CARTESIAN_POINT ( 'NONE',  ( -18.48280404870591553, -63.98126818465317456, -2.500000000000000000 ) ) ;
#22926=CARTESIAN_POINT ( 'NONE',  ( 23.04163317972315994, 3.256728484989337868, 3.973781910508482174 ) ) ;
#22931=EDGE_CURVE ( 'NONE', #8713, #34290, #7123, .T. ) ;
#22934=VERTEX_POINT ( 'NONE', #26070 ) ;
#22936=CARTESIAN_POINT ( 'NONE',  ( 22.18636049064522453, 5.270353752318829521, 3.074731245731978646 ) ) ;
#22938=CARTESIAN_POINT ( 'NONE',  ( 15.01546246723575173, -4.177556355646068198, 2.539460141531804105 ) ) ;
#22944=CARTESIAN_POINT ( 'NONE',  ( 25.38719211221763317, 0.7154116930338988434, 4.601124151639230497 ) ) ;
#22945=CARTESIAN_POINT ( 'NONE',  ( 14.61824258762769091, -4.523863395544843513, -2.500000000000095035 ) ) ;
#22953=CARTESIAN_POINT ( 'NONE',  ( 24.43246502961036626, -0.4583524411608039251, -6.968550363799582925 ) ) ;
#22956=CARTESIAN_POINT ( 'NONE',  ( -74.63738614184299536, -2.659024657488486376, 9.335863256658281983 ) ) ;
#22960=CARTESIAN_POINT ( 'NONE',  ( 23.38513527390059821, 3.559322506240827799, -3.095448560026594631 ) ) ;
#22962=DIRECTION ( 'NONE',  ( 1.000000000000000000, 0.000000000000000000, 0.000000000000000000 ) ) ;
#22964=CARTESIAN_POINT ( 'NONE',  ( 8.290806648384990041, -10.90558813203967148, 6.000000000000000000 ) ) ;
#22968=CARTESIAN_POINT ( 'NONE',  ( 22.19836525915095393, 0.7666314114482586373, -6.808643381459575039 ) ) ;
#22969=CARTESIAN_POINT ( 'NONE',  ( 35.52266373076683692, -1.204347071998821628, -5.489450149774045329 ) ) ;
#22976=CARTESIAN_POINT ( 'NONE',  ( 87.32347380307142259, -1.421525632644524251, -4.720772940814831564 ) ) ;
#22977=EDGE_CURVE ( 'NONE', #4684, #30447, #30598, .T. ) ;
#22978=VERTEX_POINT ( 'NONE', #36338 ) ;
#22979=CARTESIAN_POINT ( 'NONE',  ( -74.18786092369259677, 6.905699905533330352, -10.73326951011580555 ) ) ;
#22986=LINE ( 'NONE', #16774, #445 ) ;
#22987=VERTEX_POINT ( 'NONE', #23372 ) ;
#22989=CARTESIAN_POINT ( 'NONE',  ( 33.79294173806484736, -4.878189388823929384, 3.391004255377942922 ) ) ;
#22997=CARTESIAN_POINT ( 'NONE',  ( 33.78816593493456111, -4.856674916897421035, -3.444637928637498181 ) ) ;
#23003=CARTESIAN_POINT ( 'NONE',  ( -72.05444927908816055, 4.856418035946385103, -9.936797814648945959 ) ) ;
#23007=CARTESIAN_POINT ( 'NONE',  ( 86.38495421312710221, -0.4360953479145894263, -5.826368990767747391 ) ) ;
#23008=CARTESIAN_POINT ( 'NONE',  ( 24.75848867132678421, 3.019268511056711901, -3.350244135560401126 ) ) ;
#23015=DIRECTION ( 'NONE',  ( -1.000000000000000000, 0.000000000000000000, 0.000000000000000000 ) ) ;
#23017=CARTESIAN_POINT ( 'NONE',  ( 32.78029040100151548, -0.9298081016050898651, 5.322555130032219139 ) ) ;
#23020=CARTESIAN_POINT ( 'NONE',  ( 84.98726364908050357, 2.895996327189970021, 0.3032432708941606436 ) ) ;
#23025=CARTESIAN_POINT ( 'NONE',  ( 1.700390093233090871, -29.56993018339339940, -6.000000000000001776 ) ) ;
#23031=CARTESIAN_POINT ( 'NONE',  ( -80.13811754935157694, -6.651623698664113071, 3.918677847151820881 ) ) ;
#23033=ORIENTED_EDGE ( 'NONE', *, *, #30978, .F. ) ;
#23036=CARTESIAN_POINT ( 'NONE',  ( 25.23678314328794059, 2.025140460799608189, 4.185677819315343662 ) ) ;
#23039=CIRCLE ( 'NONE', #21093, 3.000000000000002665 ) ;
#23044=B_SPLINE_SURFACE_WITH_KNOTS ( 'NONE', 5, 3, ( 
 ( #3527, #27995, #12965, #40539, #30904, #24922, #2712 ),
 ( #9253, #21832, #31308, #31919, #38469, #13569, #4519 ),
 ( #19752, #35617, #3729, #35814, #17039, #32329, #39069 ),
 ( #10272, #4126, #29223, #16639, #23053, #1037, #7590 ),
 ( #26344, #26141, #38673, #25730, #26534, #1433, #10472 ),
 ( #23248, #32135, #38875, #22850, #13966, #6992, #13775 ),
 ( #20144, #7389, #3934, #19944, #25935, #32523, #629 ),
 ( #29617, #22451, #16452, #32724, #38274, #35020, #13171 ),
 ( #10069, #29025, #828, #4323, #6795, #16844, #29426 ),
 ( #19349, #1240, #16253, #10667, #28824, #22654, #35222 ),
 ( #35423, #13360, #19559, #7191, #20338, #11464, #14360 ),
 ( #29815, #33121, #39274, #20535, #30023, #11261, #17850 ),
 ( #10901, #20995, #26968, #26568, #4550, #14593, #14397 ) ),
 .UNSPECIFIED., .F., .F., .F.,
 ( 6, 2, 5, 6 ),
 ( 4, 1, 1, 1, 4 ),
 ( 0.000000000000000000, 0.5000000000000000000, 1.000000000000000000, 1.064435095764829642 ),
 ( -0.001274899269766986438, 0.0006125503651162966887, 0.002499999999999579815, 0.004387449634882863159, 0.006274899269766145635 ),
 .UNSPECIFIED. ) ;
#23046=CARTESIAN_POINT ( 'NONE',  ( 24.14380846906243150, 3.078890981682416150, -3.628619729749268608 ) ) ;
#23051=CARTESIAN_POINT ( 'NONE',  ( 21.85643539959776049, -3.417000210761661272, 14.19984240075801374 ) ) ;
#23053=CARTESIAN_POINT ( 'NONE',  ( 20.05068032856350513, 11.88301801996953344, -1.993596777108510576 ) ) ;
#23056=CARTESIAN_POINT ( 'NONE',  ( 88.90249899953845159, -1.697492344831515121, -0.8687328377452782080 ) ) ;
#23060=CARTESIAN_POINT ( 'NONE',  ( 31.84879310987939149, -3.762318538055401618, 4.773639746032809938 ) ) ;
#23061=CARTESIAN_POINT ( 'NONE',  ( 33.11561061937418060, -3.385635371879725408, -5.363104269438873750 ) ) ;
#23062=CARTESIAN_POINT ( 'NONE',  ( 36.14138348061285200, -3.141491348386876936, -5.847134993448860563 ) ) ;
#23064=CARTESIAN_POINT ( 'NONE',  ( 84.47471770354184173, 2.556968559651632944, -3.354246977694447462 ) ) ;
#23069=CARTESIAN_POINT ( 'NONE',  ( 29.48897355024926270, -3.189277998897150912, 4.808865534657858376 ) ) ;
#23073=CARTESIAN_POINT ( 'NONE',  ( 36.44519052358557332, -1.732482462384099975, 5.730822330882753057 ) ) ;
#23074=DIRECTION ( 'NONE',  ( -0.000000000000000000, -0.000000000000000000, -1.000000000000000000 ) ) ;
#23075=CARTESIAN_POINT ( 'NONE',  ( 33.45304404609620263, -3.772033185430891500, 5.158132413726952414 ) ) ;
#23076=CARTESIAN_POINT ( 'NONE',  ( 86.82478445301771330, -1.108591820897244062, 5.258890510423615439 ) ) ;
#23078=ORIENTED_EDGE ( 'NONE', *, *, #40496, .T. ) ;
#23086=CARTESIAN_POINT ( 'NONE',  ( 21.91074531573966766, 5.459064786471969022, 3.355207856022180302 ) ) ;
#23093=CYLINDRICAL_SURFACE ( 'NONE', #17170, 6.000000000000002665 ) ;
#23098=CARTESIAN_POINT ( 'NONE',  ( 24.20108879139602465, 2.667881056255625438, -3.983563230078315698 ) ) ;
#23102=CARTESIAN_POINT ( 'NONE',  ( 29.46612689758034875, 1.430465584783186639, -3.840811867917949929 ) ) ;
#23104=CARTESIAN_POINT ( 'NONE',  ( -70.05493584469058987, -21.28726706566848748, 9.961909801952206323 ) ) ;
#23109=CARTESIAN_POINT ( 'NONE',  ( 34.45378869156874657, -1.156911132109146312, -5.566333934908320735 ) ) ;
#23117=CARTESIAN_POINT ( 'NONE',  ( 27.58409624374816360, 1.448159382144707186, 4.473608046789665060 ) ) ;
#23123=CARTESIAN_POINT ( 'NONE',  ( -70.92837670882107659, 3.729367930467589076, 0.000000000000000000 ) ) ;
#23125=CARTESIAN_POINT ( 'NONE',  ( 85.38650254764779390, 1.316965040104128626, -5.564122293564899735 ) ) ;
#23130=CARTESIAN_POINT ( 'NONE',  ( 23.43505160883933058, 3.791633034196467467, 3.107909060890779340 ) ) ;
#23131=CYLINDRICAL_SURFACE ( 'NONE', #26100, 1.500000000000001332 ) ;
#23137=CARTESIAN_POINT ( 'NONE',  ( 22.61475275727087464, 0.2954930242483900238, 6.495504608876625952 ) ) ;
#23145=CARTESIAN_POINT ( 'NONE',  ( 24.25791012409692371, 0.7154099962172090210, -6.776768987914707942 ) ) ;
#23149=CARTESIAN_POINT ( 'NONE',  ( -77.42388607530644151, -4.859301208013656392, 9.188011873594817303 ) ) ;
#23150=CYLINDRICAL_SURFACE ( 'NONE', #35793, 9.386006772603931125 ) ;
#23153=CARTESIAN_POINT ( 'NONE',  ( 35.83227016345950489, -3.728989527342261301, -5.623816504269203875 ) ) ;
#23154=DIRECTION ( 'NONE',  ( -0.000000000000000000, -0.000000000000000000, -1.000000000000000000 ) ) ;
#23168=CARTESIAN_POINT ( 'NONE',  ( 21.78047233922835346, 5.616103166486084319, -3.473245622192032034 ) ) ;
#23169=CARTESIAN_POINT ( 'NONE',  ( 84.44530234979703209, 2.765803402995568927, 2.732740112990733383 ) ) ;
#23170=ADVANCED_FACE ( 'NONE', ( #33050 ), #9151, .F. ) ;
#23179=CARTESIAN_POINT ( 'NONE',  ( 33.68904022949467958, -4.468562645166327840, 4.246708699803020792 ) ) ;
#23182=ORIENTED_EDGE ( 'NONE', *, *, #4826, .T. ) ;
#23188=CARTESIAN_POINT ( 'NONE',  ( 33.75963076984755418, -4.729058622324783023, -3.755006780454513304 ) ) ;
#23192=CARTESIAN_POINT ( 'NONE',  ( 14.71633116765073623, -5.064965072526596224, -2.500000000000000888 ) ) ;
#23194=CARTESIAN_POINT ( 'NONE',  ( -75.36736324129955733, -5.074094651746722917, -8.962379545620084542 ) ) ;
#23198=CARTESIAN_POINT ( 'NONE',  ( -4.220127061295482087E-17, 0.7293679304675931840, 6.000000000000000000 ) ) ;
#23202=CARTESIAN_POINT ( 'NONE',  ( 33.70353959993166626, -1.254899476156281946, 5.466650496391561198 ) ) ;
#23203=EDGE_CURVE ( 'NONE', #1317, #218, #40647, .T. ) ;
#23209=DIRECTION ( 'NONE',  ( -0.000000000000000000, -1.000000000000000000, -0.000000000000000000 ) ) ;
#23213=CARTESIAN_POINT ( 'NONE',  ( 36.99281227302647324, -2.718855070858015033, 5.980021048388253213 ) ) ;
#23216=CARTESIAN_POINT ( 'NONE',  ( 86.87490948991990081, 0.7757029256828257280, 5.355124474773749199 ) ) ;
#23223=CARTESIAN_POINT ( 'NONE',  ( -79.13014441944265798, 11.46068214799393736, -5.736672290455380185 ) ) ;
#23232=CARTESIAN_POINT ( 'NONE',  ( 25.12776268638631549, 1.000125724568426078, 4.612937808490496394 ) ) ;
#23233=VERTEX_POINT ( 'NONE', #37300 ) ;
#23236=CARTESIAN_POINT ( 'NONE',  ( 37.83867290611771494, -6.084034091406928191, -6.000000000000000000 ) ) ;
#23241=CARTESIAN_POINT ( 'NONE',  ( 23.65147222854444919, 3.378127406782373665, -3.542646716268693208 ) ) ;
#23246=CARTESIAN_POINT ( 'NONE',  ( 22.79131883835711037, -5.922936844141047708, 5.170149038749508819 ) ) ;
#23248=CARTESIAN_POINT ( 'NONE',  ( 21.80570325383046182, 6.356989464231188158, 3.898355529982616918 ) ) ;
#23249=CARTESIAN_POINT ( 'NONE',  ( 13.80252870930811326, 11.14042161257683006, 2.500000000000004885 ) ) ;
#23252=CARTESIAN_POINT ( 'NONE',  ( 87.57592060778061693, -0.6244806207018304134, 5.359096402341661403 ) ) ;
#23256=CARTESIAN_POINT ( 'NONE',  ( -77.80754174939649204, -5.030728402074980288, 8.890429129847960965 ) ) ;
#23258=CARTESIAN_POINT ( 'NONE',  ( 32.23520098731326300, -3.776787765129337782, 4.847381814357383689 ) ) ;
#23259=CARTESIAN_POINT ( 'NONE',  ( 28.89658576139254720, -2.947360769642642708, -4.716409093270361730 ) ) ;
#23260=CARTESIAN_POINT ( 'NONE',  ( 32.77973188623823120, -0.9315922670084764157, -5.322467960295677258 ) ) ;
#23270=ORIENTED_EDGE ( 'NONE', *, *, #13429, .T. ) ;
#23271=CARTESIAN_POINT ( 'NONE',  ( 35.36826174472263062, -3.792953908414599340, 5.510393643995938895 ) ) ;
#23275=ORIENTED_EDGE ( 'NONE', *, *, #18970, .F. ) ;
#23280=CARTESIAN_POINT ( 'NONE',  ( 21.75869166788903186, 5.877497079131895674, 3.362859741260915580 ) ) ;
#23288=CARTESIAN_POINT ( 'NONE',  ( 23.68961767579556010, 2.539811605600059252, -4.211040149488679774 ) ) ;
#23292=CARTESIAN_POINT ( 'NONE',  ( 27.39974682155295582, 1.067777558387527748, -4.482791175521097848 ) ) ;
#23297=CARTESIAN_POINT ( 'NONE',  ( 29.21535032918476915, 2.216127810226045547, -1.021449648108430086 ) ) ;
#23299=CYLINDRICAL_SURFACE ( 'NONE', #20247, 8.080217238368755162 ) ;
#23307=CARTESIAN_POINT ( 'NONE',  ( 36.99142113593869396, -2.973170736671415071, -5.979803927800903196 ) ) ;
#23314=CARTESIAN_POINT ( 'NONE',  ( 36.88183944235395728, -2.428786062484896480, 5.959470125505070826 ) ) ;
#23319=VECTOR ( 'NONE', #19812, 1000.000000000000000 ) ;
#23322=CARTESIAN_POINT ( 'NONE',  ( 86.03314645334975808, 0.1914443106846198395, -5.998834454465889365 ) ) ;
#23323=CARTESIAN_POINT ( 'NONE',  ( 85.03548763332921112, 1.825262285978656251, -4.977705953854337118 ) ) ;
#23328=CARTESIAN_POINT ( 'NONE',  ( 21.83311778635127709, 5.946302252710771619, 3.143334175583627932 ) ) ;
#23334=CARTESIAN_POINT ( 'NONE',  ( 21.78513789440741277, 0.2163316297486854445, 8.389159167568045916 ) ) ;
#23339=CARTESIAN_POINT ( 'NONE',  ( -17.69482985384421880, -42.37473357531882101, -6.000000000000000000 ) ) ;
#23342=CARTESIAN_POINT ( 'NONE',  ( 29.08816165369256268, -2.077165169587669613, 5.788842218736271583 ) ) ;
#23345=CARTESIAN_POINT ( 'NONE',  ( -73.52991696981251835, -0.8431142006776708442, 10.87125227208380984 ) ) ;
#23346=CARTESIAN_POINT ( 'NONE',  ( 21.73433939381562752, 0.2312908497712835021, -9.065555101204189725 ) ) ;
#23348=CIRCLE ( 'NONE', #1669, 6.000000000000002665 ) ;
#23353=CARTESIAN_POINT ( 'NONE',  ( 21.73836974088880325, 4.234938348740031167, -2.803927442718175289 ) ) ;
#23362=CARTESIAN_POINT ( 'NONE',  ( 21.58862418887968460, 7.202556094215188054, 2.923978954502209682 ) ) ;
#23363=ORIENTED_EDGE ( 'NONE', *, *, #40112, .F. ) ;
#23366=CARTESIAN_POINT ( 'NONE',  ( 85.38915795161820199, 1.318023545160245558, -5.584599991349963766 ) ) ;
#23372=CARTESIAN_POINT ( 'NONE',  ( 23.06594672544511582, -8.086844732617873177, 2.500000000000001332 ) ) ;
#23378=CARTESIAN_POINT ( 'NONE',  ( 33.71578150949435582, -4.562017431774315845, 4.082147076938466235 ) ) ;
#23387=CARTESIAN_POINT ( 'NONE',  ( 21.85643539959774273, 11.87292600555486466, 1.968928953175947072 ) ) ;
#23392=CARTESIAN_POINT ( 'NONE',  ( 14.74088296503634155, -4.694786528388449121, 2.506211950836694680 ) ) ;
#23393=CARTESIAN_POINT ( 'NONE',  ( -74.90697995311768409, -4.711520037844358022, -9.180746725924359808 ) ) ;
#23396=FACE_OUTER_BOUND ( 'NONE', #32028, .T. ) ;
#23401=CARTESIAN_POINT ( 'NONE',  ( -70.92837670882107659, -37.87473357531881391, -10.00000000000000888 ) ) ;
#23409=CARTESIAN_POINT ( 'NONE',  ( 30.51572969112700306, -0.1387093445857095764, 4.969115662648612819 ) ) ;
#23411=ADVANCED_FACE ( 'NONE', ( #23867 ), #36849, .F. ) ;
#23414=CARTESIAN_POINT ( 'NONE',  ( 85.76961320806377387, 1.955528254085527662, 4.811735575706960866 ) ) ;
#23417=DIRECTION ( 'NONE',  ( 1.000000000000000000, 8.959828616340678715E-16, 0.000000000000000000 ) ) ;
#23421=CARTESIAN_POINT ( 'NONE',  ( 23.71049985568843965, -7.011247657926062971, -2.558818689067067886 ) ) ;
#23422=ORIENTED_EDGE ( 'NONE', *, *, #4826, .F. ) ;
#23425=EDGE_CURVE ( 'NONE', #38217, #10579, #20577, .T. ) ;
#23426=LINE ( 'NONE', #29799, #2360 ) ;
#23429=CARTESIAN_POINT ( 'NONE',  ( 22.48842088587040777, 0.6138701667877143331, 6.557769318399328640 ) ) ;
#23439=CARTESIAN_POINT ( 'NONE',  ( 23.68965556879579992, 3.465983028975976321, -3.401521908042043130 ) ) ;
#23443=CARTESIAN_POINT ( 'NONE',  ( 22.81791704898701667, -6.824503531841428661, 2.299112860430994054 ) ) ;
#23448=CARTESIAN_POINT ( 'NONE',  ( 88.51539661956502414, -1.738042312505858389, 3.005881034771096250 ) ) ;
#23452=CARTESIAN_POINT ( 'NONE',  ( 24.15140053283135657, 3.654133365256820198, -2.050164366749841260 ) ) ;
#23453=CARTESIAN_POINT ( 'NONE',  ( 16.00230772547182667, -3.352604421649032940, -2.703945156471453171 ) ) ;
#23454=CARTESIAN_POINT ( 'NONE',  ( 35.78589809970488034, -3.160013725310466981, -5.791652902311821727 ) ) ;
#23456=CARTESIAN_POINT ( 'NONE',  ( 84.10558833958633329, 3.011200051076408091, -0.2484360993799872019 ) ) ;
#23464=VERTEX_POINT ( 'NONE', #17477 ) ;
#23465=CARTESIAN_POINT ( 'NONE',  ( 27.81686590159541694, 1.845386698342884602, 3.904314145750329867 ) ) ;
#23479=ORIENTED_EDGE ( 'NONE', *, *, #39734, .F. ) ;
#23480=CARTESIAN_POINT ( 'NONE',  ( 24.40726884955499543, 2.958944204706972503, 3.690054115108988952 ) ) ;
#23485=ORIENTED_EDGE ( 'NONE', *, *, #18053, .T. ) ;
#23487=CARTESIAN_POINT ( 'NONE',  ( -4.890026461918812295, -8.951974136083761024, 6.000000000000000000 ) ) ;
#23488=CARTESIAN_POINT ( 'NONE',  ( 21.38476492232890180, 5.476885306300394163, -3.544007777260224312 ) ) ;
#23491=CARTESIAN_POINT ( 'NONE',  ( 24.25544397694150689, 2.781918247062924898, -3.883429013402408536 ) ) ;
#23492=CARTESIAN_POINT ( 'NONE',  ( -62.92837670882106238, -42.37473357531882812, 6.000000000000000000 ) ) ;
#23495=LINE ( 'NONE', #4371, #5234 ) ;
#23497=CARTESIAN_POINT ( 'NONE',  ( -70.82888935184436718, -48.61702805680357642, 6.000000000000001776 ) ) ;
#23499=CARTESIAN_POINT ( 'NONE',  ( 85.68874278272487288, 2.108061670072472360, -3.902156445801064244 ) ) ;
#23500=CARTESIAN_POINT ( 'NONE',  ( 29.60215801812428182, 1.109421360397880862, -4.380391640306282142 ) ) ;
#23506=CARTESIAN_POINT ( 'NONE',  ( -74.03009556761388410, -1.796639617249599086, -10.77097688889393190 ) ) ;
#23510=CARTESIAN_POINT ( 'NONE',  ( 34.77080612335073795, -3.235625644562878822, -5.633223249305419067 ) ) ;
#23517=CARTESIAN_POINT ( 'NONE',  ( 25.58352385666275097, 2.439062859384895532, 4.005113320270204724 ) ) ;
#23521=CIRCLE ( 'NONE', #30799, 0.9999999999999991118 ) ;
#23527=CARTESIAN_POINT ( 'NONE',  ( -70.17638756726756810, -48.41860179101485073, 9.972019997609882225 ) ) ;
#23532=CARTESIAN_POINT ( 'NONE',  ( 23.43077426150285092, 3.780410721560847342, 3.135869166350258919 ) ) ;
#23540=CARTESIAN_POINT ( 'NONE',  ( 22.60888406660597028, 0.2903629327645729230, 6.504315945443690516 ) ) ;
#23541=CARTESIAN_POINT ( 'NONE',  ( 14.76643007562886112, -4.521128121716065706, -2.511026874211885751 ) ) ;
#23544=VERTEX_POINT ( 'NONE', #3322 ) ;
#23548=CARTESIAN_POINT ( 'NONE',  ( 27.76889013493211067, -0.3210463222110187531, 6.029547961152755597 ) ) ;
#23552=CARTESIAN_POINT ( 'NONE',  ( 21.73423954385304668, 0.2273991419590928875, -9.075701020149493203 ) ) ;
#23557=CARTESIAN_POINT ( 'NONE',  ( 34.63600047421554962, -0.7840873862764304869, -5.277546382571144612 ) ) ;
#23558=PLANE ( 'NONE',  #16088 ) ;
#23569=CARTESIAN_POINT ( 'NONE',  ( 87.73180046618776373, -1.932853647757891258, -3.545598201197500465 ) ) ;
#23572=AXIS2_PLACEMENT_3D ( 'NONE', #1525, #13872, #14059 ) ;
#23579=EDGE_CURVE ( 'NONE', #15644, #37970, #37448, .T. ) ;
#23582=CARTESIAN_POINT ( 'NONE',  ( 33.75147498838597215, -4.699296933879914206, 3.805678930683413785 ) ) ;
#23584=CARTESIAN_POINT ( 'NONE',  ( 25.01091293555841233, 3.329590545877085805, 1.936828124349011526 ) ) ;
#23589=CARTESIAN_POINT ( 'NONE',  ( 17.35285164467449093, 14.28221863251290991, 2.500000000000000000 ) ) ;
#23590=CARTESIAN_POINT ( 'NONE',  ( 21.85643539959775339, 6.533355437427212919, 10.99619876466361212 ) ) ;
#23593=CARTESIAN_POINT ( 'NONE',  ( 14.76814867959672739, -5.160745194441147099, 2.500000607217906623 ) ) ;
#23594=CARTESIAN_POINT ( 'NONE',  ( -76.81575550944289432, 9.394122235356590522, -9.604269881316103152 ) ) ;
#23609=CARTESIAN_POINT ( 'NONE',  ( 84.99141033049929206, 2.891338577806874088, -0.4625859348280507155 ) ) ;
#23611=CARTESIAN_POINT ( 'NONE',  ( 31.02916373834690944, -0.3132898623965780782, -5.049249463166630925 ) ) ;
#23615=CARTESIAN_POINT ( 'NONE',  ( -78.88273507863694078, 11.42845723122414014, -6.074662874054942208 ) ) ;
#23622=CARTESIAN_POINT ( 'NONE',  ( 24.90974289849040346, 3.541794099149180752, -0.3255497437964431917 ) ) ;
#23624=CARTESIAN_POINT ( 'NONE',  ( 25.66178649468485773, 1.154831409588704227, 4.432321438749628584 ) ) ;
#23631=CARTESIAN_POINT ( 'NONE',  ( 22.36345331109650658, 4.261471805455568251, -3.688296226855283688 ) ) ;
#23634=CARTESIAN_POINT ( 'NONE',  ( 22.31758782591801094, 6.227955964823622459, -0.6941013191108784675 ) ) ;
#23635=CARTESIAN_POINT ( 'NONE',  ( 17.55902044582588672, 11.95912233719816342, 2.500000000000000444 ) ) ;
#23636=CARTESIAN_POINT ( 'NONE',  ( -62.92837670882106238, -23.80776546975053520, -6.000000000000000000 ) ) ;
#23638=CARTESIAN_POINT ( 'NONE',  ( 84.57067941792149668, 3.126724152278200997, 0.3173792860121260051 ) ) ;
#23642=CARTESIAN_POINT ( 'NONE',  ( 21.65999089574924596, 6.756737864946346761, -2.827852530117774599 ) ) ;
#23644=CARTESIAN_POINT ( 'NONE',  ( 26.27455094472032116, -3.204942025804789818, -4.209323993755259785 ) ) ;
#23645=CARTESIAN_POINT ( 'NONE',  ( 35.86862426242751667, -2.087724560567193244, -5.804564320744471040 ) ) ;
#23647=CARTESIAN_POINT ( 'NONE',  ( 22.04842757576495771, 0.2902497289493954358, -7.510401919737763166 ) ) ;
#23651=CARTESIAN_POINT ( 'NONE',  ( 33.62635108579966925, -1.235446387465426898, 5.454603361950056239 ) ) ;
#23653=CARTESIAN_POINT ( 'NONE',  ( -5.316495087772349137, -32.84709638682603838, 6.000000000000000888 ) ) ;
#23658=CARTESIAN_POINT ( 'NONE',  ( 27.81619187117563996, 1.844502997120055054, 3.906579784159712965 ) ) ;
#23660=CARTESIAN_POINT ( 'NONE',  ( 87.45260826627337281, -1.934911646089722659, 3.714069959888173234 ) ) ;
#23662=DIRECTION ( 'NONE',  ( 0.000000000000000000, 0.000000000000000000, -1.000000000000000000 ) ) ;
#23673=CARTESIAN_POINT ( 'NONE',  ( 24.47679419834368275, 2.965539177225203105, 3.653982106517862594 ) ) ;
#23679=CARTESIAN_POINT ( 'NONE',  ( 16.02007836965137955, -3.385103570282511409, -2.706718695280325715 ) ) ;
#23682=CARTESIAN_POINT ( 'NONE',  ( 22.25539530137726274, 2.842831528157699683, -4.834828159471090459 ) ) ;
#23690=CARTESIAN_POINT ( 'NONE',  ( 85.45255010372768822, 2.373364497502822967, 3.195069691434311743 ) ) ;
#23691=CARTESIAN_POINT ( 'NONE',  ( 28.57954844588206811, 0.5947805351201630453, 5.396286122280502084 ) ) ;
#23694=CARTESIAN_POINT ( 'NONE',  ( -80.93982711156188259, -5.651589301102212026, -4.572683551290904980 ) ) ;
#23698=CARTESIAN_POINT ( 'NONE',  ( 37.07725246739935443, -2.790096878235085676, -5.993199982913866464 ) ) ;
#23701=EDGE_CURVE ( 'NONE', #21833, #8080, #39102, .T. ) ;
#23707=CARTESIAN_POINT ( 'NONE',  ( 34.13106453884969227, -3.728238084256084495, 5.351387154442956096 ) ) ;
#23710=LINE ( 'NONE', #11337, #28642 ) ;
#23715=DIRECTION ( 'NONE',  ( 0.000000000000000000, -1.000000000000000000, 0.000000000000000000 ) ) ;
#23717=LINE ( 'NONE', #24118, #37628 ) ;
#23719=CARTESIAN_POINT ( 'NONE',  ( 22.18707434479883744, 5.266624075232406277, 3.077484895491516159 ) ) ;
#23721=CARTESIAN_POINT ( 'NONE',  ( 17.92617638325606677, -3.172788574053346355, 2.962287333578757398 ) ) ;
#23727=CARTESIAN_POINT ( 'NONE',  ( 26.06497513181486880, 0.7653527817883817308, 4.421512231569668216 ) ) ;
#23728=CARTESIAN_POINT ( 'NONE',  ( 14.76731606441705402, -5.163872065058405347, -2.500000000054358740 ) ) ;
#23734=CARTESIAN_POINT ( 'NONE',  ( 39.57450465021913999, -13.08403409140692553, 6.000000000000001776 ) ) ;
#23736=CARTESIAN_POINT ( 'NONE',  ( 29.64656804624054942, -2.931097914703496787, 5.165983120431130615 ) ) ;
#23738=VERTEX_POINT ( 'NONE', #6590 ) ;
#23740=CARTESIAN_POINT ( 'NONE',  ( 22.60882170720540429, 0.2902834165949863543, -6.504415997128977445 ) ) ;
#23741=EDGE_CURVE ( 'NONE', #37831, #10017, #20964, .T. ) ;
#23745=CARTESIAN_POINT ( 'NONE',  ( -71.91962744173181932, -48.24704961926887847, 9.950992054193424252 ) ) ;
#23746=CARTESIAN_POINT ( 'NONE',  ( 20.91845615398282376, 4.580162226973405915, -2.658158748952031747 ) ) ;
#23750=DIRECTION ( 'NONE',  ( 0.000000000000000000, 0.000000000000000000, -1.000000000000000000 ) ) ;
#23753=ADVANCED_FACE ( 'NONE', ( #39465 ), #36304, .T. ) ;
#23760=CARTESIAN_POINT ( 'NONE',  ( 86.27652758060003180, -0.2533697966053802819, -5.917929974479952726 ) ) ;
#23775=CARTESIAN_POINT ( 'NONE',  ( 21.85643539959775694, 2.564233178479530917, 15.28924334870111146 ) ) ;
#23777=FACE_OUTER_BOUND ( 'NONE', #13062, .T. ) ;
#23778=CARTESIAN_POINT ( 'NONE',  ( 14.77571469133521198, -5.163876921041897106, 2.500000000713546555 ) ) ;
#23780=CARTESIAN_POINT ( 'NONE',  ( -80.18326513131566458, 10.47830472520926826, -6.103113075884769145 ) ) ;
#23785=B_SPLINE_CURVE_WITH_KNOTS ( 'NONE', 3,
 ( #6417, #30728, #25146, #37679, #18757, #14844, #9482, #15057, #2946, #24739, #37288, #18543, #2533, #34030, #9280, #2322, #8872, #40569, #40172, #2737, #34433, #22072, #34643, #36885, #28023, #27811, #40364, #27410, #39973, #18971, #12167, #8665, #11743, #24322, #9081, #6008, #12380, #21244, #33816, #21858, #31128, #31332, #3156, #37893, #35045, #11038, #9701, #26513, #38852, #25354, #12991, #32898, #4498, #23615, #23223, #20314, #36181, #39247, #10645, #35787, #7564, #451, #7765, #31947, #20119, #39043 ),
 .UNSPECIFIED., .F., .F.,
 ( 4, 2, 2, 2, 2, 2, 2, 2, 2, 2, 2, 2, 2, 2, 2, 2, 2, 2, 2, 2, 2, 2, 2, 2, 2, 2, 2, 2, 2, 2, 2, 2, 4 ),
 ( 0.04111556421994554816, 0.04237963096789508499, 0.04364369771584461488, 0.04490776446379415171, 0.04617183121174368160, 0.04869996470764277607, 0.04996403145559230596, 0.05122809820354183585, 0.05249216495149136574, 0.05375623169944089563, 0.05502029844739042552, 0.05628436519533996235, 0.05881249869123900131, 0.06007656543918852426, 0.06134063218713804722, 0.06260469893508756323, 0.06386876568303709312, 0.06513283243098660913, 0.06639689917893612514, 0.06766096592688564115, 0.06829299930086041304, 0.06892503267483519880, 0.07018909942278475644, 0.07082113279675951445, 0.07145316617073427246, 0.07271723291868376071, 0.07398129966663326285, 0.07524536641458275110, 0.07650943316253225324, 0.07777349991048174149, 0.07903756665843122975, 0.08030163340638071801, 0.08156570015433022014 ),
 .UNSPECIFIED. ) ;
#23792=CARTESIAN_POINT ( 'NONE',  ( 87.77108079546424335, -0.2309192195606523390, 3.753057804081372684 ) ) ;
#23796=CARTESIAN_POINT ( 'NONE',  ( 35.47949778313863334, -1.848513373575088714, 5.743831722591982825 ) ) ;
#23798=CARTESIAN_POINT ( 'NONE',  ( 85.12050554930138446, 2.746332700819607453, -1.966258668667607123 ) ) ;
#23810=CARTESIAN_POINT ( 'NONE',  ( 26.22005767131799914, 1.338533239893550109, 4.347865427178345676 ) ) ;
#23816=CARTESIAN_POINT ( 'NONE',  ( 82.38753728249152175, 5.816132372599501110, 5.999999999999998224 ) ) ;
#23820=( BOUNDED_SURFACE ( )  B_SPLINE_SURFACE ( 3, 2, ( 
 ( #12270, #24843, #37785 ),
 ( #9593, #37389, #19070 ),
 ( #9183, #21756, #34744 ),
 ( #3256, #15778, #34338 ) ),
 .UNSPECIFIED., .F., .F., .T. ) 
 B_SPLINE_SURFACE_WITH_KNOTS ( ( 4, 4 ),
 ( 3, 3 ),
 ( 0.005269474087521970260, 0.007542904871472735570 ),
 ( 0.000000000000000000, 1.000000000000000000 ),
 .UNSPECIFIED. ) 
 GEOMETRIC_REPRESENTATION_ITEM ( )  RATIONAL_B_SPLINE_SURFACE ( (
 ( 1.000000000000000000, 0.8929779998654624462, 1.000000000000000000),
 ( 1.000000000000000000, 0.8751601137609862358, 1.000000000000000000),
 ( 1.000000000000000000, 0.8609322455899910409, 1.000000000000000000),
 ( 1.000000000000000000, 0.8503447817689703259, 1.000000000000000000) ) ) 
 REPRESENTATION_ITEM ( '' )  SURFACE ( )  );
#23821=CARTESIAN_POINT ( 'NONE',  ( 21.82801474315459345, 4.845872665800435186, -3.845916247992467785 ) ) ;
#23822=VERTEX_POINT ( 'NONE', #1829 ) ;
#23825=CARTESIAN_POINT ( 'NONE',  ( 22.71016324673079012, -4.497379315063210647, 7.328459856909534054 ) ) ;
#23827=DIRECTION ( 'NONE',  ( 0.000000000000000000, -0.000000000000000000, -1.000000000000000000 ) ) ;
#23829=CARTESIAN_POINT ( 'NONE',  ( 85.98118993947397826, 1.447477879098551856, 5.565446759936045318 ) ) ;
#23831=ORIENTED_EDGE ( 'NONE', *, *, #33873, .T. ) ;
#23835=CARTESIAN_POINT ( 'NONE',  ( 18.24666052293414253, -3.095731080093750087, -3.016724835387484482 ) ) ;
#23837=CARTESIAN_POINT ( 'NONE',  ( 36.99184966288904519, -2.719776486114577008, -5.979870809795490239 ) ) ;
#23838=CARTESIAN_POINT ( 'NONE',  ( -70.92837670882107659, -56.35932253828835314, 0.000000000000000000 ) ) ;
#23839=CARTESIAN_POINT ( 'NONE',  ( 24.67432665942473236, 0.7056974025990818689, -4.794247048528192501 ) ) ;
#23846=ORIENTED_EDGE ( 'NONE', *, *, #24370, .F. ) ;
#23847=CARTESIAN_POINT ( 'NONE',  ( 33.94687777511632021, -0.4864967322304499797, 5.119561820975840227 ) ) ;
#23849=CARTESIAN_POINT ( 'NONE',  ( 17.88642430224130209, -3.177481357815599594, -2.956548120854927575 ) ) ;
#23862=CARTESIAN_POINT ( 'NONE',  ( 23.41947422422738967, 3.389483684519994711, 3.647767087863493796 ) ) ;
#23867=FACE_OUTER_BOUND ( 'NONE', #3759, .T. ) ;
#23868=CARTESIAN_POINT ( 'NONE',  ( 18.13303797671674644, -2.853770859205107868, -3.036497144084084443 ) ) ;
#23871=AXIS2_PLACEMENT_3D ( 'NONE', #40019, #5856, #34287 ) ;
#23872=CARTESIAN_POINT ( 'NONE',  ( 21.85601462913819049, 3.177268030137100130, -4.957676561649461355 ) ) ;
#23881=CARTESIAN_POINT ( 'NONE',  ( 87.00024757794628272, 0.6349172363070331171, 4.931108601852515427 ) ) ;
#23882=B_SPLINE_CURVE_WITH_KNOTS ( 'NONE', 3,
 ( #12873, #2820, #8748, #21333, #34119, #15761, #28316, #37771, #40445, #12254, #15344, #24826, #18626, #3036, #21741, #6093, #12665, #25240, #16963, #13478, #28730, #19258 ),
 .UNSPECIFIED., .F., .F.,
 ( 4, 1, 1, 1, 1, 1, 1, 2, 2, 2, 1, 1, 2, 2, 4 ),
 ( 0.000000000000000000, 0.2500000000000843214, 0.3750000000001239009, 0.4375000000001435518, 0.4687500000001555422, 0.4843750000001613154, 0.4921875000001640355, 0.4960937500001632583, 0.5000000000001625367, 0.6250000000001404432, 0.6875000000001272316, 0.7187500000001187939, 0.7343750000001144640, 0.7500000000001101341, 1.000000000000000000 ),
 .UNSPECIFIED. ) ;
#23883=CARTESIAN_POINT ( 'NONE',  ( 30.36459403182758265, -1.672762201151555939, 6.017704416797944766 ) ) ;
#23890=CARTESIAN_POINT ( 'NONE',  ( 37.01039123596240898, -2.703883751567390359, -5.982764670703224041 ) ) ;
#23892=CARTESIAN_POINT ( 'NONE',  ( -70.92837670882012446, 0.2170085631207802901, 6.000000000001379341 ) ) ;
#23893=DIRECTION ( 'NONE',  ( 0.000000000000000000, -1.000000000000000000, -0.000000000000000000 ) ) ;
#23898=CARTESIAN_POINT ( 'NONE',  ( 33.45095132737965571, -3.771342036780488627, 5.158305224127381017 ) ) ;
#23904=VERTEX_POINT ( 'NONE', #18048 ) ;
#23908=CARTESIAN_POINT ( 'NONE',  ( -80.69880588614331884, 11.48364438412461119, 2.288095856349301016 ) ) ;
#23911=ORIENTED_EDGE ( 'NONE', *, *, #35633, .T. ) ;
#23912=CARTESIAN_POINT ( 'NONE',  ( 23.43164679671629003, 3.783403669430692062, 3.128883362209908814 ) ) ;
#23920=CARTESIAN_POINT ( 'NONE',  ( 23.58768437045748101, 0.4155699572297044120, 5.528158402111618130 ) ) ;
#23921=CARTESIAN_POINT ( 'NONE',  ( 14.75560021692665202, -5.144521063667438554, -2.500000000017701840 ) ) ;
#23929=CARTESIAN_POINT ( 'NONE',  ( 36.60794128011109905, -3.504051565419862069, -5.830873203126740734 ) ) ;
#23932=CARTESIAN_POINT ( 'NONE',  ( 36.10284116201629701, 0.9159659085930716982, 5.999999999999999112 ) ) ;
#23933=CARTESIAN_POINT ( 'NONE',  ( 23.98959816390508593, 3.209834647534565377, 4.521976212143768770 ) ) ;
#23937=CARTESIAN_POINT ( 'NONE',  ( -80.91065676098011750, -6.597313057213483489, -0.5950503846463429669 ) ) ;
#23938=CARTESIAN_POINT ( 'NONE',  ( 22.28822635994833945, 0.2533368339982051132, -7.122398813026761033 ) ) ;
#23942=DIRECTION ( 'NONE',  ( -0.000000000000000000, -1.000000000000000000, -0.000000000000000000 ) ) ;
#23943=CARTESIAN_POINT ( 'NONE',  ( 33.45628508796660583, -3.829382271890817258, -5.093793554038391846 ) ) ;
#23944=CARTESIAN_POINT ( 'NONE',  ( 30.80878225244670077, -3.348914835482470043, -4.960346515808566892 ) ) ;
#23946=CARTESIAN_POINT ( 'NONE',  ( -71.92070561156705821, -48.24608967860918085, 5.917785064630586511 ) ) ;
#23948=CARTESIAN_POINT ( 'NONE',  ( -73.08797875314412806, 4.425365387401466677, 10.93635685748529873 ) ) ;
#23954=ORIENTED_EDGE ( 'NONE', *, *, #33061, .T. ) ;
#23958=CARTESIAN_POINT ( 'NONE',  ( 21.71185578408363881, 6.328645931448866335, 3.192210964217056191 ) ) ;
#23962=DIRECTION ( 'NONE',  ( -0.000000000000000000, -0.000000000000000000, -1.000000000000000000 ) ) ;
#23963=VERTEX_POINT ( 'NONE', #7916 ) ;
#23967=ORIENTED_EDGE ( 'NONE', *, *, #33061, .F. ) ;
#23969=CARTESIAN_POINT ( 'NONE',  ( 17.36540201846515075, 9.558839302759881917, -2.500000000000007105 ) ) ;
#23978=CARTESIAN_POINT ( 'NONE',  ( 21.85643539959779957, 3.623429283794106670, 13.13803316603621241 ) ) ;
#23980=CARTESIAN_POINT ( 'NONE',  ( -78.36455021024127632, 10.14388467517119707, 6.697453011245038113 ) ) ;
#23982=CARTESIAN_POINT ( 'NONE',  ( 14.73442315498073540, -4.754054855475527752, 2.504681350756293945 ) ) ;
#23983=CARTESIAN_POINT ( 'NONE',  ( -78.60820997296055168, 10.22189545475253070, -6.417293082551506878 ) ) ;
#23988=CARTESIAN_POINT ( 'NONE',  ( 14.61588355500315828, 13.14117221797890345, 2.487560133874544999 ) ) ;
#23994=EDGE_LOOP ( 'NONE', ( #10791, #24968, #25466, #31033 ) ) ;
#23997=CARTESIAN_POINT ( 'NONE',  ( 36.99148392659544271, -2.973123077218505106, 5.979813727801484013 ) ) ;
#24000=CARTESIAN_POINT ( 'NONE',  ( 88.02721697999687933, -0.6980542412123691420, -4.669518943469966210 ) ) ;
#24001=CARTESIAN_POINT ( 'NONE',  ( 30.30396332325029718, -0.06004591992995000210, 5.542382567169830132 ) ) ;
#24006=CARTESIAN_POINT ( 'NONE',  ( -61.24591834330252027, -42.37473357531882812, 2.500000000000000000 ) ) ;
#24015=CARTESIAN_POINT ( 'NONE',  ( 21.74703536819586347, 0.5577694647882641688, 8.300425383226157194 ) ) ;
#24027=CARTESIAN_POINT ( 'NONE',  ( 21.72652366223498177, 6.198145607837613369, -3.240109526687368291 ) ) ;
#24031=CARTESIAN_POINT ( 'NONE',  ( 22.81652408475101979, -6.765098194116612618, -2.522738730058198264 ) ) ;
#24037=CARTESIAN_POINT ( 'NONE',  ( 84.45327006356104960, 2.923007647743876447, -2.091752339247905823 ) ) ;
#24043=CARTESIAN_POINT ( 'NONE',  ( 31.36819916996323698, -3.287745066446770892, -5.091721761760051201 ) ) ;
#24045=DIRECTION ( 'NONE',  ( 0.000000000000000000, 0.000000000000000000, -1.000000000000000000 ) ) ;
#24046=CARTESIAN_POINT ( 'NONE',  ( 25.30174877026170321, 0.8083424722246850269, -4.611467558984948312 ) ) ;
#24050=CARTESIAN_POINT ( 'NONE',  ( 31.83263240781453973, -2.965535539804599718, -5.174650181000254534 ) ) ;
#24051=ORIENTED_EDGE ( 'NONE', *, *, #34749, .T. ) ;
#24052=VERTEX_POINT ( 'NONE', #7716 ) ;
#24054=CARTESIAN_POINT ( 'NONE',  ( 34.14254696827997293, -3.849676149305037320, 5.233320676800256699 ) ) ;
#24056=CARTESIAN_POINT ( 'NONE',  ( -69.42837670882107659, -47.11702805680359063, 9.886859966642603581 ) ) ;
#24057=CARTESIAN_POINT ( 'NONE',  ( 18.44527402623563361, -3.111956244387396264, -3.036883180503353596 ) ) ;
#24065=CARTESIAN_POINT ( 'NONE',  ( 14.77500745536057813, -5.175466302041957789, 2.500000552286355759 ) ) ;
#24069=CARTESIAN_POINT ( 'NONE',  ( 22.37319937022849814, 4.167743866275963605, 3.748729264894208324 ) ) ;
#24081=CARTESIAN_POINT ( 'NONE',  ( 23.88986409409178790, 2.649682191105962037, -4.076355408754036347 ) ) ;
#24089=CARTESIAN_POINT ( 'NONE',  ( 85.32384696181071604, 2.517929975123688990, -2.669340390032339361 ) ) ;
#24090=CARTESIAN_POINT ( 'NONE',  ( 29.67925625648019405, 0.9272574953382407559, 4.669903954941619695 ) ) ;
#24095=CARTESIAN_POINT ( 'NONE',  ( 34.98303455028736408, -1.566528556295725849, -5.666346628096917470 ) ) ;
#24106=CARTESIAN_POINT ( 'NONE',  ( 32.03504567309566653, 0.1963253013062704611, 4.819203286259713614 ) ) ;
#24115=CARTESIAN_POINT ( 'NONE',  ( 86.46043323462474461, 1.241262327860113590, 4.894917242394325463 ) ) ;
#24117=DIRECTION ( 'NONE',  ( 0.000000000000000000, 1.000000000000000000, 0.000000000000000000 ) ) ;
#24118=CARTESIAN_POINT ( 'NONE',  ( -7.890026461918812295, -6.626103207857777159E-16, 6.000000000000000000 ) ) ;
#24120=CARTESIAN_POINT ( 'NONE',  ( 22.18852649867165283, 5.259174019323452853, 3.082925981170793861 ) ) ;
#24122=DIRECTION ( 'NONE',  ( -0.000000000000000000, -0.000000000000000000, -1.000000000000000000 ) ) ;
#24125=CARTESIAN_POINT ( 'NONE',  ( -4.220127061295482087E-17, 0.7293679304675931840, -6.000000000000000000 ) ) ;
#24129=CARTESIAN_POINT ( 'NONE',  ( 27.43541126664922558, 0.9752269244486642119, 4.488355539249689663 ) ) ;
#24130=CARTESIAN_POINT ( 'NONE',  ( 14.62203240282402206, -4.616478718678312276, -2.500000000000228706 ) ) ;
#24142=CARTESIAN_POINT ( 'NONE',  ( 26.56634348862415251, 2.991955253353971500, -0.5426703667890996341 ) ) ;
#24143=FACE_OUTER_BOUND ( 'NONE', #20441, .T. ) ;
#24146=CARTESIAN_POINT ( 'NONE',  ( -80.91031161377242142, -5.699894439238892829, -0.6008404087775668367 ) ) ;
#24148=CARTESIAN_POINT ( 'NONE',  ( 4.938390203311415748E-15, -42.37473357531882101, 6.000000000000000000 ) ) ;
#24154=CARTESIAN_POINT ( 'NONE',  ( 33.94509347138731670, -0.4898356627277217767, -5.123723072070831996 ) ) ;
#24160=LINE ( 'NONE', #20455, #10176 ) ;
#24163=AXIS2_PLACEMENT_3D ( 'NONE', #31665, #19096, #6551 ) ;
#24165=CARTESIAN_POINT ( 'NONE',  ( 22.52490398424734863, 1.961233960008371024, -5.344660709420910649 ) ) ;
#24169=VERTEX_POINT ( 'NONE', #34487 ) ;
#24175=VERTEX_POINT ( 'NONE', #37537 ) ;
#24182=CARTESIAN_POINT ( 'NONE',  ( 24.42597585396890025, 3.174433883044760929, 3.223073399387599736 ) ) ;
#24184=EDGE_CURVE ( 'NONE', #615, #37655, #15049, .T. ) ;
#24187=CARTESIAN_POINT ( 'NONE',  ( 17.20447544827797515, 12.11625409491893812, -2.500000000000000444 ) ) ;
#24190=CARTESIAN_POINT ( 'NONE',  ( 8.290806648384990041, 0.000000000000000000, 6.000000000000000000 ) ) ;
#24192=CARTESIAN_POINT ( 'NONE',  ( 21.85643539959776760, -1.092963988217814375, -14.35370713741404458 ) ) ;
#24195=CARTESIAN_POINT ( 'NONE',  ( -79.25269282065100640, 11.47373787457623884, 5.555836242586228657 ) ) ;
#24196=CARTESIAN_POINT ( 'NONE',  ( 14.69276469947978647, -4.522233606460802413, 2.500000000000264233 ) ) ;
#24197=CARTESIAN_POINT ( 'NONE',  ( -75.90835578683964968, 8.772181813903891623, -10.10645397056114803 ) ) ;
#24203=CARTESIAN_POINT ( 'NONE',  ( -70.12815439591902589, -0.1689404852770337306, 9.968370014334123397 ) ) ;
#24207=CARTESIAN_POINT ( 'NONE',  ( 86.80189613381685376, 0.8577149926806704183, 5.030330955187197972 ) ) ;
#24210=AXIS2_PLACEMENT_3D ( 'NONE', #20745, #21169, #27131 ) ;
#24212=CARTESIAN_POINT ( 'NONE',  ( 35.78817461119013643, -3.222426957731786334, 5.792008206986667851 ) ) ;
#24216=CARTESIAN_POINT ( 'NONE',  ( 84.97295377430323526, 2.662001904288300302, 3.416982328422734305 ) ) ;
#24219=DIRECTION ( 'NONE',  ( 1.385724075720358314E-16, -1.000000000000000000, 0.000000000000000000 ) ) ;
#24220=CARTESIAN_POINT ( 'NONE',  ( 33.45855146796573365, -3.830112298179899177, 5.093503661137224192 ) ) ;
#24223=EDGE_LOOP ( 'NONE', ( #26368, #21856, #21782, #32104, #22260, #10469, #33157 ) ) ;
#24229=CARTESIAN_POINT ( 'NONE',  ( 23.60520478173619807, 0.4415638201438380483, 5.510117418379326892 ) ) ;
#24240=ORIENTED_EDGE ( 'NONE', *, *, #38755, .F. ) ;
#24242=CARTESIAN_POINT ( 'NONE',  ( 24.08269697565317813, 2.216436711090640888, -5.807619368686713024 ) ) ;
#24243=LINE ( 'NONE', #5515, #8418 ) ;
#24246=CARTESIAN_POINT ( 'NONE',  ( 86.54029261786013194, -0.3196574014320466284, 5.877194713501632251 ) ) ;
#24251=AXIS2_PLACEMENT_3D ( 'NONE', #35341, #37989, #19470 ) ;
#24254=CARTESIAN_POINT ( 'NONE',  ( 33.13127733337127978, -3.703616631181526397, -5.170032777214017550 ) ) ;
#24256=PLANE ( 'NONE',  #20055 ) ;
#24259=CARTESIAN_POINT ( 'NONE',  ( 32.77846936337113704, -0.9351094977892036031, 5.322270913068036791 ) ) ;
#24263=VECTOR ( 'NONE', #15022, 1000.000000000000000 ) ;
#24267=CARTESIAN_POINT ( 'NONE',  ( 33.11406552165681916, -0.1504008805997818499, 4.940950335661676185 ) ) ;
#24270=CARTESIAN_POINT ( 'NONE',  ( 25.55635707441696880, -2.736503067813388590, 4.195085622931020275 ) ) ;
#24282=CARTESIAN_POINT ( 'NONE',  ( 22.24827523181307143, 3.072553326788747707, 4.656571929184647907 ) ) ;
#24288=CARTESIAN_POINT ( 'NONE',  ( 15.73410864315090762, -3.515507921127240643, -2.662086203255957351 ) ) ;
#24291=CARTESIAN_POINT ( 'NONE',  ( 22.83256966555022771, 3.311254434957428217, -4.047795553463541474 ) ) ;
#24293=CARTESIAN_POINT ( 'NONE',  ( 21.85643539959776760, 9.535790418011023561, -9.299971273199719946 ) ) ;
#24299=CARTESIAN_POINT ( 'NONE',  ( 86.12362567153361681, 1.619580568575353485, 4.895344567657775592 ) ) ;
#24300=CARTESIAN_POINT ( 'NONE',  ( 13.52694889643372278, 17.29870644234688370, 2.500000000000000000 ) ) ;
#24303=CARTESIAN_POINT ( 'NONE',  ( 17.15375077719031438, -3.245341706395144410, 2.857006424881785911 ) ) ;
#24305=CARTESIAN_POINT ( 'NONE',  ( 36.64653950724111553, -2.460867072496613517, -5.925976808648774075 ) ) ;
#24311=CARTESIAN_POINT ( 'NONE',  ( -69.42837670882107659, -47.11702805680359063, 5.809475019311128641 ) ) ;
#24313=ORIENTED_EDGE ( 'NONE', *, *, #20671, .F. ) ;
#24314=CARTESIAN_POINT ( 'NONE',  ( 37.09095381799627944, -3.108752521506979338, 5.978566616837214909 ) ) ;
#24318=DIRECTION ( 'NONE',  ( 1.000000000000000000, 0.000000000000000000, 0.000000000000000000 ) ) ;
#24319=ORIENTED_EDGE ( 'NONE', *, *, #33873, .F. ) ;
#24322=CARTESIAN_POINT ( 'NONE',  ( -72.37659067963534198, 5.886899662738341199, -9.895437931856170266 ) ) ;
#24329=CARTESIAN_POINT ( 'NONE',  ( 23.72357854948797140, 3.529942696455977025, 3.269053811182030866 ) ) ;
#24331=CARTESIAN_POINT ( 'NONE',  ( -72.84815947045233031, 2.429809908903243443, 12.50000000000000000 ) ) ;
#24333=VERTEX_POINT ( 'NONE', #22925 ) ;
#24335=ORIENTED_EDGE ( 'NONE', *, *, #23701, .T. ) ;
#24337=CARTESIAN_POINT ( 'NONE',  ( 25.40538314162099809, 0.6392986327759521137, 4.601631931458681990 ) ) ;
#24342=ORIENTED_EDGE ( 'NONE', *, *, #38525, .F. ) ;
#24348=CARTESIAN_POINT ( 'NONE',  ( 31.72291873093343284, -3.714249907566092634, 4.801291842747894556 ) ) ;
#24349=CARTESIAN_POINT ( 'NONE',  ( 14.62597543585568793, -4.708289007715579899, -2.500000000000003997 ) ) ;
#24352=CARTESIAN_POINT ( 'NONE',  ( 21.79667146064388206, 0.2347865111010814521, -8.327566971649902783 ) ) ;
#24353=LINE ( 'NONE', #37516, #10357 ) ;
#24358=VECTOR ( 'NONE', #35481, 1000.000000000000000 ) ;
#24360=CARTESIAN_POINT ( 'NONE',  ( 36.47577210302739559, -3.472112016856729877, -5.836390310795054326 ) ) ;
#24362=CARTESIAN_POINT ( 'NONE',  ( 27.06148380711046642, 1.345426480462052821, -4.421175649609593528 ) ) ;
#24366=CARTESIAN_POINT ( 'NONE',  ( -74.47588865074813214, 7.309999117102635502, 10.65416010709459194 ) ) ;
#24368=CARTESIAN_POINT ( 'NONE',  ( 14.73396276735570787, -4.758955132908557317, -2.504555023738491037 ) ) ;
#24369=CARTESIAN_POINT ( 'NONE',  ( 24.83719285264605148, 2.308780662792858429, -4.092877271418466023 ) ) ;
#24370=EDGE_CURVE ( 'NONE', #11160, #13546, #22373, .T. ) ;
#24386=CARTESIAN_POINT ( 'NONE',  ( 23.43766775396862911, 3.794989907829951825, 3.097544954452251087 ) ) ;
#24388=CIRCLE ( 'NONE', #11874, 15.73502530973474478 ) ;
#24392=CARTESIAN_POINT ( 'NONE',  ( 17.42606438386317791, 12.01804243839431585, -2.500000000000000444 ) ) ;
#24394=EDGE_CURVE ( 'NONE', #28666, #22380, #272, .T. ) ;
#24398=CARTESIAN_POINT ( 'NONE',  ( 18.51830382657068341, 13.21772817956447277, 2.500000000000000444 ) ) ;
#24399=CARTESIAN_POINT ( 'NONE',  ( 21.85643539959773207, -2.370478073490382531, -12.58538558043069600 ) ) ;
#24400=ORIENTED_EDGE ( 'NONE', *, *, #15605, .T. ) ;
#24402=CARTESIAN_POINT ( 'NONE',  ( 37.03382163445419906, -3.210012919756318528, 5.955199199487100969 ) ) ;
#24403=AXIS2_PLACEMENT_3D ( 'NONE', #33222, #39995, #13513 ) ;
#24405=LINE ( 'NONE', #9158, #26101 ) ;
#24406=CARTESIAN_POINT ( 'NONE',  ( -75.50324732371151981, 10.04197788123400414, -8.898607310640866075 ) ) ;
#24410=CARTESIAN_POINT ( 'NONE',  ( 14.63934257578662290, 12.89545353563754304, 2.491221481426366680 ) ) ;
#24417=CARTESIAN_POINT ( 'NONE',  ( 24.42049692777757741, 2.955061417206801710, -3.687805831412614310 ) ) ;
#24419=EDGE_LOOP ( 'NONE', ( #23954, #12188, #3544 ) ) ;
#24421=CARTESIAN_POINT ( 'NONE',  ( 36.43211955938636493, -3.203076905710052102, 5.892511390020157336 ) ) ;
#24424=CARTESIAN_POINT ( 'NONE',  ( 87.14327233159831110, 0.3315334873356338141, 5.689878492676547772 ) ) ;
#24443=EDGE_CURVE ( 'NONE', #18492, #28666, #9752, .T. ) ;
#24445=CARTESIAN_POINT ( 'NONE',  ( 23.15428476648550671, 3.937122355327012269, -3.239522367696926253 ) ) ;
#24449=CARTESIAN_POINT ( 'NONE',  ( 23.92064240948634790, 4.179079982057642972, -0.5982227118658990372 ) ) ;
#24453=CARTESIAN_POINT ( 'NONE',  ( 85.50109956362166486, 1.391598633704343113, -5.555888502831813902 ) ) ;
#24459=CARTESIAN_POINT ( 'NONE',  ( 17.03662858313420259, -3.187941445456853096, -2.857527714150005504 ) ) ;
#24461=CARTESIAN_POINT ( 'NONE',  ( 85.87360894986291271, 0.4889004943431661254, 5.985809846730117734 ) ) ;
#24469=CARTESIAN_POINT ( 'NONE',  ( 36.88857704436834695, -3.352795655385050200, 5.910168394248842993 ) ) ;
#24470=CARTESIAN_POINT ( 'NONE',  ( 14.72021916802428443, 13.05558383789484900, -2.500000000000000000 ) ) ;
#24484=CARTESIAN_POINT ( 'NONE',  ( 22.44694882813763570, 3.194566178373594134, 4.411186854447311845 ) ) ;
#24485=CARTESIAN_POINT ( 'NONE',  ( 14.75988012747214206, 13.12337194104200577, 2.499999999999984901 ) ) ;
#24489=EDGE_CURVE ( 'NONE', #9007, #32259, #40477, .T. ) ;
#24497=CARTESIAN_POINT ( 'NONE',  ( 24.14002715383752573, 2.925673756400894110, -3.791870614624193170 ) ) ;
#24501=CARTESIAN_POINT ( 'NONE',  ( 21.85643539959777115, -1.425092139247138734, 16.06258187428232986 ) ) ;
#24506=CARTESIAN_POINT ( 'NONE',  ( 85.21894181876761820, 2.635764410888131959, 2.550537924818469637 ) ) ;
#24510=ORIENTED_EDGE ( 'NONE', *, *, #35578, .T. ) ;
#24511=CARTESIAN_POINT ( 'NONE',  ( 28.90011140548632440, -3.472380137462792948, 4.526229835286804892 ) ) ;
#24513=CARTESIAN_POINT ( 'NONE',  ( 34.13594578679055758, -3.137541451073295740, -5.534137939634120151 ) ) ;
#24515=B_SPLINE_CURVE_WITH_KNOTS ( 'NONE', 3,
 ( #19274, #31034, #6111, #21562, #19072, #18446, #15973, #18648, #9595, #28747, #27917, #37998, #6725, #28538, #37185, #9798, #37391, #25259, #6315, #18863, #22177, #31639, #22381, #3652, #2841, #150, #40463, #3053, #3460, #24632, #31231, #34748, #24847, #12272, #348, #557, #8975, #31841, #34137, #12891, #34341, #5907, #15361, #31436, #9185, #25455, #16180, #21758, #15573, #28334, #6525, #34945, #28127, #3258, #12485, #25054, #37586, #9383, #21969, #34541, #15782, #12681, #19874, #6918, #35347, #13898, #9997, #4244, #29548, #38198, #22579, #10402 ),
 .UNSPECIFIED., .F., .F.,
 ( 4, 2, 2, 1, 2, 2, 2, 1, 2, 2, 2, 1, 1, 2, 2, 2, 2, 2, 1, 2, 2, 1, 1, 1, 1, 1, 2, 2, 2, 2, 1, 1, 1, 1, 2, 2, 2, 1, 1, 1, 1, 1, 1, 2, 2, 4 ),
 ( 0.000000000000000000, 0.03125000000000544009, 0.04687500000000813932, 0.05468750000000939526, 0.05859375000001094957, 0.06250000000001250389, 0.07812500000001883216, 0.08593750000002287059, 0.08984375000002582656, 0.09375000000002878253, 0.1093750000000364153, 0.1171875000000392741, 0.1210937500000393574, 0.1230468750000377753, 0.1250000000000361655, 0.1562499999999986955, 0.1640624999999889810, 0.1718749999999792666, 0.1874999999999598377, 0.1953124999999492351, 0.2031249999999386324, 0.2187499999999198419, 0.2343749999999010514, 0.2421874999998926692, 0.2460937499998885336, 0.2480468749998864797, 0.2490234374998846478, 0.2499999999998828160, 0.3749999999999580336, 0.4374999999999957256, 0.4687500000000153211, 0.4843750000000243694, 0.4921875000000288658, 0.4960937500000311418, 0.4980468750000315858, 0.5000000000000319744, 0.6249999999999867883, 0.6874999999999652500, 0.7187499999999533706, 0.7343749999999473754, 0.7421874999999458211, 0.7460937499999450440, 0.7480468749999459321, 0.7490234374999463762, 0.7499999999999469313, 1.000000000000000000 ),
 .UNSPECIFIED. ) ;
#24522=CARTESIAN_POINT ( 'NONE',  ( 35.19021350240149104, -1.105041489952045985, 5.467004813264366270 ) ) ;
#24525=CARTESIAN_POINT ( 'NONE',  ( -71.92837670882107659, -0.7829914368874778541, 9.949874371066204759 ) ) ;
#24527=ORIENTED_EDGE ( 'NONE', *, *, #22931, .F. ) ;
#24535=CARTESIAN_POINT ( 'NONE',  ( 22.21849618742577093, 5.138564923484444158, 3.154761569516522979 ) ) ;
#24542=CARTESIAN_POINT ( 'NONE',  ( 14.68628669673910458, -4.762509258086469188, -2.500000000000608402 ) ) ;
#24549=AXIS2_PLACEMENT_3D ( 'NONE', #1540, #11179, #10778 ) ;
#24550=DIRECTION ( 'NONE',  ( -0.000000000000000000, -0.000000000000000000, -1.000000000000000000 ) ) ;
#24555=ORIENTED_EDGE ( 'NONE', *, *, #13992, .T. ) ;
#24556=CARTESIAN_POINT ( 'NONE',  ( 29.58677136987063960, -0.8116067495284342570, -6.002319972564883699 ) ) ;
#24560=CARTESIAN_POINT ( 'NONE',  ( 26.03637107960420849, 0.8233936766560462361, -4.423249474891364663 ) ) ;
#24565=FACE_OUTER_BOUND ( 'NONE', #2484, .T. ) ;
#24568=CARTESIAN_POINT ( 'NONE',  ( 33.08021759589966848, -0.2095332219197587609, -5.024918305154424836 ) ) ;
#24570=CARTESIAN_POINT ( 'NONE',  ( 70.22075738143423962, -4.730509630324903902, -5.999999999999999112 ) ) ;
#24577=CARTESIAN_POINT ( 'NONE',  ( 24.51166757111680994, 1.776401893265235676, -4.441653616560364171 ) ) ;
#24580=B_SPLINE_CURVE_WITH_KNOTS ( 'NONE', 3,
 ( #34717, #31609, #25021, #37558 ),
 .UNSPECIFIED., .F., .F.,
 ( 4, 4 ),
 ( 0.6850855086804076288, 1.000000000000000000 ),
 .UNSPECIFIED. ) ;
#24590=CARTESIAN_POINT ( 'NONE',  ( 24.07141319651289280, 3.351886934043508681, 3.193749788468272843 ) ) ;
#24595=CARTESIAN_POINT ( 'NONE',  ( 15.67275388389877833, 8.062146399472998937, -3.484635956154243264 ) ) ;
#24603=CARTESIAN_POINT ( 'NONE',  ( 21.85643539959775694, 0.06084538214464753347, 12.63034898425695296 ) ) ;
#24605=CARTESIAN_POINT ( 'NONE',  ( -79.19778882647081275, 10.32772801069598678, 7.503737277772331460 ) ) ;
#24610=CARTESIAN_POINT ( 'NONE',  ( 33.43921609458320177, -3.587388448609353020, -5.336552248008303856 ) ) ;
#24611=CARTESIAN_POINT ( 'NONE',  ( 36.88807738535138014, -3.351649916613822278, -5.910501343806321195 ) ) ;
#24619=CARTESIAN_POINT ( 'NONE',  ( 29.11756219249926758, -3.932895944232090546, -4.208584474947498322 ) ) ;
#24620=CARTESIAN_POINT ( 'NONE',  ( 26.82849101641929579, 1.498248074508184091, -4.376000038070654519 ) ) ;
#24621=ORIENTED_EDGE ( 'NONE', *, *, #18405, .F. ) ;
#24622=ORIENTED_EDGE ( 'NONE', *, *, #15578, .F. ) ;
#24624=CARTESIAN_POINT ( 'NONE',  ( 35.79596573831845063, -3.408953143014849196, 5.784744517605735936 ) ) ;
#24627=DIRECTION ( 'NONE',  ( -0.000000000000000000, -0.000000000000000000, -1.000000000000000000 ) ) ;
#24628=CARTESIAN_POINT ( 'NONE',  ( 84.57490107788032674, 3.121871263001978924, -0.4841835102440271710 ) ) ;
#24630=CARTESIAN_POINT ( 'NONE',  ( 33.46397865298071395, -3.088978469517898340, -5.429261216816389179 ) ) ;
#24632=CARTESIAN_POINT ( 'NONE',  ( 24.41800086858311758, 2.826335870316004861, 3.825790758725832408 ) ) ;
#24651=CARTESIAN_POINT ( 'NONE',  ( 26.40632256607097972, -4.828918925250113681, 3.355911752401763426 ) ) ;
#24653=CARTESIAN_POINT ( 'NONE',  ( 33.89851005511244608, -5.475126146365266955, 0.2339871931363489144 ) ) ;
#24654=CARTESIAN_POINT ( 'NONE',  ( 23.14945514779503100, 3.965360163098824664, -3.203264653297140274 ) ) ;
#24657=CARTESIAN_POINT ( 'NONE',  ( 24.87384391889476021, -2.282154821806516409, -6.307558310060713325 ) ) ;
#24660=CARTESIAN_POINT ( 'NONE',  ( 87.94553049950697243, -1.849565313017166535, -3.579236442506480653 ) ) ;
#24674=CARTESIAN_POINT ( 'NONE',  ( 36.44665502137046786, -2.355026295696516669, 5.894780000404371556 ) ) ;
#24676=EDGE_CURVE ( 'NONE', #29224, #32959, #23785, .T. ) ;
#24677=CARTESIAN_POINT ( 'NONE',  ( 86.66388813748453401, 1.012732124415782531, -5.000054679117940104 ) ) ;
#24680=CARTESIAN_POINT ( 'NONE',  ( 25.73464818478049665, 2.638161164068132170, 3.516476401580347133 ) ) ;
#24681=CARTESIAN_POINT ( 'NONE',  ( 28.29734904859521194, -2.858939882045380632, 4.622883711642937321 ) ) ;
#24682=ADVANCED_FACE ( 'NONE', ( #4297 ), #25556, .T. ) ;
#24686=ORIENTED_EDGE ( 'NONE', *, *, #24891, .F. ) ;
#24690=EDGE_LOOP ( 'NONE', ( #11484, #11534, #31044, #3318, #4919, #15216, #13846, #38555, #364, #10574, #40523, #26065, #2531, #15480, #26640, #3351, #23363, #38256, #1259, #37964, #12990, #10266, #6362, #28821, #5032, #10302, #24319 ) ) ;
#24693=ORIENTED_EDGE ( 'NONE', *, *, #30305, .T. ) ;
#24694=CARTESIAN_POINT ( 'NONE',  ( 22.72517738501652573, 2.451757356526896636, 4.776331650956242569 ) ) ;
#24696=VERTEX_POINT ( 'NONE', #7962 ) ;
#24700=CIRCLE ( 'NONE', #37208, 7.744449365083023729 ) ;
#24708=CARTESIAN_POINT ( 'NONE',  ( 22.22567626914783290, 3.610917974856977075, -4.269881377294811209 ) ) ;
#24711=CARTESIAN_POINT ( 'NONE',  ( 21.85643539959776760, -1.092963988217814375, -14.35370713741404458 ) ) ;
#24712=CARTESIAN_POINT ( 'NONE',  ( -58.92473026143643722, -52.43948302755219260, 2.500000000000000000 ) ) ;
#24715=CARTESIAN_POINT ( 'NONE',  ( 86.68816865751659861, 0.9854590918928021193, 5.166709667929270999 ) ) ;
#24718=CARTESIAN_POINT ( 'NONE',  ( 28.89421610208889746, -3.378331890283770012, 4.594240448401521348 ) ) ;
#24720=CARTESIAN_POINT ( 'NONE',  ( 37.04404980618738819, -2.893053985391248251, -5.988017904622426890 ) ) ;
#24724=CARTESIAN_POINT ( 'NONE',  ( 22.01541346579904967, 4.834729283906541220, -3.642368534677343117 ) ) ;
#24727=VECTOR ( 'NONE', #39431, 1000.000000000000000 ) ;
#24730=CARTESIAN_POINT ( 'NONE',  ( 32.00271079493634119, 0.1412851624054302091, 4.903334175247278992 ) ) ;
#24737=EDGE_LOOP ( 'NONE', ( #40217, #25095, #30875, #30320 ) ) ;
#24738=CARTESIAN_POINT ( 'NONE',  ( 87.74971820199947103, -0.2069237406511922894, -3.800190472810109021 ) ) ;
#24739=CARTESIAN_POINT ( 'NONE',  ( -78.94357670570525443, -6.586313634853134147, -6.037452900681159917 ) ) ;
#24740=CARTESIAN_POINT ( 'NONE',  ( 19.21387499064117321, 6.947138423917541772, 3.205187900248952726 ) ) ;
#24742=DIRECTION ( 'NONE',  ( 0.9999026450364576490, 0.01395351027862084051, 0.000000000000000000 ) ) ;
#24745=CARTESIAN_POINT ( 'NONE',  ( 22.01556798311525753, 5.489466605003165967, 3.155826305233227824 ) ) ;
#24749=ORIENTED_EDGE ( 'NONE', *, *, #17117, .T. ) ;
#24763=DIRECTION ( 'NONE',  ( 1.000000000000000000, 0.000000000000000000, 0.000000000000000000 ) ) ;
#24765=CARTESIAN_POINT ( 'NONE',  ( 31.71671097226645131, -1.585248588153130855, -6.002663613118158992 ) ) ;
#24770=CARTESIAN_POINT ( 'NONE',  ( 26.02598813970154623, 0.8351557787169782143, -4.424076136248003444 ) ) ;
#24773=ORIENTED_EDGE ( 'NONE', *, *, #22977, .F. ) ;
#24775=DIRECTION ( 'NONE',  ( 1.165409145176970240E-16, -1.000000000000000000, 0.000000000000000000 ) ) ;
#24778=CARTESIAN_POINT ( 'NONE',  ( 32.03508869243609070, 0.1963088816440640705, -4.819211608773691147 ) ) ;
#24786=CARTESIAN_POINT ( 'NONE',  ( 86.43572624768425783, -0.5192074800720990480, -5.777013305174518720 ) ) ;
#24788=CARTESIAN_POINT ( 'NONE',  ( 21.81178528484681323, 1.722486916688236835, -6.429858153412585153 ) ) ;
#24790=CARTESIAN_POINT ( 'NONE',  ( -12.99139449055068241, -10.90558813203967148, -2.500000000000000000 ) ) ;
#24791=ORIENTED_EDGE ( 'NONE', *, *, #13402, .F. ) ;
#24796=VERTEX_POINT ( 'NONE', #24006 ) ;
#24797=CARTESIAN_POINT ( 'NONE',  ( 87.32189673294487875, -1.771757446153727322, -4.160567758657673920 ) ) ;
#24802=AXIS2_PLACEMENT_3D ( 'NONE', #31008, #12457, #15753 ) ;
#24806=CARTESIAN_POINT ( 'NONE',  ( 22.38241241717832608, 4.945970055669522303, 3.038707014936568029 ) ) ;
#24807=CARTESIAN_POINT ( 'NONE',  ( 22.20101428496644402, -3.080863327041267752, 3.573976167030509021 ) ) ;
#24813=ORIENTED_EDGE ( 'NONE', *, *, #31116, .T. ) ;
#24816=CARTESIAN_POINT ( 'NONE',  ( 21.85643539959779247, -11.31796667593991401, 0.7532527802845886411 ) ) ;
#24818=CARTESIAN_POINT ( 'NONE',  ( -72.95667172690721713, 3.805589226921943791, 9.852272255005502188 ) ) ;
#24819=CARTESIAN_POINT ( 'NONE',  ( 36.61039225523681040, -3.503863859546586745, 5.830862488035224445 ) ) ;
#24820=AXIS2_PLACEMENT_3D ( 'NONE', #21372, #23827, #30433 ) ;
#24822=CARTESIAN_POINT ( 'NONE',  ( 29.49012604331536025, 1.222189331997720618, -4.216495775964309800 ) ) ;
#24824=CARTESIAN_POINT ( 'NONE',  ( 15.57083851783882444, 11.09451738654227171, 2.625278935214002018 ) ) ;
#24826=CARTESIAN_POINT ( 'NONE',  ( 29.72221670659310178, -3.784665454809892360, 4.453569354697067162 ) ) ;
#24827=CARTESIAN_POINT ( 'NONE',  ( 14.62586668347152496, -4.707709139745178462, 2.499999999999999556 ) ) ;
#24831=CARTESIAN_POINT ( 'NONE',  ( 21.73802686818168439, 0.3490801365243696996, -8.770837729082545664 ) ) ;
#24832=CARTESIAN_POINT ( 'NONE',  ( 36.75577213747256167, -1.983309010297000130, -5.827804699962920054 ) ) ;
#24833=CARTESIAN_POINT ( 'NONE',  ( 24.49910823378019842, 2.769216814238300017, -3.858631695855636590 ) ) ;
#24836=CARTESIAN_POINT ( 'NONE',  ( 36.14935728473858489, -3.245521681047676577, 5.848379498429883583 ) ) ;
#24837=CARTESIAN_POINT ( 'NONE',  ( -12.99139449055068241, -10.90558813203967148, -2.500000000000000000 ) ) ;
#24840=CARTESIAN_POINT ( 'NONE',  ( 88.76896161869186130, -1.545781173472005943, 2.128395682968124092 ) ) ;
#24843=CARTESIAN_POINT ( 'NONE',  ( 22.47913989204488061, 3.956929407484332195, 2.823518125048976923 ) ) ;
#24845=AXIS2_PLACEMENT_3D ( 'NONE', #8326, #39844, #1989 ) ;
#24847=CARTESIAN_POINT ( 'NONE',  ( 24.47171158531734392, 2.787145917774926929, 3.848838691513146948 ) ) ;
#24848=CARTESIAN_POINT ( 'NONE',  ( -7.890026461918810519, -29.56993018339340651, -6.000000000000000000 ) ) ;
#24866=CARTESIAN_POINT ( 'NONE',  ( 24.67792551878487117, 2.994442889702503940, -3.478280344776563560 ) ) ;
#24870=CARTESIAN_POINT ( 'NONE',  ( 24.99136039731803294, -2.601164552868876267, 6.036718378868273227 ) ) ;
#24871=CARTESIAN_POINT ( 'NONE',  ( -80.58693949271321344, -5.694496834616916026, -2.621342879253132807 ) ) ;
#24874=CARTESIAN_POINT ( 'NONE',  ( 85.94684271633954609, 0.9790069142357779031, 5.868308835085408681 ) ) ;
#24875=CARTESIAN_POINT ( 'NONE',  ( 18.29979634815094869, 8.276402169532444120, 2.983512989312166130 ) ) ;
#24881=EDGE_CURVE ( 'NONE', #40670, #10861, #3582, .T. ) ;
#24882=CARTESIAN_POINT ( 'NONE',  ( -70.92837670882107659, 13.87661300689599742, 0.000000000000000000 ) ) ;
#24884=CARTESIAN_POINT ( 'NONE',  ( 25.29478483175916637, 1.731669011002412661, -4.154260948315759983 ) ) ;
#24885=CARTESIAN_POINT ( 'NONE',  ( 85.57577930415899914, 1.015208198401525541, 5.782835925834406865 ) ) ;
#24888=CARTESIAN_POINT ( 'NONE',  ( 37.04356103307386405, -2.892718132023992528, 5.987941619757027212 ) ) ;
#24890=CARTESIAN_POINT ( 'NONE',  ( 87.74221684178165503, -0.1984978568185522818, 3.841619981418926244 ) ) ;
#24891=EDGE_CURVE ( 'NONE', #28300, #10739, #7612, .T. ) ;
#24894=CARTESIAN_POINT ( 'NONE',  ( -61.24591834330252027, -49.47158280949359010, 2.500000000000000000 ) ) ;
#24895=CARTESIAN_POINT ( 'NONE',  ( 18.19526664008617800, -2.845337040135758500, 3.046209432008794238 ) ) ;
#24897=CARTESIAN_POINT ( 'NONE',  ( -70.92837670882107659, 0.7293679304675899644, 0.000000000000000000 ) ) ;
#24899=CARTESIAN_POINT ( 'NONE',  ( 27.17156870755912124, -4.509646516228694502, -3.611948544634925096 ) ) ;
#24901=ORIENTED_EDGE ( 'NONE', *, *, #29347, .T. ) ;
#24906=ORIENTED_EDGE ( 'NONE', *, *, #30791, .F. ) ;
#24907=CARTESIAN_POINT ( 'NONE',  ( 22.45948225295538592, 3.011618625913302871, 4.542466585459654205 ) ) ;
#24908=CARTESIAN_POINT ( 'NONE',  ( 35.96429208010314227, -1.440254987971542500, 5.601774252719624592 ) ) ;
#24912=CARTESIAN_POINT ( 'NONE',  ( -70.05495661583778144, -0.2787455909213534810, 5.936304882227261714 ) ) ;
#24913=CARTESIAN_POINT ( 'NONE',  ( 85.60328218737365091, 2.204055066975417976, -3.382088663712862431 ) ) ;
#24918=CARTESIAN_POINT ( 'NONE',  ( 22.84217460911794007, 3.239333396839658707, -4.097155120049850829 ) ) ;
#24921=CARTESIAN_POINT ( 'NONE',  ( 21.85643539959774273, 11.87292600555486466, 1.968928953175947072 ) ) ;
#24922=CARTESIAN_POINT ( 'NONE',  ( 16.10603109340134509, 15.28195951422513232, -3.145749391471717615 ) ) ;
#24926=CARTESIAN_POINT ( 'NONE',  ( 88.42181306311033495, -0.9618525881974497871, -1.725133412809377598 ) ) ;
#24927=VERTEX_POINT ( 'NONE', #34751 ) ;
#24928=EDGE_CURVE ( 'NONE', #20545, #15995, #4238, .T. ) ;
#24931=CARTESIAN_POINT ( 'NONE',  ( 23.84193253497030440, -2.761854320939544749, 3.927508210036176450 ) ) ;
#24934=CIRCLE ( 'NONE', #7839, 27.95745752244933158 ) ;
#24935=CARTESIAN_POINT ( 'NONE',  ( 21.30795695682776625, 3.457868135880847849, -3.532020036634553328 ) ) ;
#24943=CARTESIAN_POINT ( 'NONE',  ( 33.11218242963668956, -0.1536849661985871807, 4.945614694268311240 ) ) ;
#24954=CARTESIAN_POINT ( 'NONE',  ( 24.32733003514473680, 3.133098549323304116, 3.417467526496732688 ) ) ;
#24964=CARTESIAN_POINT ( 'NONE',  ( 15.78541918192386362, 10.65456781717563040, -2.670094453781548083 ) ) ;
#24968=ORIENTED_EDGE ( 'NONE', *, *, #5070, .T. ) ;
#24974=CARTESIAN_POINT ( 'NONE',  ( 31.47838864403340509, -3.170179483860372738, -5.357953045474171283 ) ) ;
#24976=DIRECTION ( 'NONE',  ( -0.000000000000000000, -0.000000000000000000, -1.000000000000000000 ) ) ;
#24978=CARTESIAN_POINT ( 'NONE',  ( 23.08405860376734964, 0.3616624716994971123, -5.928390910620995768 ) ) ;
#24982=VERTEX_POINT ( 'NONE', #24848 ) ;
#24983=DIRECTION ( 'NONE',  ( -0.000000000000000000, -0.000000000000000000, -1.000000000000000000 ) ) ;
#24985=CARTESIAN_POINT ( 'NONE',  ( 33.46397865298071395, -3.088978469517898340, -5.429261216816389179 ) ) ;
#24986=CARTESIAN_POINT ( 'NONE',  ( 37.17919206969111912, -2.754564175853643437, -6.000958797263274747 ) ) ;
#24988=CARTESIAN_POINT ( 'NONE',  ( 30.67121742200687962, -3.774223789334631096, 4.535454642798929292 ) ) ;
#24989=CARTESIAN_POINT ( 'NONE',  ( 8.290806648384990041, -10.90558813203967148, -2.500000000000000000 ) ) ;
#24993=CARTESIAN_POINT ( 'NONE',  ( 20.70210560442331627, 10.21350129193277034, 2.500000000000000888 ) ) ;
#24995=DIRECTION ( 'NONE',  ( 0.000000000000000000, 0.000000000000000000, 1.000000000000000000 ) ) ;
#25005=CARTESIAN_POINT ( 'NONE',  ( 21.71132468300342921, 6.334557977395378181, 3.191024146652045257 ) ) ;
#25010=CARTESIAN_POINT ( 'NONE',  ( 21.73812098194953180, 0.3516627487957126319, 8.764633167989723361 ) ) ;
#25014=EDGE_CURVE ( 'NONE', #141, #20369, #31233, .T. ) ;
#25020=CARTESIAN_POINT ( 'NONE',  ( 21.85643539959774273, -8.640774161329524361, 8.772446831725494221 ) ) ;
#25021=CARTESIAN_POINT ( 'NONE',  ( 21.85643539959776760, -15.17897001446843142, 1.975458193255289263 ) ) ;
#25023=CARTESIAN_POINT ( 'NONE',  ( -71.84574099016961668, 0.8742997958048870366, 9.958011348621333525 ) ) ;
#25024=CARTESIAN_POINT ( 'NONE',  ( 36.68439403812833177, -3.468466653191531357, 5.851900647971171487 ) ) ;
#25029=CARTESIAN_POINT ( 'NONE',  ( -81.49198538235609135, 10.49122877029617129, -2.851835521983549615 ) ) ;
#25031=CARTESIAN_POINT ( 'NONE',  ( 33.11474090711421780, -0.1493249260898398267, -4.939405552518099540 ) ) ;
#25040=CARTESIAN_POINT ( 'NONE',  ( 26.97785997608481523, 1.400405612006494716, -4.405071484031834572 ) ) ;
#25042=CARTESIAN_POINT ( 'NONE',  ( 24.46830168776173053, 2.964004347679559004, -3.655893466831604766 ) ) ;
#25047=CARTESIAN_POINT ( 'NONE',  ( 31.75252458562886915, -0.4599371113500814179, 5.162147417933157456 ) ) ;
#25050=CARTESIAN_POINT ( 'NONE',  ( 88.14352194013933683, -1.303227188646099544, -4.271130342077624320 ) ) ;
#25052=CARTESIAN_POINT ( 'NONE',  ( 36.39130890773654414, -2.321068141369555082, -5.886141900820864414 ) ) ;
#25054=CARTESIAN_POINT ( 'NONE',  ( 25.65562067725548090, 2.148648913715160091, 4.136967372009855204 ) ) ;
#25055=CARTESIAN_POINT ( 'NONE',  ( 0.6783104270758654186, -48.60743831809499227, 6.000000000000000000 ) ) ;
#25056=ORIENTED_EDGE ( 'NONE', *, *, #19818, .T. ) ;
#25069=VECTOR ( 'NONE', #27992, 1000.000000000000000 ) ;
#25071=CARTESIAN_POINT ( 'NONE',  ( 24.05978824533461591, 3.343990756392554609, -3.225742063477944566 ) ) ;
#25075=ADVANCED_FACE ( 'NONE', ( #15575 ), #40682, .F. ) ;
#25076=CARTESIAN_POINT ( 'NONE',  ( 24.25791012409692371, 0.7154099962172090210, -6.776768987914707942 ) ) ;
#25078=EDGE_CURVE ( 'NONE', #17373, #21802, #1722, .T. ) ;
#25079=CARTESIAN_POINT ( 'NONE',  ( -75.83774951876674209, -5.401831623872992871, -8.713785153582826126 ) ) ;
#25080=DIRECTION ( 'NONE',  ( -0.000000000000000000, -1.000000000000000000, -0.000000000000000000 ) ) ;
#25082=CARTESIAN_POINT ( 'NONE',  ( 85.19771215196759329, 1.813128620488922760, 5.066052097874169213 ) ) ;
#25083=CARTESIAN_POINT ( 'NONE',  ( 21.05507626271832677, 6.110270179408970215, 3.370876190096979474 ) ) ;
#25090=CARTESIAN_POINT ( 'NONE',  ( 85.93940314300044747, 0.3675543374994592050, 5.999999582814343313 ) ) ;
#25092=CARTESIAN_POINT ( 'NONE',  ( 25.29564187210237591, 1.734060676602622975, 4.154394710188922701 ) ) ;
#25094=CARTESIAN_POINT ( 'NONE',  ( 87.09859342968812257, 0.5244505078549105415, -5.068689133590885909 ) ) ;
#25095=ORIENTED_EDGE ( 'NONE', *, *, #18609, .T. ) ;
#25099=CARTESIAN_POINT ( 'NONE',  ( 14.66483024702261773, 13.02142279098982591, -2.495199448944585452 ) ) ;
#25100=VERTEX_POINT ( 'NONE', #25260 ) ;
#25107=CARTESIAN_POINT ( 'NONE',  ( 23.40509239944908870, 3.763556924256647562, 3.087706618777893652 ) ) ;
#25109=CARTESIAN_POINT ( 'NONE',  ( 24.19261158263253719, 2.582287494170470321, 4.035689301652516825 ) ) ;
#25110=CARTESIAN_POINT ( 'NONE',  ( 36.16041087367324280, -1.555341878182815440, 5.654033472726598397 ) ) ;
#25119=CARTESIAN_POINT ( 'NONE',  ( 21.85424650998301743, 3.950402723962838092, -4.385458540445601905 ) ) ;
#25122=CARTESIAN_POINT ( 'NONE',  ( 21.85643539959776049, -3.688311691778667800, 15.92486026856874304 ) ) ;
#25124=EDGE_CURVE ( 'NONE', #3011, #15995, #38804, .T. ) ;
#25128=CARTESIAN_POINT ( 'NONE',  ( 85.02283808163620904, 2.856037436078923797, 1.058370034767218248 ) ) ;
#25131=CARTESIAN_POINT ( 'NONE',  ( 17.12179616700453622, -3.119139029776307304, 2.877302616401834712 ) ) ;
#25132=CARTESIAN_POINT ( 'NONE',  ( 36.78937917427825965, -3.042007186898596949, -5.948270393280488122 ) ) ;
#25135=CARTESIAN_POINT ( 'NONE',  ( -76.50589831764405346, -4.344217460646190965, 9.790531055125489601 ) ) ;
#25138=VERTEX_POINT ( 'NONE', #16770 ) ;
#25140=CARTESIAN_POINT ( 'NONE',  ( 37.18590179202365675, -2.963059666527390057, 6.000009849583459065 ) ) ;
#25141=DIRECTION ( 'NONE',  ( -0.000000000000000000, -0.000000000000000000, -1.000000000000000000 ) ) ;
#25144=ORIENTED_EDGE ( 'NONE', *, *, #29478, .F. ) ;
#25146=CARTESIAN_POINT ( 'NONE',  ( -80.83360071539431146, -6.606523484500073096, -1.436172935955783991 ) ) ;
#25147=ORIENTED_EDGE ( 'NONE', *, *, #8685, .T. ) ;
#25150=VERTEX_POINT ( 'NONE', #29744 ) ;
#25151=CARTESIAN_POINT ( 'NONE',  ( 21.72876610684703635, 6.177728964813395507, 3.247520083845313987 ) ) ;
#25158=CARTESIAN_POINT ( 'NONE',  ( -70.92837670882107659, -45.61702805680359063, 6.000000000000002665 ) ) ;
#25160=CARTESIAN_POINT ( 'NONE',  ( 15.02851297552613907, 11.88222368738628276, -2.551960934427589756 ) ) ;
#25167=LINE ( 'NONE', #40594, #10241 ) ;
#25173=CARTESIAN_POINT ( 'NONE',  ( 29.34248944929254677, 1.775380825033272991, -3.063368523016994249 ) ) ;
#25180=DIRECTION ( 'NONE',  ( 1.000000000000000000, 0.000000000000000000, 0.000000000000000000 ) ) ;
#25183=CARTESIAN_POINT ( 'NONE',  ( 29.45350768790538609, 1.169329251362175803, -4.331148011843218626 ) ) ;
#25184=CARTESIAN_POINT ( 'NONE',  ( 11.29080664838498826, -10.90558813203967148, 2.500000000000000000 ) ) ;
#25188=CARTESIAN_POINT ( 'NONE',  ( -75.68638550784876884, 8.581835957161722206, 10.20520400634731395 ) ) ;
#25189=AXIS2_PLACEMENT_3D ( 'NONE', #14303, #11813, #17585 ) ;
#25202=CARTESIAN_POINT ( 'NONE',  ( 21.85576838308406522, 3.890922448482609042, 4.421358135619450458 ) ) ;
#25210=CARTESIAN_POINT ( 'NONE',  ( 23.44095116515602228, 3.798737197898152118, 3.085442469092725126 ) ) ;
#25218=CARTESIAN_POINT ( 'NONE',  ( 25.36652333831873207, 0.7419792049594144956, 4.603917168115059688 ) ) ;
#25226=CARTESIAN_POINT ( 'NONE',  ( 21.85643539959774273, -5.916281280498693285, 11.28130179073419015 ) ) ;
#25229=CARTESIAN_POINT ( 'NONE',  ( -74.22931914091192596, 6.964638644170447535, 9.493301944864269259 ) ) ;
#25230=CARTESIAN_POINT ( 'NONE',  ( 36.65102539693456407, -3.484761920582832850, 5.842386807897074874 ) ) ;
#25234=CARTESIAN_POINT ( 'NONE',  ( -81.58802495621657158, 10.48337376234404594, -2.413223970079951375 ) ) ;
#25235=CARTESIAN_POINT ( 'NONE',  ( 28.65970685016134212, -3.315807845019801636, -4.679438410342736887 ) ) ;
#25236=CARTESIAN_POINT ( 'NONE',  ( 34.14229113142901184, -3.848523386208314356, -5.234441351989421065 ) ) ;
#25238=CARTESIAN_POINT ( 'NONE',  ( 17.87965550805309789, 8.681448112502556214, 2.924000077491842209 ) ) ;
#25240=CARTESIAN_POINT ( 'NONE',  ( 30.14635126286890809, -3.703246014866541813, 4.591439750246522067 ) ) ;
#25242=DIRECTION ( 'NONE',  ( 0.000000000000000000, 0.000000000000000000, 1.000000000000000000 ) ) ;
#25244=CARTESIAN_POINT ( 'NONE',  ( 21.74663786822173250, 0.5495625321154745668, -8.317879680902361628 ) ) ;
#25245=CARTESIAN_POINT ( 'NONE',  ( 33.45716606812183613, -3.829385970599605393, -5.093809925484540813 ) ) ;
#25246=CARTESIAN_POINT ( 'NONE',  ( 24.35712842162025282, 2.896715692034056211, -3.774200513959965697 ) ) ;
#25247=ORIENTED_EDGE ( 'NONE', *, *, #17443, .F. ) ;
#25248=ORIENTED_EDGE ( 'NONE', *, *, #18499, .T. ) ;
#25250=CARTESIAN_POINT ( 'NONE',  ( 34.76884925160979378, -3.305569524749743859, 5.632917832143227166 ) ) ;
#25253=CARTESIAN_POINT ( 'NONE',  ( 86.11108918975101290, 0.7237488529220831301, -5.972109037703948076 ) ) ;
#25255=CARTESIAN_POINT ( 'NONE',  ( 34.81543154690208297, -1.659450418315846276, -5.640188125924651352 ) ) ;
#25259=CARTESIAN_POINT ( 'NONE',  ( 24.45682347496569875, 2.962563052341233405, 3.663525943864573531 ) ) ;
#25260=CARTESIAN_POINT ( 'NONE',  ( 22.01622206693788897, 4.835086392017111656, 3.641232820207879417 ) ) ;
#25263=VERTEX_POINT ( 'NONE', #39613 ) ;
#25264=VERTEX_POINT ( 'NONE', #20888 ) ;
#25270=ORIENTED_EDGE ( 'NONE', *, *, #23425, .T. ) ;
#25273=CARTESIAN_POINT ( 'NONE',  ( 25.30351261480555181, -5.499558619331433640, 2.998554388806299098 ) ) ;
#25276=CARTESIAN_POINT ( 'NONE',  ( 21.83340148893537247, 5.944224929364805732, -3.144417420793418572 ) ) ;
#25282=CARTESIAN_POINT ( 'NONE',  ( -81.77719981938685123, -5.605734774677030963, -1.101378227362841855 ) ) ;
#25283=VECTOR ( 'NONE', #9449, 1000.000000000000000 ) ;
#25286=CARTESIAN_POINT ( 'NONE',  ( 87.73180046618776373, -1.932853647757891258, -3.545598201197500465 ) ) ;
#25290=CARTESIAN_POINT ( 'NONE',  ( 24.95151757009657345, 3.450432584360191512, -1.327079065887385667 ) ) ;
#25293=CARTESIAN_POINT ( 'NONE',  ( 17.06237155660811311, -3.282733088328227744, -2.837945724647277235 ) ) ;
#25297=CARTESIAN_POINT ( 'NONE',  ( 36.97940331721468254, -2.956265398274180889, 5.977928256536974239 ) ) ;
#25299=VECTOR ( 'NONE', #15749, 1000.000000000000000 ) ;
#25300=CARTESIAN_POINT ( 'NONE',  ( 87.34576652878352832, 0.2468139514080059382, -4.863684402402743245 ) ) ;
#25304=CARTESIAN_POINT ( 'NONE',  ( -70.00729340478747531, -45.91674883463290513, 9.958481521799541270 ) ) ;
#25305=DIRECTION ( 'NONE',  ( -5.786005779812646808E-17, 1.000000000000000000, 0.000000000000000000 ) ) ;
#25306=EDGE_CURVE ( 'NONE', #8047, #23544, #30788, .T. ) ;
#25310=ADVANCED_FACE ( 'NONE', ( #36537, #17369 ), #21104, .T. ) ;
#25312=CARTESIAN_POINT ( 'NONE',  ( -75.23198901687325701, -4.970357482903310142, 9.028257795211104053 ) ) ;
#25316=CARTESIAN_POINT ( 'NONE',  ( 35.96230930003272164, -3.155107722808913717, 5.819186136643963891 ) ) ;
#25317=CARTESIAN_POINT ( 'NONE',  ( 23.09208776549577280, 1.724322394091927668, 5.081303647213513131 ) ) ;
#25318=CARTESIAN_POINT ( 'NONE',  ( 37.14829660986974602, -2.504506050704642384, 5.969554084226253998 ) ) ;
#25324=CARTESIAN_POINT ( 'NONE',  ( 85.30708422457949780, 2.536758677189234756, -2.233489723537867011 ) ) ;
#25328=CARTESIAN_POINT ( 'NONE',  ( 23.89361308182833454, 3.044991201845574480, -3.758575451611194662 ) ) ;
#25331=CARTESIAN_POINT ( 'NONE',  ( 21.85643539959778892, -10.77729622265174392, -9.134175241038137827 ) ) ;
#25335=VECTOR ( 'NONE', #26258, 1000.000000000000000 ) ;
#25336=CARTESIAN_POINT ( 'NONE',  ( 86.29974207331044056, 1.340767688666749446, -5.501321414410665689 ) ) ;
#25337=ORIENTED_EDGE ( 'NONE', *, *, #31062, .F. ) ;
#25338=CARTESIAN_POINT ( 'NONE',  ( -81.80090188080514224, -5.603160304130404334, -0.6545554231109831367 ) ) ;
#25339=CARTESIAN_POINT ( 'NONE',  ( 33.10412314342393358, -3.384999426498728425, 5.361320240025687411 ) ) ;
#25340=CARTESIAN_POINT ( 'NONE',  ( 33.68702248893509221, -3.103532886746783070, -5.464072601754253355 ) ) ;
#25344=CARTESIAN_POINT ( 'NONE',  ( 33.45832265597695709, -3.170157842402876014, 5.428378461693221801 ) ) ;
#25346=CARTESIAN_POINT ( 'NONE',  ( 37.17543001156804650, -2.565671956813902810, 5.981153472165249063 ) ) ;
#25352=AXIS2_PLACEMENT_3D ( 'NONE', #39969, #30725, #5388 ) ;
#25354=CARTESIAN_POINT ( 'NONE',  ( -77.15111496589565832, 10.95266906899447434, -7.837837878649032142 ) ) ;
#25360=ORIENTED_EDGE ( 'NONE', *, *, #13429, .F. ) ;
#25361=CARTESIAN_POINT ( 'NONE',  ( 22.66006657518957468, 4.460635658965687256, 3.191315208006852089 ) ) ;
#25370=CARTESIAN_POINT ( 'NONE',  ( 16.22818509040511969, 10.38736679505083416, -2.694565954548105324 ) ) ;
#25379=CARTESIAN_POINT ( 'NONE',  ( 29.08816165369256268, -2.077165169587669613, 5.788842218736271583 ) ) ;
#25385=VECTOR ( 'NONE', #34736, 1000.000000000000000 ) ;
#25389=CARTESIAN_POINT ( 'NONE',  ( 36.17107013121489700, -3.462217916649524607, -5.816204344453734798 ) ) ;
#25392=CARTESIAN_POINT ( 'NONE',  ( 33.96533676093090293, -3.130127305233405099, -5.507510274953758334 ) ) ;
#25394=CARTESIAN_POINT ( 'NONE',  ( -78.80493796903779469, 10.24293490670538986, 7.984127664817240344 ) ) ;
#25395=AXIS2_PLACEMENT_3D ( 'NONE', #38772, #10760, #10567 ) ;
#25407=CARTESIAN_POINT ( 'NONE',  ( 24.15678335194577286, 2.895156585529552906, 3.814851139992612161 ) ) ;
#25416=CARTESIAN_POINT ( 'NONE',  ( 25.29953812343164543, 0.8105978175163669475, 4.611665186302273511 ) ) ;
#25421=VECTOR ( 'NONE', #2717, 1000.000000000000000 ) ;
#25424=CARTESIAN_POINT ( 'NONE',  ( 23.96136931976388951, 3.582231692328178063, -3.646207630380492226 ) ) ;
#25427=CARTESIAN_POINT ( 'NONE',  ( -73.04279461669972306, 7.303834032481013594, 9.776029631287352473 ) ) ;
#25428=CARTESIAN_POINT ( 'NONE',  ( 21.77915531863882848, 0.2033464020057170196, -8.424740673328486196 ) ) ;
#25431=CARTESIAN_POINT ( 'NONE',  ( -80.69318187898312544, 11.48007516437627196, -2.193839972823662166 ) ) ;
#25433=CARTESIAN_POINT ( 'NONE',  ( 36.49343378766320711, -3.559996503287254033, -5.796408034747916993 ) ) ;
#25435=CARTESIAN_POINT ( 'NONE',  ( 20.51617099466335858, 5.905244554751226005, 3.408442687824492445 ) ) ;
#25440=CIRCLE ( 'NONE', #35337, 7.744449365083023729 ) ;
#25442=CARTESIAN_POINT ( 'NONE',  ( 32.10354844262580087, -3.770861253239083055, -4.822966298526184303 ) ) ;
#25444=ORIENTED_EDGE ( 'NONE', *, *, #19262, .T. ) ;
#25452=CARTESIAN_POINT ( 'NONE',  ( 87.41819985312852737, -0.4314763451276128481, -5.556477619079806196 ) ) ;
#25455=CARTESIAN_POINT ( 'NONE',  ( 24.76215755375829275, 2.615058120370138628, 3.935479537194128241 ) ) ;
#25456=CARTESIAN_POINT ( 'NONE',  ( -70.79763891489490391, -21.78299143688767359, 6.000000000000034639 ) ) ;
#25463=DIRECTION ( 'NONE',  ( 1.000000000000000000, 0.000000000000000000, 0.000000000000000000 ) ) ;
#25466=ORIENTED_EDGE ( 'NONE', *, *, #32833, .T. ) ;
#25471=CARTESIAN_POINT ( 'NONE',  ( 1.700390093233090871, -29.56993018339339940, 27.90461065042423527 ) ) ;
#25474=CARTESIAN_POINT ( 'NONE',  ( 22.00805480815993675, 5.522815187245081248, -3.139564157486774754 ) ) ;
#25475=ORIENTED_EDGE ( 'NONE', *, *, #6764, .T. ) ;
#25476=PLANE ( 'NONE',  #34755 ) ;
#25479=CARTESIAN_POINT ( 'NONE',  ( -62.92837670882106238, -23.80776546975053520, -6.000000000000000000 ) ) ;
#25480=CARTESIAN_POINT ( 'NONE',  ( -78.79614016259206721, -5.365327593382188454, -7.951721105412269175 ) ) ;
#25483=CARTESIAN_POINT ( 'NONE',  ( 85.50394501772831291, 1.137698216002840157, 5.721642786829533200 ) ) ;
#25494=CARTESIAN_POINT ( 'NONE',  ( 36.91070730316501169, -2.639519445664956887, 5.967206582125117009 ) ) ;
#25496=CARTESIAN_POINT ( 'NONE',  ( 85.68874278272487288, 2.108061670072472360, -3.902156445801064244 ) ) ;
#25504=DIRECTION ( 'NONE',  ( -1.000000000000000000, -5.421010862427517240E-17, 0.000000000000000000 ) ) ;
#25508=CARTESIAN_POINT ( 'NONE',  ( -73.80648002973117627, -3.552836831368545223, 9.577764321634322897 ) ) ;
#25513=CARTESIAN_POINT ( 'NONE',  ( 24.20720853044049292, 2.174628992932770899, 4.300592713746694606 ) ) ;
#25520=CARTESIAN_POINT ( 'NONE',  ( 14.73500979046645831, 12.83520685450572074, -2.502377855999197820 ) ) ;
#25525=CARTESIAN_POINT ( 'NONE',  ( 23.65416832550485893, 3.201561871976233320, -3.718035610939157465 ) ) ;
#25530=CARTESIAN_POINT ( 'NONE',  ( 21.85643539959781023, -11.34362525346678474, 8.214566034197922306 ) ) ;
#25535=CARTESIAN_POINT ( 'NONE',  ( 87.14327233159831110, 0.3315334873356338141, 5.689878492676547772 ) ) ;
#25536=ORIENTED_EDGE ( 'NONE', *, *, #250, .T. ) ;
#25539=VECTOR ( 'NONE', #20493, 1000.000000000000000 ) ;
#25540=CARTESIAN_POINT ( 'NONE',  ( 14.85966502733631778, -5.942515497032718308, 2.521215392215149009 ) ) ;
#25542=CARTESIAN_POINT ( 'NONE',  ( 33.62812902532535020, -1.230530048054541359, -5.454880852412670400 ) ) ;
#25545=CARTESIAN_POINT ( 'NONE',  ( -73.39219586654201066, -0.5165367281780630648, 10.89398956819519348 ) ) ;
#25549=VERTEX_POINT ( 'NONE', #26224 ) ;
#25551=CARTESIAN_POINT ( 'NONE',  ( 35.21959567110821610, -1.049937720980187672, 5.413415876260859960 ) ) ;
#25556=CYLINDRICAL_SURFACE ( 'NONE', #10759, 12.38600677260393113 ) ;
#25560=ORIENTED_EDGE ( 'NONE', *, *, #6764, .F. ) ;
#25561=CARTESIAN_POINT ( 'NONE',  ( 23.42426635392413914, 3.731876618793696920, 3.231681589700163393 ) ) ;
#25570=CARTESIAN_POINT ( 'NONE',  ( 15.71090316427554967, 10.60011360582976003, -2.658464427050829304 ) ) ;
#25579=CARTESIAN_POINT ( 'NONE',  ( 14.38908526677529842, 8.635444969966599160, 3.482730074327033520 ) ) ;
#25580=CARTESIAN_POINT ( 'NONE',  ( 27.99192205930350497, 2.110044335382625924, -3.171593750069938711 ) ) ;
#25582=DIRECTION ( 'NONE',  ( -1.000000000000000000, 0.000000000000000000, 0.000000000000000000 ) ) ;
#25585=CARTESIAN_POINT ( 'NONE',  ( 14.77222811005485603, -4.461988841550141416, 2.511961482897715481 ) ) ;
#25589=CARTESIAN_POINT ( 'NONE',  ( 25.49148164000159156, 2.250841665744788500, -4.142222679967197507 ) ) ;
#25594=CARTESIAN_POINT ( 'NONE',  ( 22.12509260470467609, -10.94958406946211760, -2.499999999999999556 ) ) ;
#25600=ORIENTED_EDGE ( 'NONE', *, *, #11400, .F. ) ;
#25602=VECTOR ( 'NONE', #1830, 1000.000000000000000 ) ;
#25604=CARTESIAN_POINT ( 'NONE',  ( 24.48230801151231262, 2.778427030854781599, 3.854342034842722420 ) ) ;
#25615=CARTESIAN_POINT ( 'NONE',  ( 22.32644494669605706, 0.2764816045299239300, 7.043421893595684047 ) ) ;
#25624=CARTESIAN_POINT ( 'NONE',  ( 22.71016324673079012, -4.497379315063210647, 7.328459856909534054 ) ) ;
#25627=CARTESIAN_POINT ( 'NONE',  ( -71.87772275130814137, 3.993544671651554800, 9.955241825054214289 ) ) ;
#25628=CARTESIAN_POINT ( 'NONE',  ( 25.40522817991440618, 0.6234987413466189787, -4.602598919802544764 ) ) ;
#25635=CARTESIAN_POINT ( 'NONE',  ( 29.58584611389639463, -3.738994457646588998, -4.503545041254670700 ) ) ;
#25636=CARTESIAN_POINT ( 'NONE',  ( 36.20088530600373389, -3.650368342384689324, -5.718075320652626026 ) ) ;
#25638=CARTESIAN_POINT ( 'NONE',  ( 16.93205111601292856, 9.104991719096041436, 2.849054098494264498 ) ) ;
#25640=LINE ( 'NONE', #38182, #7561 ) ;
#25643=CARTESIAN_POINT ( 'NONE',  ( 23.62990479565404556, 0.6233627752244329523, -5.429377995287568481 ) ) ;
#25644=CARTESIAN_POINT ( 'NONE',  ( 33.57278938729775319, -0.3416013291472669855, -5.045988930500178604 ) ) ;
#25650=CARTESIAN_POINT ( 'NONE',  ( 88.36457133188896762, -1.562442635866588381, -3.606418352999261945 ) ) ;
#25653=CARTESIAN_POINT ( 'NONE',  ( -72.91739463649112452, 3.507283232836214015, -10.95474081624619167 ) ) ;
#25658=VERTEX_POINT ( 'NONE', #29507 ) ;
#25672=CARTESIAN_POINT ( 'NONE',  ( 21.85643539959775694, 4.302923821179891029, -14.48878861646959315 ) ) ;
#25673=CARTESIAN_POINT ( 'NONE',  ( 23.74238088461279972, 3.559840393902792055, -3.189493409904875953 ) ) ;
#25679=CARTESIAN_POINT ( 'NONE',  ( -80.91065676098011750, -6.597313057213480825, -0.5950503846463365276 ) ) ;
#25680=EDGE_CURVE ( 'NONE', #22934, #11656, #13244, .T. ) ;
#25682=DIRECTION ( 'NONE',  ( -0.000000000000000000, -0.000000000000000000, 1.000000000000000000 ) ) ;
#25684=CARTESIAN_POINT ( 'NONE',  ( 86.70396871743868417, -0.5679530053852996918, -5.718564545587779158 ) ) ;
#25685=CARTESIAN_POINT ( 'NONE',  ( 22.06617482514043616, 4.214940469348163354, -2.278054249745394166 ) ) ;
#25687=CARTESIAN_POINT ( 'NONE',  ( 24.90994014085372399, 3.541349694169430684, -0.3428566583711011306 ) ) ;
#25694=CARTESIAN_POINT ( 'NONE',  ( 31.71897322010782005, -0.5584286422544006978, 5.156910915900758674 ) ) ;
#25698=CARTESIAN_POINT ( 'NONE',  ( 86.00040182524281818, 1.757991441285688961, 4.533237565279400805 ) ) ;
#25705=ORIENTED_EDGE ( 'NONE', *, *, #21905, .T. ) ;
#25709=CARTESIAN_POINT ( 'NONE',  ( -76.98048151946119333, -6.014858136247810627, 7.963062423954818669 ) ) ;
#25715=CARTESIAN_POINT ( 'NONE',  ( 22.53613453900640451, 1.693789802652694521, 5.566700593757581750 ) ) ;
#25722=CARTESIAN_POINT ( 'NONE',  ( 85.33631068939730824, 2.503930124734163432, 2.279864513413099925 ) ) ;
#25726=CARTESIAN_POINT ( 'NONE',  ( 22.41273418899857361, 3.677808312967091098, -4.075635063406390479 ) ) ;
#25729=CARTESIAN_POINT ( 'NONE',  ( 21.85643539959777826, -11.73360331217645225, -7.400322805736739618 ) ) ;
#25730=CARTESIAN_POINT ( 'NONE',  ( 21.20506779834672884, 9.695729361094967302, 1.510497956681738305E-12 ) ) ;
#25731=ORIENTED_EDGE ( 'NONE', *, *, #22573, .T. ) ;
#25734=CARTESIAN_POINT ( 'NONE',  ( 85.96608680028057847, 1.729603650198207054, 5.123763289084741324 ) ) ;
#25735=EDGE_CURVE ( 'NONE', #18355, #18960, #23717, .T. ) ;
#25739=CARTESIAN_POINT ( 'NONE',  ( 14.74798687898900162, -4.496105769315120959, 2.508178052513492684 ) ) ;
#25740=CARTESIAN_POINT ( 'NONE',  ( 36.39182469969075839, -2.321310407235841033, 5.886222402629798900 ) ) ;
#25742=CARTESIAN_POINT ( 'NONE',  ( 21.25554376393856160, 3.326128914239820489, -3.523839690267918545 ) ) ;
#25746=CARTESIAN_POINT ( 'NONE',  ( -73.02027574113616026, 0.7163629790712561229, 10.94380017644704495 ) ) ;
#25753=ORIENTED_EDGE ( 'NONE', *, *, #28742, .T. ) ;
#25754=CARTESIAN_POINT ( 'NONE',  ( 35.72916689304948790, -1.306553130388697470, 5.539900376742572519 ) ) ;
#25755=CARTESIAN_POINT ( 'NONE',  ( 11.29080664838498826, -10.90558813203967148, 6.000000000000000000 ) ) ;
#25761=FACE_OUTER_BOUND ( 'NONE', #27056, .T. ) ;
#25763=CARTESIAN_POINT ( 'NONE',  ( -70.92837670882107659, -23.80776546975053520, 0.000000000000000000 ) ) ;
#25775=CARTESIAN_POINT ( 'NONE',  ( 14.77413646174418993, 12.29989388524484717, -2.512259327332496461 ) ) ;
#25780=AXIS2_PLACEMENT_3D ( 'NONE', #31096, #31703, #12545 ) ;
#25785=CARTESIAN_POINT ( 'NONE',  ( 13.68084590952481427, 8.951769248947412549, 3.481680054008543745 ) ) ;
#25786=CARTESIAN_POINT ( 'NONE',  ( 27.46505532721044318, 0.1961140298417080874, 5.884446595982424810 ) ) ;
#25788=CARTESIAN_POINT ( 'NONE',  ( -80.92837670882107659, 2.429809908903242555, 12.50000000000000000 ) ) ;
#25792=DIRECTION ( 'NONE',  ( -1.000000000000000000, 0.000000000000000000, 0.000000000000000000 ) ) ;
#25793=CARTESIAN_POINT ( 'NONE',  ( 37.05407933310225133, -3.059547152614165544, -5.984220936588256379 ) ) ;
#25797=CARTESIAN_POINT ( 'NONE',  ( -80.23765913646487036, 10.48825455491124536, 6.049483936935463824 ) ) ;
#25798=LINE ( 'NONE', #4186, #30716 ) ;
#25806=CARTESIAN_POINT ( 'NONE',  ( 24.12107463544779407, 2.969626750525581560, 3.756100707807366046 ) ) ;
#25822=CARTESIAN_POINT ( 'NONE',  ( 22.30986545779548536, 0.2685651372915308088, 7.076871089830634176 ) ) ;
#25826=DIRECTION ( 'NONE',  ( 0.000000000000000000, -1.000000000000000000, 0.000000000000000000 ) ) ;
#25830=CARTESIAN_POINT ( 'NONE',  ( 24.19350110911862828, 1.223952504169800948, -6.554579921768042716 ) ) ;
#25834=CARTESIAN_POINT ( 'NONE',  ( -77.85578999393689514, -5.090959542573109786, 7.225404102923549843 ) ) ;
#25835=CARTESIAN_POINT ( 'NONE',  ( 24.74194048200748597, 0.5346423267196033224, -4.782325428828064773 ) ) ;
#25837=ORIENTED_EDGE ( 'NONE', *, *, #12119, .T. ) ;
#25838=CARTESIAN_POINT ( 'NONE',  ( 24.15143939495542469, 3.654138348660112445, 2.050033071069497392 ) ) ;
#25839=CARTESIAN_POINT ( 'NONE',  ( 25.73330770164922043, 2.636588466549696808, -3.521397845908182944 ) ) ;
#25842=CARTESIAN_POINT ( 'NONE',  ( 19.21638140921048432, 7.328436742462230313, 3.172542048904986256 ) ) ;
#25848=CARTESIAN_POINT ( 'NONE',  ( 22.45284782988909811, 0.4695142227150546077, -6.716274792382588288 ) ) ;
#25849=CARTESIAN_POINT ( 'NONE',  ( 35.79905751890628096, -1.348410822439406020, -5.558858606210413278 ) ) ;
#25850=CARTESIAN_POINT ( 'NONE',  ( 14.77222812468949620, -65.19654454972992141, 2.511961485181804843 ) ) ;
#25853=ORIENTED_EDGE ( 'NONE', *, *, #15939, .F. ) ;
#25855=CARTESIAN_POINT ( 'NONE',  ( 87.21044761576042958, -0.9232309944945271685, 5.337239039084527015 ) ) ;
#25856=ORIENTED_EDGE ( 'NONE', *, *, #20772, .T. ) ;
#25857=CARTESIAN_POINT ( 'NONE',  ( -73.02118209071689137, 4.148434801556117435, -10.94370216587312328 ) ) ;
#25876=CARTESIAN_POINT ( 'NONE',  ( 23.14179022917130624, 4.013511596053603192, -3.137277550560443995 ) ) ;
#25882=CARTESIAN_POINT ( 'NONE',  ( -73.70917786874233002, -1.221531673705063215, -10.83923324353724382 ) ) ;
#25884=CARTESIAN_POINT ( 'NONE',  ( -70.92837670882238399, -21.78299143689875095, 10.00000000000113154 ) ) ;
#25886=CARTESIAN_POINT ( 'NONE',  ( 84.54687988124997844, 2.467165036067117789, -3.672804150685311964 ) ) ;
#25894=CARTESIAN_POINT ( 'NONE',  ( 18.54755872719595544, 7.518511093671114587, -3.101193132418598175 ) ) ;
#25899=CARTESIAN_POINT ( 'NONE',  ( 31.71961843867553199, -0.5565345743523945066, 5.157011617862919728 ) ) ;
#25902=CARTESIAN_POINT ( 'NONE',  ( 88.28392341775159480, -0.8069683938931414557, -2.555979571574120257 ) ) ;
#25915=EDGE_CURVE ( 'NONE', #21520, #24796, #18761, .T. ) ;
#25918=CARTESIAN_POINT ( 'NONE',  ( 24.13837906798738686, 1.684127973681580848, 4.584305409718924196 ) ) ;
#25919=ORIENTED_EDGE ( 'NONE', *, *, #32226, .F. ) ;
#25922=AXIS2_PLACEMENT_3D ( 'NONE', #23123, #16523, #29099 ) ;
#25926=CARTESIAN_POINT ( 'NONE',  ( 85.63625186893746388, 2.167021955807470590, 3.489522741179289067 ) ) ;
#25929=CARTESIAN_POINT ( 'NONE',  ( 22.77263692411995066, 3.805474047185834596, -3.697090138710067198 ) ) ;
#25933=EDGE_CURVE ( 'NONE', #5343, #25658, #12172, .T. ) ;
#25934=CARTESIAN_POINT ( 'NONE',  ( 21.85643539959774273, 10.54442680926682208, -0.8960936389291185300 ) ) ;
#25935=CARTESIAN_POINT ( 'NONE',  ( 21.77466435201619888, 5.668278662187346661, -2.100676170762209249 ) ) ;
#25938=CARTESIAN_POINT ( 'NONE',  ( 88.61980888719223515, -1.376070350315937940, 2.940712392697649058 ) ) ;
#25945=CARTESIAN_POINT ( 'NONE',  ( 32.39520944364767274, -3.784153674530718714, 4.877599362950213013 ) ) ;
#25946=CARTESIAN_POINT ( 'NONE',  ( 36.78920673448757128, -3.041418453456746551, -5.948243479880678919 ) ) ;
#25956=CARTESIAN_POINT ( 'NONE',  ( 33.44054677433027933, -3.435571797939218186, 5.408185224205094954 ) ) ;
#25959=CARTESIAN_POINT ( 'NONE',  ( 34.79243474202561970, -3.834671068451598330, 5.377539100044668174 ) ) ;
#25962=CARTESIAN_POINT ( 'NONE',  ( 87.79841724921489288, -2.358232370636156094, -2.005059250078357724 ) ) ;
#25964=DIRECTION ( 'NONE',  ( 0.000000000000000000, 0.000000000000000000, -1.000000000000000000 ) ) ;
#25970=CARTESIAN_POINT ( 'NONE',  ( 22.91573592208010623, 4.163909958596558880, 3.247526573974286013 ) ) ;
#25978=DIRECTION ( 'NONE',  ( -0.000000000000000000, -0.000000000000000000, -1.000000000000000000 ) ) ;
#25981=ORIENTED_EDGE ( 'NONE', *, *, #27979, .F. ) ;
#25982=LINE ( 'NONE', #16298, #33337 ) ;
#25985=CARTESIAN_POINT ( 'NONE',  ( 25.94849358905778658, 1.816623773615693160, -4.256288009898165470 ) ) ;
#25988=CARTESIAN_POINT ( 'NONE',  ( 29.14988983353436680, -2.161137664473038900, -5.740130334263455758 ) ) ;
#25990=CARTESIAN_POINT ( 'NONE',  ( 30.13156937888698650, -4.637989059070824815, 0.4506576151153146581 ) ) ;
#25996=CARTESIAN_POINT ( 'NONE',  ( 36.88189763748390959, -2.428839298856057205, -5.959479764620102316 ) ) ;
#26002=CARTESIAN_POINT ( 'NONE',  ( 21.86476427169857217, -13.72881702355425659, -2.499999999999999556 ) ) ;
#26003=VECTOR ( 'NONE', #27752, 1000.000000000000000 ) ;
#26006=CYLINDRICAL_SURFACE ( 'NONE', #21423, 12.73502530973474123 ) ;
#26008=CARTESIAN_POINT ( 'NONE',  ( 36.73497401824715780, -2.304546233985284687, 5.935212642074513489 ) ) ;
#26015=CARTESIAN_POINT ( 'NONE',  ( 30.71442180045753290, -3.288768831658976932, 4.965733434219046671 ) ) ;
#26016=CARTESIAN_POINT ( 'NONE',  ( 23.47630927499801246, 3.090003628763607679, 3.883072686897193648 ) ) ;
#26021=CARTESIAN_POINT ( 'NONE',  ( 22.38222497467343430, 4.936969384760538482, 3.050972054430843183 ) ) ;
#26026=CARTESIAN_POINT ( 'NONE',  ( 26.75149414979017237, 0.8971556662521585901, 4.382797809037470849 ) ) ;
#26036=CARTESIAN_POINT ( 'NONE',  ( 22.82080504511013430, -6.970192185297126031, -1.116939615399285657 ) ) ;
#26039=CARTESIAN_POINT ( 'NONE',  ( -80.77097820227440650, -5.650553507305215994, 4.970441783940528602 ) ) ;
#26040=CARTESIAN_POINT ( 'NONE',  ( 26.76517688821456886, 0.8539537780654303800, -4.383552559536760818 ) ) ;
#26042=CIRCLE ( 'NONE', #25395, 1.000000000000005107 ) ;
#26047=CARTESIAN_POINT ( 'NONE',  ( 36.49309394506007465, -3.558324574553789699, -5.797191926096202153 ) ) ;
#26052=LINE ( 'NONE', #32241, #25335 ) ;
#26056=CARTESIAN_POINT ( 'NONE',  ( 22.80317954561651561, 0.6168027127662122355, -6.115043150466682675 ) ) ;
#26057=CARTESIAN_POINT ( 'NONE',  ( 32.98075398114073664, -0.1054326221632065214, -4.920934273367439715 ) ) ;
#26059=CARTESIAN_POINT ( 'NONE',  ( 19.45444762198869881, 11.13896630807285781, -2.499999999999990230 ) ) ;
#26063=CARTESIAN_POINT ( 'NONE',  ( 84.10435792013542766, 3.012680099502687892, -0.4953216543819284889 ) ) ;
#26065=ORIENTED_EDGE ( 'NONE', *, *, #37090, .T. ) ;
#26066=CARTESIAN_POINT ( 'NONE',  ( -8.295002936191391285, 28.24537450226321411, 2.500000000000000000 ) ) ;
#26068=VECTOR ( 'NONE', #16206, 1000.000000000000000 ) ;
#26070=CARTESIAN_POINT ( 'NONE',  ( -61.24591834330252027, 10.37661300689600097, -2.500000000000000000 ) ) ;
#26071=ORIENTED_EDGE ( 'NONE', *, *, #28738, .T. ) ;
#26079=CARTESIAN_POINT ( 'NONE',  ( 24.20923528093676680, 2.663529708714821087, 3.984834686794740399 ) ) ;
#26082=CARTESIAN_POINT ( 'NONE',  ( 21.85643539959776049, -3.688311691778667800, 15.92486026856874304 ) ) ;
#26084=CARTESIAN_POINT ( 'NONE',  ( 24.06794754132348046, 3.349686124075685445, -3.202891862519920529 ) ) ;
#26089=LINE ( 'NONE', #38824, #28078 ) ;
#26091=CARTESIAN_POINT ( 'NONE',  ( -72.95563224246589584, 3.799282472582091508, -9.852485720729166729 ) ) ;
#26092=DIRECTION ( 'NONE',  ( -0.000000000000000000, -0.000000000000000000, -1.000000000000000000 ) ) ;
#26093=CYLINDRICAL_SURFACE ( 'NONE', #16872, 3.000000000000002665 ) ;
#26095=CARTESIAN_POINT ( 'NONE',  ( 86.27652758060003180, -0.2533697966053802819, -5.917929974479952726 ) ) ;
#26100=AXIS2_PLACEMENT_3D ( 'NONE', #7676, #11151, #13658 ) ;
#26101=VECTOR ( 'NONE', #28307, 1000.000000000000000 ) ;
#26107=EDGE_CURVE ( 'NONE', #14959, #25549, #19382, .T. ) ;
#26110=CARTESIAN_POINT ( 'NONE',  ( 35.78611850173684417, -3.163414878908757277, 5.791687301379355723 ) ) ;
#26112=CARTESIAN_POINT ( 'NONE',  ( 87.14484084030976874, 0.3304612005822565313, -5.669005978848654870 ) ) ;
#26127=CARTESIAN_POINT ( 'NONE',  ( 23.86924164457367681, 1.381515540322357793, 4.867119774624979023 ) ) ;
#26132=CARTESIAN_POINT ( 'NONE',  ( 86.45266110354762645, 1.249992354373530290, 4.889332228698039629 ) ) ;
#26135=CARTESIAN_POINT ( 'NONE',  ( 23.66861057507165356, 3.139937292340087893, -3.766843508339346780 ) ) ;
#26140=CARTESIAN_POINT ( 'NONE',  ( 21.85643539959774273, 10.58808081918846256, 0.01331417752983106093 ) ) ;
#26141=CARTESIAN_POINT ( 'NONE',  ( 21.38787910473958220, 9.379444465846978218, 3.308503362033488049 ) ) ;
#26144=CARTESIAN_POINT ( 'NONE',  ( 87.00363285854439255, 0.09201467311058098009, -5.867932143725643535 ) ) ;
#26147=CARTESIAN_POINT ( 'NONE',  ( -80.83812573300635052, -5.651420041020555729, 4.817690839865847785 ) ) ;
#26148=CARTESIAN_POINT ( 'NONE',  ( 19.69258716046599744, -2.691695111070238955, 3.279902512047694341 ) ) ;
#26150=DIRECTION ( 'NONE',  ( 0.000000000000000000, -0.000000000000000000, -1.000000000000000000 ) ) ;
#26151=CARTESIAN_POINT ( 'NONE',  ( 14.85065079210121652, -6.130908026932606170, -2.524201239090782867 ) ) ;
#26153=CARTESIAN_POINT ( 'NONE',  ( 36.97934183402728792, -2.956306430206838254, -5.977918660598608547 ) ) ;
#26156=CARTESIAN_POINT ( 'NONE',  ( 29.83052353176027793, -3.763946442397907877, -4.488211747472833579 ) ) ;
#26158=VECTOR ( 'NONE', #18350, 1000.000000000000000 ) ;
#26159=( GEOMETRIC_REPRESENTATION_CONTEXT ( 3 ) GLOBAL_UNCERTAINTY_ASSIGNED_CONTEXT ( ( #37794 ) ) GLOBAL_UNIT_ASSIGNED_CONTEXT ( ( #6529, #10201, #35352 ) ) REPRESENTATION_CONTEXT ( 'NONE', 'WORKASPACE' ) );
#26164=CARTESIAN_POINT ( 'NONE',  ( 37.17655189852746389, -2.564752334915549437, 5.980995930358914414 ) ) ;
#26167=CARTESIAN_POINT ( 'NONE',  ( 87.91634809178921728, -2.499602875977831484, 0.5197879843876231920 ) ) ;
#26174=ORIENTED_EDGE ( 'NONE', *, *, #8902, .T. ) ;
#26175=CARTESIAN_POINT ( 'NONE',  ( 22.11225299742777750, 4.986280216054901793, 3.411143437232363240 ) ) ;
#26194=CARTESIAN_POINT ( 'NONE',  ( 86.50262394474026451, 1.193871719766480100, -4.934721793127618383 ) ) ;
#26195=CARTESIAN_POINT ( 'NONE',  ( 28.10280119166142399, -0.8120181649793116740, 6.074162340139093175 ) ) ;
#26203=EDGE_CURVE ( 'NONE', #19840, #1813, #33187, .T. ) ;
#26204=CARTESIAN_POINT ( 'NONE',  ( 33.82080240299477225, -0.7236866431670748723, -5.383600818459516546 ) ) ;
#26209=DIRECTION ( 'NONE',  ( 0.000000000000000000, 1.000000000000000000, 0.000000000000000000 ) ) ;
#26210=DIRECTION ( 'NONE',  ( -0.000000000000000000, -0.000000000000000000, -1.000000000000000000 ) ) ;
#26213=CARTESIAN_POINT ( 'NONE',  ( 33.43765011243894492, -3.587404715383258669, 5.336366798597405037 ) ) ;
#26220=CARTESIAN_POINT ( 'NONE',  ( 30.78887672857765168, -3.335710177092375162, 4.962067852009124813 ) ) ;
#26221=CARTESIAN_POINT ( 'NONE',  ( 85.89661503870057402, 0.4533383911654620402, -5.989758072366164754 ) ) ;
#26224=CARTESIAN_POINT ( 'NONE',  ( 8.290806648384990041, -25.50263309590217276, 6.000000000000001776 ) ) ;
#26226=CARTESIAN_POINT ( 'NONE',  ( 21.98943303986548514, 5.609607562178218210, 3.094355746606469726 ) ) ;
#26233=CARTESIAN_POINT ( 'NONE',  ( 23.59121300012005307, 0.4241677973105192345, 5.524108833373179372 ) ) ;
#26241=CARTESIAN_POINT ( 'NONE',  ( 11.29080664838498826, -10.90558813203967148, 6.000000000000000000 ) ) ;
#26242=ORIENTED_EDGE ( 'NONE', *, *, #7348, .T. ) ;
#26244=CARTESIAN_POINT ( 'NONE',  ( 22.35506120569036170, 4.170988562608182626, 6.826273348963533216 ) ) ;
#26246=ORIENTED_EDGE ( 'NONE', *, *, #30094, .F. ) ;
#26247=CARTESIAN_POINT ( 'NONE',  ( -78.23674730379569553, -6.442058846907860570, 6.837204711868661633 ) ) ;
#26252=CARTESIAN_POINT ( 'NONE',  ( 35.22080398260825262, -1.047803307765222902, -5.411327744522335337 ) ) ;
#26254=CARTESIAN_POINT ( 'NONE',  ( -4.444218661349752963, -35.94265729135299381, -2.500000000000000000 ) ) ;
#26258=DIRECTION ( 'NONE',  ( -0.000000000000000000, -0.000000000000000000, -1.000000000000000000 ) ) ;
#26265=CARTESIAN_POINT ( 'NONE',  ( 84.13636243568421946, 2.973867306686137191, 1.134085816324387430 ) ) ;
#26274=DIRECTION ( 'NONE',  ( 0.000000000000000000, 1.000000000000000000, 0.000000000000000000 ) ) ;
#26279=CARTESIAN_POINT ( 'NONE',  ( 33.78683981622189947, -4.850133216411556702, 3.460854720750057290 ) ) ;
#26281=CARTESIAN_POINT ( 'NONE',  ( -12.99139449055068241, -10.90558813203967148, 2.500000000000000000 ) ) ;
#26283=CARTESIAN_POINT ( 'NONE',  ( 25.78209274739939971, 1.896337777400309399, 4.230317134137809632 ) ) ;
#26286=CARTESIAN_POINT ( 'NONE',  ( 21.85643539959777470, -5.967561930184303698, -15.30482168765389694 ) ) ;
#26291=CARTESIAN_POINT ( 'NONE',  ( 14.66134950408317472, -4.888884664723367024, -2.500000000000003553 ) ) ;
#26293=CARTESIAN_POINT ( 'NONE',  ( -74.81248793487165472, -2.854500793830079264, -10.54724492771533839 ) ) ;
#26295=CARTESIAN_POINT ( 'NONE',  ( -70.92837670882107659, -65.19654454972992141, 0.000000000000000000 ) ) ;
#26308=CARTESIAN_POINT ( 'NONE',  ( 25.29826323614737404, 1.741216666318694317, 4.154803837446060299 ) ) ;
#26310=CARTESIAN_POINT ( 'NONE',  ( 85.25019696446999262, 2.600657147776545663, -2.704904232406868836 ) ) ;
#26325=CARTESIAN_POINT ( 'NONE',  ( 24.59373887808777681, 0.8454200395481480390, 4.793554178231363316 ) ) ;
#26333=CARTESIAN_POINT ( 'NONE',  ( 8.290806648384990041, -25.50263309590217276, 2.499999999999998668 ) ) ;
#26335=B_SPLINE_SURFACE_WITH_KNOTS ( 'NONE', 3, 3, ( 
 ( #28801, #34591, #6159, #9027 ),
 ( #12525, #22016, #25099, #6021 ),
 ( #40582, #34447, #15685, #9500 ),
 ( #18987, #31965, #37498, #12797 ),
 ( #3374, #13006, #16293, #25775 ),
 ( #19187, #18772, #31346, #18558 ),
 ( #257, #28449, #25160, #31143 ),
 ( #15688, #22293, #28661, #28039 ),
 ( #3767, #13207, #15890, #35262 ),
 ( #22086, #38312, #24964, #25570 ),
 ( #25370, #28863, #37908, #31753 ),
 ( #9714, #21873, #22697, #10109 ),
 ( #34864, #19391, #28239, #35061 ),
 ( #2961, #3173, #9917, #6432 ),
 ( #6640, #64, #3565, #34660 ),
 ( #9295, #15477, #670, #40586 ),
 ( #12396, #34450, #6227, #12593 ),
 ( #37695, #9503, #18990, #16095 ),
 ( #31551, #467, #22498, #38114 ),
 ( #6835, #11109, #26781, #35855 ),
 ( #7833, #16680, #23488, #7428 ),
 ( #39116, #35658, #20383, #1278 ) ),
 .UNSPECIFIED., .F., .F., .F.,
 ( 4, 3, 3, 3, 3, 3, 3, 4 ),
 ( 4, 4 ),
 ( 0.004706533420950041041, 0.005436807504379657062, 0.006167081587809273083, 0.007627629754668505992, 0.009088177921527738901, 0.01054872608838697094, 0.01346982242210543676, 0.01639091875582390084 ),
 ( -0.006049311920859260297, 1.000000000000000000 ),
 .UNSPECIFIED. ) ;
#26339=CARTESIAN_POINT ( 'NONE',  ( 23.16337524629349076, 3.871609807089642530, -3.315521066308895204 ) ) ;
#26342=CARTESIAN_POINT ( 'NONE',  ( 23.96136931976388951, 3.582231692328178063, -3.646207630380492226 ) ) ;
#26344=CARTESIAN_POINT ( 'NONE',  ( 21.46948114135329533, 9.243557392227998548, 3.873122283670993315 ) ) ;
#26347=CARTESIAN_POINT ( 'NONE',  ( 88.14352194013933683, -1.303227188646099544, -4.271130342077624320 ) ) ;
#26352=CARTESIAN_POINT ( 'NONE',  ( 32.25525712155970837, -3.777699995816486744, 4.851130129795467205 ) ) ;
#26353=CARTESIAN_POINT ( 'NONE',  ( 28.89950236053841692, -2.887785649367553553, -4.716864299104555514 ) ) ;
#26354=CARTESIAN_POINT ( 'NONE',  ( 31.71837165913483148, -0.5603379253444896735, -5.156817027762116368 ) ) ;
#26357=CARTESIAN_POINT ( 'NONE',  ( 30.28289254991746304, -3.677685065117360264, -4.636463722753257244 ) ) ;
#26358=ORIENTED_EDGE ( 'NONE', *, *, #10627, .T. ) ;
#26364=CARTESIAN_POINT ( 'NONE',  ( 36.71923328895664440, -3.458898378518612038, 5.860548135656104662 ) ) ;
#26365=CARTESIAN_POINT ( 'NONE',  ( -58.92473026143643722, -52.43948302755219260, 2.500000000000000000 ) ) ;
#26367=CARTESIAN_POINT ( 'NONE',  ( 86.41034863701202084, -0.4798547535092105298, 5.807516434511641457 ) ) ;
#26368=ORIENTED_EDGE ( 'NONE', *, *, #38211, .T. ) ;
#26376=EDGE_LOOP ( 'NONE', ( #12584, #40428, #11945, #24051, #31653, #17340 ) ) ;
#26377=CARTESIAN_POINT ( 'NONE',  ( 21.78882382717254274, 5.524186801048877271, 3.510389251737664473 ) ) ;
#26379=FACE_OUTER_BOUND ( 'NONE', #1409, .T. ) ;
#26381=ORIENTED_EDGE ( 'NONE', *, *, #38211, .F. ) ;
#26383=CARTESIAN_POINT ( 'NONE',  ( 33.46455515056310759, -3.089188617792877789, 5.429351193206847448 ) ) ;
#26387=CARTESIAN_POINT ( 'NONE',  ( 24.55753766420681217, 2.522355539012570702, -4.006862819802994302 ) ) ;
#26389=AXIS2_PLACEMENT_3D ( 'NONE', #24837, #17453, #27911 ) ;
#26391=CARTESIAN_POINT ( 'NONE',  ( 24.75065437802840052, 2.392517948343078960, -4.069336231166236217 ) ) ;
#26396=CARTESIAN_POINT ( 'NONE',  ( 33.86666996155606313, -5.260714354287511441, -2.203027216165969637 ) ) ;
#26403=CARTESIAN_POINT ( 'NONE',  ( 35.47955784773917998, -1.848538386244011900, -5.743841097125561568 ) ) ;
#26411=CARTESIAN_POINT ( 'NONE',  ( 36.17116650710612902, -3.462198426845603638, 5.816222086175844019 ) ) ;
#26419=CARTESIAN_POINT ( 'NONE',  ( 85.37673136558751708, 1.331923910713227466, -5.551005466948024214 ) ) ;
#26424=CARTESIAN_POINT ( 'NONE',  ( 24.38923258654877202, 3.155769846838503589, 3.307240130081302798 ) ) ;
#26428=CARTESIAN_POINT ( 'NONE',  ( 26.00772565174600359, -2.423984237576000123, -4.803821987795020121 ) ) ;
#26432=CARTESIAN_POINT ( 'NONE',  ( 22.29628800937758015, 0.2617764422785469614, 7.104517024768484568 ) ) ;
#26440=CARTESIAN_POINT ( 'NONE',  ( 28.70293208761703241, -1.592347763559425200, -5.966126087555218227 ) ) ;
#26443=CARTESIAN_POINT ( 'NONE',  ( -78.50546482259380809, -6.500811299971071655, 6.538465153154030318 ) ) ;
#26444=CARTESIAN_POINT ( 'NONE',  ( 22.61749032200219034, 0.2966866550508970302, -6.491723916333954847 ) ) ;
#26448=CARTESIAN_POINT ( 'NONE',  ( 34.63659524554710600, -0.7829862400395763977, -5.276330072109475466 ) ) ;
#26449=CARTESIAN_POINT ( 'NONE',  ( 1.700390093233090871, -29.56993018339339940, -6.000000000000000000 ) ) ;
#26463=CARTESIAN_POINT ( 'NONE',  ( 84.65562454054800412, 2.508334066475362167, -3.654169056841765517 ) ) ;
#26464=CARTESIAN_POINT ( 'NONE',  ( -80.04662500899941335, 10.46548227099173900, -6.327377141109288061 ) ) ;
#26474=CARTESIAN_POINT ( 'NONE',  ( 33.53294034083837261, -4.003968611202963324, 4.914558353369265831 ) ) ;
#26478=FACE_OUTER_BOUND ( 'NONE', #40560, .T. ) ;
#26481=CARTESIAN_POINT ( 'NONE',  ( 21.85643539959780313, -9.021070270546461600, 11.21731785579436291 ) ) ;
#26482=CARTESIAN_POINT ( 'NONE',  ( 22.38220106028803613, 4.937111810673596501, -3.050830205725867383 ) ) ;
#26488=FACE_OUTER_BOUND ( 'NONE', #28175, .T. ) ;
#26489=CARTESIAN_POINT ( 'NONE',  ( -75.35807269576923773, -3.444886077232420796, -9.005146983506810088 ) ) ;
#26491=CYLINDRICAL_SURFACE ( 'NONE', #3087, 6.000000000000002665 ) ;
#26497=EDGE_CURVE ( 'NONE', #26946, #16350, #32435, .T. ) ;
#26503=CARTESIAN_POINT ( 'NONE',  ( 36.78928159892215177, -3.041397198625128695, 5.948255164286288199 ) ) ;
#26507=CARTESIAN_POINT ( 'NONE',  ( 87.15505355144220800, 0.4610318193416703680, -5.246243280819175681 ) ) ;
#26513=CARTESIAN_POINT ( 'NONE',  ( -76.51582565984999462, 10.65402114766428987, -8.295614104186167737 ) ) ;
#26520=CARTESIAN_POINT ( 'NONE',  ( 23.62669510910421167, 0.5457874777667105493, 5.460871266645791700 ) ) ;
#26521=ORIENTED_EDGE ( 'NONE', *, *, #33518, .T. ) ;
#26522=AXIS2_PLACEMENT_3D ( 'NONE', #31881, #34984, #12719 ) ;
#26524=CARTESIAN_POINT ( 'NONE',  ( 14.69558838330753936, 10.99631180437154399, -6.000000000000000888 ) ) ;
#26529=CARTESIAN_POINT ( 'NONE',  ( 21.76138600010604307, 5.847767184895531933, -3.374880873801382020 ) ) ;
#26533=CARTESIAN_POINT ( 'NONE',  ( 21.85643539959775694, 4.180186707270823199, 11.06385087694989799 ) ) ;
#26534=CARTESIAN_POINT ( 'NONE',  ( 21.26333942294113655, 9.593021065649088186, -2.042309770458127893 ) ) ;
#26535=CARTESIAN_POINT ( 'NONE',  ( 15.67275371359048997, 8.062146741059187605, 3.484635839389762069 ) ) ;
#26538=CARTESIAN_POINT ( 'NONE',  ( 87.00256539079671825, 0.09090593131677454641, 5.889906316148251442 ) ) ;
#26541=CARTESIAN_POINT ( 'NONE',  ( -76.83900407126830601, -4.548844688613328024, 9.590346143861395944 ) ) ;
#26542=CARTESIAN_POINT ( 'NONE',  ( 18.24134202378618497, -2.850333121144178694, 3.053400609972546587 ) ) ;
#26544=CARTESIAN_POINT ( 'NONE',  ( 14.73497390326914491, -4.430518890905947416, -2.506147062932408520 ) ) ;
#26545=CARTESIAN_POINT ( 'NONE',  ( 30.51508027424239700, -0.1407365609915100790, -4.969014305437574386 ) ) ;
#26547=CARTESIAN_POINT ( 'NONE',  ( 85.36230419630793165, 1.362237581505277406, 5.546959353559891781 ) ) ;
#26549=EDGE_LOOP ( 'NONE', ( #21389, #10690, #40466, #37359 ) ) ;
#26553=VECTOR ( 'NONE', #9222, 1000.000000000000000 ) ;
#26558=CARTESIAN_POINT ( 'NONE',  ( 33.94626592564545575, -0.4876026740605987619, 5.120945191898142568 ) ) ;
#26561=CARTESIAN_POINT ( 'NONE',  ( 87.85437433257010298, -2.425468598688185207, 1.529927975848801136 ) ) ;
#26562=AXIS2_PLACEMENT_3D ( 'NONE', #13094, #12273, #22382 ) ;
#26564=VERTEX_POINT ( 'NONE', #30777 ) ;
#26568=CARTESIAN_POINT ( 'NONE',  ( 21.91948103535845505, 3.888016741293982115, 2.591533416524685960E-12 ) ) ;
#26570=CARTESIAN_POINT ( 'NONE',  ( 24.20056197448974089, 3.097996102763779902, 3.573029051228984621 ) ) ;
#26575=CARTESIAN_POINT ( 'NONE',  ( 14.89512109076932944, -4.197941490224893712, -2.531141904716178725 ) ) ;
#26578=CARTESIAN_POINT ( 'NONE',  ( 22.26754414936907267, 2.303131529692775459, -5.275206787684171950 ) ) ;
#26580=AXIS2_PLACEMENT_3D ( 'NONE', #11951, #27207, #14438 ) ;
#26582=DIRECTION ( 'NONE',  ( 1.000000000000000000, 7.232507224765808510E-18, 0.000000000000000000 ) ) ;
#26587=CARTESIAN_POINT ( 'NONE',  ( 86.00040182524281818, 1.757991441285688961, 4.533237565279400805 ) ) ;
#26588=CARTESIAN_POINT ( 'NONE',  ( 32.62845853548997610, -2.537451394787784142, 5.899574533259067444 ) ) ;
#26590=CARTESIAN_POINT ( 'NONE',  ( -72.12105268511338352, -46.20207945875944944, 9.928773179615475897 ) ) ;
#26592=CARTESIAN_POINT ( 'NONE',  ( -77.95630793809591808, -5.091041188919200877, -8.764182688739834859 ) ) ;
#26596=CARTESIAN_POINT ( 'NONE',  ( 35.33516124645243650, -3.300847515999512094, -5.721304515250182909 ) ) ;
#26600=ADVANCED_FACE ( 'NONE', ( #22118, #2998 ), #14895, .T. ) ;
#26605=CARTESIAN_POINT ( 'NONE',  ( 31.93464789591948261, 0.01672602609938712154, 5.060956730290721239 ) ) ;
#26615=CARTESIAN_POINT ( 'NONE',  ( 85.95116560976015307, 0.3509943572283380497, -5.999998676670047715 ) ) ;
#26620=CARTESIAN_POINT ( 'NONE',  ( 22.61872426168702077, 4.601640665309255418, 3.069969487110096207 ) ) ;
#26627=CARTESIAN_POINT ( 'NONE',  ( 24.73536326808030950, 0.6125365926123585991, 4.779974774574727192 ) ) ;
#26638=CARTESIAN_POINT ( 'NONE',  ( 24.33259761278756272, 0.1721304915443387373, 6.926443425830641765 ) ) ;
#26640=ORIENTED_EDGE ( 'NONE', *, *, #13331, .T. ) ;
#26641=CARTESIAN_POINT ( 'NONE',  ( -80.93415443611787907, -6.594512348378300359, 0.2227253658375672740 ) ) ;
#26642=CARTESIAN_POINT ( 'NONE',  ( 26.04620955633046009, 0.8112080387504423395, -4.422430910127713055 ) ) ;
#26646=CIRCLE ( 'NONE', #38468, 6.000000000000002665 ) ;
#26648=CARTESIAN_POINT ( 'NONE',  ( 34.13626153038629951, -3.787416908594791742, -5.295464026636712340 ) ) ;
#26656=CARTESIAN_POINT ( 'NONE',  ( 21.99236933195925658, 1.173799028591102189, -6.729090458912794226 ) ) ;
#26662=CARTESIAN_POINT ( 'NONE',  ( 86.79384979562775015, -0.7021008148363506729, 5.624057257660853182 ) ) ;
#26666=DIRECTION ( 'NONE',  ( 0.000000000000000000, 1.000000000000000000, 0.000000000000000000 ) ) ;
#26674=CARTESIAN_POINT ( 'NONE',  ( 33.88293910487175964, -5.368702826017877960, 1.511118951966003987 ) ) ;
#26675=EDGE_CURVE ( 'NONE', #24927, #14959, #12635, .T. ) ;
#26680=CARTESIAN_POINT ( 'NONE',  ( 19.75425538659450453, 11.81160871140306767, 2.500000000000000444 ) ) ;
#26682=CARTESIAN_POINT ( 'NONE',  ( 21.85643539959776049, -13.25144142801168634, -1.676981927294508345 ) ) ;
#26688=CARTESIAN_POINT ( 'NONE',  ( 14.73615518778700029, -5.027433023050646099, 2.500473092695826072 ) ) ;
#26689=CARTESIAN_POINT ( 'NONE',  ( -79.06668015796786619, 10.34652177153921926, -5.823291136487683595 ) ) ;
#26696=CARTESIAN_POINT ( 'NONE',  ( 31.02880894190926142, -0.3131658439163265695, 5.049194088601750785 ) ) ;
#26699=CARTESIAN_POINT ( 'NONE',  ( 87.35326390485820980, 0.2383925427539270170, 4.560928763750174753 ) ) ;
#26704=CARTESIAN_POINT ( 'NONE',  ( 36.79824929224523089, -3.072007531421248494, 5.949654789713833658 ) ) ;
#26707=CARTESIAN_POINT ( 'NONE',  ( 85.43834401013396018, 2.333645700298356829, -4.102255839672300120 ) ) ;
#26713=DIRECTION ( 'NONE',  ( -1.000000000000000000, 0.000000000000000000, 0.000000000000000000 ) ) ;
#26719=CARTESIAN_POINT ( 'NONE',  ( 24.97416265246179634, 3.401756802687047720, -1.620313636369559829 ) ) ;
#26721=CARTESIAN_POINT ( 'NONE',  ( 23.18800229536432767, 0.6779291438705001838, 5.705356198791737832 ) ) ;
#26731=CARTESIAN_POINT ( 'NONE',  ( 24.60713993353984463, 2.981604336055061477, -3.554838876931238012 ) ) ;
#26736=CARTESIAN_POINT ( 'NONE',  ( 21.85643539959774273, 9.255709152629782110, 0.01215589129642568461 ) ) ;
#26737=CARTESIAN_POINT ( 'NONE',  ( 15.87703778079246852, 7.971370532067864723, 3.484773800359326490 ) ) ;
#26739=AXIS2_PLACEMENT_3D ( 'NONE', #15537, #12022, #6076 ) ;
#26741=CARTESIAN_POINT ( 'NONE',  ( 84.76444386024292044, 2.549623173165235457, -3.635552437183829699 ) ) ;
#26747=CARTESIAN_POINT ( 'NONE',  ( 19.67387626504557119, -2.726682240971237903, -3.276982224292623425 ) ) ;
#26748=CARTESIAN_POINT ( 'NONE',  ( 36.97888601131364794, -2.955670041283646743, -5.977847518440031038 ) ) ;
#26750=CARTESIAN_POINT ( 'NONE',  ( 22.09089903963538504, 0.3679612555529369611, -7.362811209300283544 ) ) ;
#26752=EDGE_LOOP ( 'NONE', ( #21998, #1176, #16186, #10864 ) ) ;
#26753=CARTESIAN_POINT ( 'NONE',  ( 36.90998175379526458, -2.640409580673696244, 5.967093342598490224 ) ) ;
#26759=CARTESIAN_POINT ( 'NONE',  ( 35.83237527962609903, -3.728971877112755795, 5.623842631175056006 ) ) ;
#26761=CIRCLE ( 'NONE', #8994, 7.744449365083023729 ) ;
#26763=VECTOR ( 'NONE', #29969, 1000.000000000000000 ) ;
#26764=CARTESIAN_POINT ( 'NONE',  ( 86.31797065848635953, -0.3216205983069810870, 5.878345525829285378 ) ) ;
#26769=ORIENTED_EDGE ( 'NONE', *, *, #17986, .F. ) ;
#26770=DIRECTION ( 'NONE',  ( -1.000000000000000000, 0.000000000000000000, 0.000000000000000000 ) ) ;
#26772=ORIENTED_EDGE ( 'NONE', *, *, #992, .F. ) ;
#26774=CARTESIAN_POINT ( 'NONE',  ( 22.36021236311070837, 4.293190201525941774, 3.667803422475389930 ) ) ;
#26778=ORIENTED_EDGE ( 'NONE', *, *, #25078, .T. ) ;
#26780=CARTESIAN_POINT ( 'NONE',  ( 23.66263933634246541, -2.671893037885467947, -3.899525170167924770 ) ) ;
#26781=CARTESIAN_POINT ( 'NONE',  ( 20.61566240124719229, 6.034574563953731818, -3.423970728030660826 ) ) ;
#26783=CARTESIAN_POINT ( 'NONE',  ( 21.84425409567527865, 2.562565029795382809, -5.509240067314594924 ) ) ;
#26787=EDGE_CURVE ( 'NONE', #5350, #6564, #3407, .T. ) ;
#26792=CARTESIAN_POINT ( 'NONE',  ( 85.19528866922426857, 2.662332751101227579, -1.941753459690362726 ) ) ;
#26793=CARTESIAN_POINT ( 'NONE',  ( 30.63785892209476458, -0.4682215140425676214, 5.751446082446129537 ) ) ;
#26796=CARTESIAN_POINT ( 'NONE',  ( -79.07517032757485254, -5.439101939624123361, -7.647829796408795566 ) ) ;
#26798=CARTESIAN_POINT ( 'NONE',  ( 14.93018881926248120, -5.919497445998742613, 2.519022926048594346 ) ) ;
#26800=CARTESIAN_POINT ( 'NONE',  ( 36.66731919220198677, -2.423882815175043337, -5.929219981045500631 ) ) ;
#26806=CARTESIAN_POINT ( 'NONE',  ( 37.12958521530237022, -2.935469131982732183, 5.998845046471068976 ) ) ;
#26810=EDGE_LOOP ( 'NONE', ( #33865, #36427, #8265, #3363, #28806, #12880, #18968, #26772, #17673, #29837, #17071, #34145, #16915, #21849, #32508, #34312, #3217, #19294 ) ) ;
#26811=B_SPLINE_CURVE_WITH_KNOTS ( 'NONE', 3,
 ( #8225, #27381, #20795, #4564, #20189, #32775 ),
 .UNSPECIFIED., .F., .F.,
 ( 4, 2, 4 ),
 ( 0.000000000000000000, 0.5000000000000000000, 1.000000000000000000 ),
 .UNSPECIFIED. ) ;
#26813=FACE_OUTER_BOUND ( 'NONE', #3873, .T. ) ;
#26814=CARTESIAN_POINT ( 'NONE',  ( 86.09291566217842728, 0.07834183196763176704, -5.989438611547945435 ) ) ;
#26815=CARTESIAN_POINT ( 'NONE',  ( 85.14718662316111875, 1.669408076102861349, -5.191970801932679791 ) ) ;
#26820=CARTESIAN_POINT ( 'NONE',  ( 22.87852314092918604, 4.327528820093371920, 3.073438435473089481 ) ) ;
#26825=CARTESIAN_POINT ( 'NONE',  ( 27.44649324819909353, 0.9063735473286961275, 4.490087085965837943 ) ) ;
#26826=CARTESIAN_POINT ( 'NONE',  ( 14.78205480818345130, -5.168698993129799746, -2.499999999988669508 ) ) ;
#26831=CARTESIAN_POINT ( 'NONE',  ( 36.34168992152566346, -3.603234009378773806, -5.757187825781041823 ) ) ;
#26835=CARTESIAN_POINT ( 'NONE',  ( 23.91855504425362255, 4.211737807167565961, 0.007810489111244203406 ) ) ;
#26838=CARTESIAN_POINT ( 'NONE',  ( -80.33671669984387620, -5.680595701363414740, 3.413160419656412259 ) ) ;
#26839=CARTESIAN_POINT ( 'NONE',  ( 22.29352313805566155, 0.2601191645372996630, -7.110266727710765622 ) ) ;
#26843=CARTESIAN_POINT ( 'NONE',  ( 33.11223012084407458, -0.1537037112411065998, -4.945624661800740007 ) ) ;
#26844=LINE ( 'NONE', #20655, #15432 ) ;
#26852=CARTESIAN_POINT ( 'NONE',  ( 22.24669285715049938, 1.156305209326864425, -6.358976223308567377 ) ) ;
#26857=CARTESIAN_POINT ( 'NONE',  ( 85.39947451146549895, 1.536583868559685762, 5.410284084896357371 ) ) ;
#26876=CARTESIAN_POINT ( 'NONE',  ( 21.85643539959772497, -13.01485165473748573, 3.478087416278500932 ) ) ;
#26879=CARTESIAN_POINT ( 'NONE',  ( -77.23777935285242791, 9.655128411724760440, 7.769674086704672966 ) ) ;
#26880=CARTESIAN_POINT ( 'NONE',  ( 14.77590839487426777, -5.162981251534658256, 2.500001664204352547 ) ) ;
#26881=B_SPLINE_CURVE_WITH_KNOTS ( 'NONE', 3,
 ( #39999, #11769, #24349, #26291, #36913, #11979, #23192, #2559, #15081, #35568, #7336, #19896, #33225, #36706 ),
 .UNSPECIFIED., .F., .F.,
 ( 4, 2, 2, 2, 2, 2, 4 ),
 ( 0.000000000000000000, 0.0003684622442568309176, 0.0005526933663852468372, 0.0006448089274494569383, 0.0006908667079815606878, 0.0007138955982476137552, 0.0007369244885136669310 ),
 .UNSPECIFIED. ) ;
#26882=CARTESIAN_POINT ( 'NONE',  ( -79.20124688682111014, 10.32858273165098595, -7.499809273847732882 ) ) ;
#26890=CARTESIAN_POINT ( 'NONE',  ( -70.05488178572183244, -0.2788347306335496323, 9.961904852117910991 ) ) ;
#26895=CARTESIAN_POINT ( 'NONE',  ( 36.46939072216235189, -2.309382896708789268, 5.898328456377949003 ) ) ;
#26900=CARTESIAN_POINT ( 'NONE',  ( 87.85599567641696694, -0.3262996441500809475, -4.386575958041428080 ) ) ;
#26902=CARTESIAN_POINT ( 'NONE',  ( 33.61667494505991982, -1.223710831992580239, -5.453093166169209915 ) ) ;
#26907=ORIENTED_EDGE ( 'NONE', *, *, #11639, .F. ) ;
#26915=CARTESIAN_POINT ( 'NONE',  ( 25.51906755988597553, 1.283014276674031340, 4.421375708069085420 ) ) ;
#26926=CARTESIAN_POINT ( 'NONE',  ( 24.26931705048690446, 3.117373144333289936, -3.494565216830213927 ) ) ;
#26930=CARTESIAN_POINT ( 'NONE',  ( 22.37440129197860728, 3.331413251109061058, -7.657642981191555620 ) ) ;
#26933=CARTESIAN_POINT ( 'NONE',  ( 85.11033487576473533, 2.122656363318763173, 4.626068480629312418 ) ) ;
#26937=CARTESIAN_POINT ( 'NONE',  ( -79.28861043050481783, -5.487522343443236750, 7.393227751528659297 ) ) ;
#26939=CARTESIAN_POINT ( 'NONE',  ( 21.58863023475808873, 7.202558683720228672, -2.923977588977705544 ) ) ;
#26940=VECTOR ( 'NONE', #2603, 1000.000000000000000 ) ;
#26941=CARTESIAN_POINT ( 'NONE',  ( 23.83525155650060867, -3.101377793311910658, -3.828427711158430835 ) ) ;
#26942=CARTESIAN_POINT ( 'NONE',  ( 33.46291576196824025, -3.080929388775397015, -5.429095326967858348 ) ) ;
#26944=CARTESIAN_POINT ( 'NONE',  ( 24.12374896606528552, 0.5377693420488547371, -5.092152185932238062 ) ) ;
#26946=VERTEX_POINT ( 'NONE', #32991 ) ;
#26947=FACE_OUTER_BOUND ( 'NONE', #29407, .T. ) ;
#26951=CARTESIAN_POINT ( 'NONE',  ( 37.17729982316707549, -2.564139253649980521, 5.980890902488024352 ) ) ;
#26955=CARTESIAN_POINT ( 'NONE',  ( 20.13561717962239328, -3.050796925077462696, -3.278976415860665572 ) ) ;
#26961=ORIENTED_EDGE ( 'NONE', *, *, #40033, .F. ) ;
#26964=EDGE_LOOP ( 'NONE', ( #3319, #8525, #22233, #34286 ) ) ;
#26966=ORIENTED_EDGE ( 'NONE', *, *, #17621, .T. ) ;
#26968=CARTESIAN_POINT ( 'NONE',  ( 21.90912465240509732, 3.662607847369724556, 2.128491611106550607 ) ) ;
#26970=CARTESIAN_POINT ( 'NONE',  ( 23.87850738558080366, 3.138038174018865423, 3.674020033097090909 ) ) ;
#26976=CARTESIAN_POINT ( 'NONE',  ( 25.88797439567527903, -2.749903636904698967, -4.246842526108601135 ) ) ;
#26980=CARTESIAN_POINT ( 'NONE',  ( 22.46204726948479546, 2.974089873731441624, -4.569747218150055801 ) ) ;
#26987=CARTESIAN_POINT ( 'NONE',  ( 85.88709644997106807, 1.885261416588465799, 4.127327262050844325 ) ) ;
#26988=CARTESIAN_POINT ( 'NONE',  ( 32.93308485139972674, -2.920656968542761245, -5.757540729513444866 ) ) ;
#26990=CARTESIAN_POINT ( 'NONE',  ( -76.13539268176610619, -4.086280762280473766, -9.992012468020183391 ) ) ;
#26991=CARTESIAN_POINT ( 'NONE',  ( 16.27325576391341500, -3.466558749124218686, 2.727822142381055137 ) ) ;
#26993=CARTESIAN_POINT ( 'NONE',  ( 21.35934244005222737, 3.587024235528914584, -3.540039984054675681 ) ) ;
#26996=DIRECTION ( 'NONE',  ( 0.000000000000000000, 0.000000000000000000, -1.000000000000000000 ) ) ;
#27003=CARTESIAN_POINT ( 'NONE',  ( 29.45347667344336884, 1.169340884980286877, 4.331142282593965831 ) ) ;
#27006=CARTESIAN_POINT ( 'NONE',  ( -71.72747510529796955, -0.1678074918106684243, 9.968450010350146329 ) ) ;
#27009=EDGE_LOOP ( 'NONE', ( #27589, #3262, #23270, #33169, #22888, #24555, #26778, #24749, #4120 ) ) ;
#27011=CARTESIAN_POINT ( 'NONE',  ( 86.00533037392021640, 0.2452800639758652423, -6.000000104874900764 ) ) ;
#27012=CARTESIAN_POINT ( 'NONE',  ( 84.97881024039070041, 1.902655756596536518, -4.858038791751294383 ) ) ;
#27013=CARTESIAN_POINT ( 'NONE',  ( -18.48280404870591553, -63.98126818465317456, 2.500000000000000000 ) ) ;
#27017=CARTESIAN_POINT ( 'NONE',  ( 23.14039851168018558, 4.035316712620898194, 3.101781372617715249 ) ) ;
#27024=VECTOR ( 'NONE', #1475, 1000.000000000000000 ) ;
#27025=CARTESIAN_POINT ( 'NONE',  ( 23.04469232822262725, 0.3231521739056994469, 5.972309192691233726 ) ) ;
#27026=CARTESIAN_POINT ( 'NONE',  ( 14.77498549067719935, -5.165673680530092682, -2.500001149280607571 ) ) ;
#27031=CARTESIAN_POINT ( 'NONE',  ( 34.20739662544301041, -3.854094502681030932, -5.250102797243501485 ) ) ;
#27037=CARTESIAN_POINT ( 'NONE',  ( 30.11529565287584020, -4.511537616843412479, 1.859944388213511157 ) ) ;
#27039=CARTESIAN_POINT ( 'NONE',  ( -7.890026461918812295, -8.913725925455491250, 6.000000000000000000 ) ) ;
#27041=CARTESIAN_POINT ( 'NONE',  ( -81.77390411455343155, -5.606086203577094196, 1.137401704552885251 ) ) ;
#27042=CARTESIAN_POINT ( 'NONE',  ( 26.06502655271711433, 0.7650683268001282622, -4.421515112517789170 ) ) ;
#27044=B_SPLINE_CURVE_WITH_KNOTS ( 'NONE', 3,
 ( #40374, #27624, #17942, #36691, #21257, #39780 ),
 .UNSPECIFIED., .F., .F.,
 ( 4, 2, 4 ),
 ( 0.000000000000000000, 0.5000000000000001110, 1.000000000000000000 ),
 .UNSPECIFIED. ) ;
#27047=CARTESIAN_POINT ( 'NONE',  ( 27.81486881904474018, 1.842726162330621476, -3.911115716677233678 ) ) ;
#27052=CARTESIAN_POINT ( 'NONE',  ( -70.92837670882106238, -48.61702805680358352, 6.000000000000002665 ) ) ;
#27056=EDGE_LOOP ( 'NONE', ( #27509, #12324, #15671, #9699, #21356, #184 ) ) ;
#27057=CARTESIAN_POINT ( 'NONE',  ( -70.17127749215180188, -48.42661992061006515, 5.954803573902830216 ) ) ;
#27063=CARTESIAN_POINT ( 'NONE',  ( 87.78960583812504126, -2.347739977990699778, 2.116702103816012759 ) ) ;
#27070=PRODUCT_CONTEXT ( 'NONE', #13950, 'mechanical' ) ;
#27077=CARTESIAN_POINT ( 'NONE',  ( 16.91049444498251120, 9.757949283939643337, -2.500000000000007105 ) ) ;
#27082=CARTESIAN_POINT ( 'NONE',  ( -80.92837670882107659, 2.429809908903242555, 12.50000000000000000 ) ) ;
#27083=CARTESIAN_POINT ( 'NONE',  ( 21.85643539959773207, -9.550271554086487313, -10.69920392963802769 ) ) ;
#27085=CARTESIAN_POINT ( 'NONE',  ( -79.28028571780328093, 10.39372739289916758, 5.513573824196321027 ) ) ;
#27086=CARTESIAN_POINT ( 'NONE',  ( 14.78293163467730587, -5.166176174648792419, 2.500000000038486547 ) ) ;
#27087=CARTESIAN_POINT ( 'NONE',  ( -73.24681673169105522, 4.967639606635550820, -10.91583103658519960 ) ) ;
#27099=CARTESIAN_POINT ( 'NONE',  ( 36.42112393931954273, -3.116698823254151041, 5.890795257578658628 ) ) ;
#27102=CARTESIAN_POINT ( 'NONE',  ( 88.18839210903504977, -0.8832026502337909646, 4.329116466421397469 ) ) ;
#27104=CARTESIAN_POINT ( 'NONE',  ( -71.43230626105646763, -21.65663085445836344, 5.980032331837192849 ) ) ;
#27115=CARTESIAN_POINT ( 'NONE',  ( 21.89417189222532301, 0.4921803897989117105, 7.737752117221773140 ) ) ;
#27122=CARTESIAN_POINT ( 'NONE',  ( 87.04213330793392345, 0.5878691963682337596, -6.000000000000000000 ) ) ;
#27124=CARTESIAN_POINT ( 'NONE',  ( 14.61802081865033642, -4.461995682952384357, -2.500000000000000000 ) ) ;
#27127=CARTESIAN_POINT ( 'NONE',  ( 23.67152737812504526, 3.427402071259508354, -3.470193783917488783 ) ) ;
#27128=ORIENTED_EDGE ( 'NONE', *, *, #24443, .T. ) ;
#27130=CARTESIAN_POINT ( 'NONE',  ( 22.63837051618441620, -3.414681707391253429, 8.302592004085083133 ) ) ;
#27131=DIRECTION ( 'NONE',  ( 1.000000000000000000, 0.000000000000000000, 0.000000000000000000 ) ) ;
#27134=CARTESIAN_POINT ( 'NONE',  ( 87.83080901603209156, -0.9320485544948414747, 4.955211484752597428 ) ) ;
#27139=CARTESIAN_POINT ( 'NONE',  ( 14.92610986758655045, -6.101699263985318922, -2.531194043802452942 ) ) ;
#27140=CARTESIAN_POINT ( 'NONE',  ( 36.91003892329680980, -2.640456672357779144, -5.967102265281861051 ) ) ;
#27142=CARTESIAN_POINT ( 'NONE',  ( 25.90788401527250429, 0.9445445186425489581, -4.431966072703408699 ) ) ;
#27143=CARTESIAN_POINT ( 'NONE',  ( 33.46397865298071395, -3.088978469517898340, -5.429261216816389179 ) ) ;
#27145=CARTESIAN_POINT ( 'NONE',  ( 34.13642104789413878, -3.131480944053012028, 5.534212115622173300 ) ) ;
#27148=EDGE_CURVE ( 'NONE', #6701, #12553, #3547, .T. ) ;
#27151=CARTESIAN_POINT ( 'NONE',  ( 34.79267513315475924, -3.836925689216892366, 5.375550132972651163 ) ) ;
#27157=EDGE_LOOP ( 'NONE', ( #10451, #11401, #27538, #5777 ) ) ;
#27166=CARTESIAN_POINT ( 'NONE',  ( 24.11084648476953873, 3.002081633687809337, 3.727765853929763118 ) ) ;
#27171=CARTESIAN_POINT ( 'NONE',  ( 19.65961218291280233, -2.698309273198196134, -3.274755969297673097 ) ) ;
#27172=DIRECTION ( 'NONE',  ( 1.000000000000000000, 0.000000000000000000, -0.000000000000000000 ) ) ;
#27175=CARTESIAN_POINT ( 'NONE',  ( 23.22712546262786049, 2.410586217767674899, -4.514815941842217129 ) ) ;
#27176=ORIENTED_EDGE ( 'NONE', *, *, #766, .T. ) ;
#27178=CARTESIAN_POINT ( 'NONE',  ( 17.49770824240842870, -6.259500660934115501, 2.499999999999995115 ) ) ;
#27183=CARTESIAN_POINT ( 'NONE',  ( 85.49511565994269802, 2.325552844478905090, -3.343772400554256397 ) ) ;
#27190=DIRECTION ( 'NONE',  ( 0.000000000000000000, -0.000000000000000000, -1.000000000000000000 ) ) ;
#27193=CARTESIAN_POINT ( 'NONE',  ( 33.44985200980665496, -3.250795928539166102, -5.427056412495004700 ) ) ;
#27200=EDGE_CURVE ( 'NONE', #28666, #5954, #37673, .T. ) ;
#27202=CARTESIAN_POINT ( 'NONE',  ( 35.67313104109378230, -1.412451363119313852, 5.626408984427851756 ) ) ;
#27205=CARTESIAN_POINT ( 'NONE',  ( -72.84815947045233031, 2.429809908903064919, -10.96147798754375202 ) ) ;
#27206=EDGE_LOOP ( 'NONE', ( #20942, #14748, #24773 ) ) ;
#27207=DIRECTION ( 'NONE',  ( 1.000000000000000000, 8.398074759113475787E-17, -0.000000000000000000 ) ) ;
#27208=CARTESIAN_POINT ( 'NONE',  ( 86.00134810727946899, 0.2530519298808260320, -5.999722280616810899 ) ) ;
#27214=CARTESIAN_POINT ( 'NONE',  ( 24.72551563480591241, 3.007151916241646017, 3.409849726662557590 ) ) ;
#27221=CARTESIAN_POINT ( 'NONE',  ( 23.58969270755171976, 0.4216153867694091839, 5.525703236370836713 ) ) ;
#27222=CARTESIAN_POINT ( 'NONE',  ( 14.67750890824153487, -4.951417047788147840, -2.499999999999853895 ) ) ;
#27226=CARTESIAN_POINT ( 'NONE',  ( 36.01029390836630029, -3.690187617478303483, -5.670464297519259844 ) ) ;
#27232=CARTESIAN_POINT ( 'NONE',  ( 26.98641761431236930, 1.293889648236598022, -5.140668381306381818 ) ) ;
#27236=CARTESIAN_POINT ( 'NONE',  ( 26.74579300571716800, 0.9069395800068310587, -4.382589997453513853 ) ) ;
#27238=CARTESIAN_POINT ( 'NONE',  ( -4.444218661349752963, -35.94265729135299381, 6.000000000000000000 ) ) ;
#27242=CARTESIAN_POINT ( 'NONE',  ( 35.72977957149858241, -1.305545292155645187, -5.539037271891777969 ) ) ;
#27244=CARTESIAN_POINT ( 'NONE',  ( 27.43879703630890887, 0.9604363013853572939, -4.488885905966782275 ) ) ;
#27252=CARTESIAN_POINT ( 'NONE',  ( 24.93942215624759484, 2.519938839411334897, -3.978906813874826920 ) ) ;
#27263=CARTESIAN_POINT ( 'NONE',  ( 22.88299028827532666, 4.349279440556175658, 3.031013114583645418 ) ) ;
#27268=CARTESIAN_POINT ( 'NONE',  ( 18.79220261045992046, 6.725182846677081550, -3.484773916742352817 ) ) ;
#27278=CARTESIAN_POINT ( 'NONE',  ( 21.85643539959778181, 11.38078789530947788, 4.862784767728865809 ) ) ;
#27283=CARTESIAN_POINT ( 'NONE',  ( 14.77222812468941449, -4.461849342347315783, 2.511961485181791520 ) ) ;
#27284=EDGE_CURVE ( 'NONE', #1864, #7, #38898, .T. ) ;
#27285=CARTESIAN_POINT ( 'NONE',  ( -74.09550586375644343, 6.760974547859217587, -10.75457049036731938 ) ) ;
#27289=CARTESIAN_POINT ( 'NONE',  ( 14.71123721502443082, 12.78438965696137863, 2.502442378657849353 ) ) ;
#27298=CARTESIAN_POINT ( 'NONE',  ( 31.72026365724324393, -0.5546405064503883153, 5.157112319825081670 ) ) ;
#27302=VECTOR ( 'NONE', #30002, 1000.000000000000000 ) ;
#27303=CARTESIAN_POINT ( 'NONE',  ( 87.06807637922989329, 0.009568187950425697044, -5.830412620327568796 ) ) ;
#27304=CARTESIAN_POINT ( 'NONE',  ( 8.290806648384990041, 0.000000000000000000, 2.500000000000000000 ) ) ;
#27307=FACE_OUTER_BOUND ( 'NONE', #28990, .T. ) ;
#27309=CARTESIAN_POINT ( 'NONE',  ( -70.05507390326904726, -21.28749960934529639, 5.936322957303396208 ) ) ;
#27311=CARTESIAN_POINT ( 'NONE',  ( -17.69482985384421880, -42.37473357531882101, 6.000000000000000000 ) ) ;
#27312=EDGE_LOOP ( 'NONE', ( #24791, #1021 ) ) ;
#27317=CARTESIAN_POINT ( 'NONE',  ( 23.13594544608132964, 0.4166732799763251949, 5.866887071280732613 ) ) ;
#27322=CARTESIAN_POINT ( 'NONE',  ( 66.41194937274630661, -13.65448019739280028, -6.000000000000000000 ) ) ;
#27327=CARTESIAN_POINT ( 'NONE',  ( 22.41749760006145209, 4.809556558396148596, -3.145958556896370606 ) ) ;
#27328=ORIENTED_EDGE ( 'NONE', *, *, #17278, .F. ) ;
#27332=CARTESIAN_POINT ( 'NONE',  ( 25.51676067120702740, -4.685157242005201006, -0.9133679171623337867 ) ) ;
#27338=CARTESIAN_POINT ( 'NONE',  ( 85.61743365444765175, 1.218782235343771836, 5.694237175320765232 ) ) ;
#27339=CARTESIAN_POINT ( 'NONE',  ( -17.27251170661583402, 3.729367930467589076, 2.500000000000000000 ) ) ;
#27343=ORIENTED_EDGE ( 'NONE', *, *, #18609, .F. ) ;
#27345=CARTESIAN_POINT ( 'NONE',  ( 16.06814633003477510, -3.505435886482454411, -2.701413578244389324 ) ) ;
#27352=CARTESIAN_POINT ( 'NONE',  ( 87.93559242015480493, -0.4157064846058496355, 3.292354338654781998 ) ) ;
#27354=ORIENTED_EDGE ( 'NONE', *, *, #14385, .T. ) ;
#27356=CARTESIAN_POINT ( 'NONE',  ( 30.88427062897021713, 0.7007091440377163361, 4.489139483277927667 ) ) ;
#27357=CARTESIAN_POINT ( 'NONE',  ( 20.92499718081190352, -2.659581275971057757, 3.472249901671649042 ) ) ;
#27358=CARTESIAN_POINT ( 'NONE',  ( 17.83173683073222549, -3.184001612988465624, -2.948685647352225825 ) ) ;
#27363=ORIENTED_EDGE ( 'NONE', *, *, #17175, .F. ) ;
#27364=CARTESIAN_POINT ( 'NONE',  ( 0.6783104270758654186, -48.60743831809499227, 2.500000000000000000 ) ) ;
#27366=MECHANICAL_DESIGN_GEOMETRIC_PRESENTATION_REPRESENTATION('',(#2423),#26159);
#27368=VERTEX_POINT ( 'NONE', #10492 ) ;
#27369=CARTESIAN_POINT ( 'NONE',  ( 22.86800780692831481, 3.053438318512094352, 4.223698497200296664 ) ) ;
#27376=CARTESIAN_POINT ( 'NONE',  ( 26.16633878416043757, -2.761556949326915866, -4.290288021199886614 ) ) ;
#27379=CARTESIAN_POINT ( 'NONE',  ( 22.63225339419747328, 3.325388178310765941, -4.169375494914318914 ) ) ;
#27381=CARTESIAN_POINT ( 'NONE',  ( 16.13270506554978923, 15.26110145415460195, 1.497002735631780768 ) ) ;
#27387=CARTESIAN_POINT ( 'NONE',  ( 87.11756278340992310, 0.5031432294147388795, -4.836983121871330837 ) ) ;
#27388=CARTESIAN_POINT ( 'NONE',  ( 29.20166386951125048, 2.268204792580242213, 0.006282727923920283265 ) ) ;
#27391=CARTESIAN_POINT ( 'NONE',  ( 15.00253043624129212, -6.083877922989610276, 2.528644475646949275 ) ) ;
#27393=CARTESIAN_POINT ( 'NONE',  ( 35.78605622417325804, -3.164553250030355258, -5.791677581459363289 ) ) ;
#27396=AXIS2_PLACEMENT_3D ( 'NONE', #9227, #38246, #6365 ) ;
#27403=CARTESIAN_POINT ( 'NONE',  ( 36.20067509515345705, -3.648475481699166689, 5.719151051457621371 ) ) ;
#27410=CARTESIAN_POINT ( 'NONE',  ( -71.75878675104897297, 2.184363218556831132, -9.965500343853747722 ) ) ;
#27411=CARTESIAN_POINT ( 'NONE',  ( 17.27299901063489074, 8.731752785486881052, 2.902267263306012701 ) ) ;
#27413=EDGE_CURVE ( 'NONE', #4341, #13546, #35969, .T. ) ;
#27417=CARTESIAN_POINT ( 'NONE',  ( 21.85364604960087220, 5.828349873347765886, 3.192828959171670533 ) ) ;
#27419=CARTESIAN_POINT ( 'NONE',  ( 14.77500745536057813, -5.175466302041957789, 2.500000552286355759 ) ) ;
#27424=ORIENTED_EDGE ( 'NONE', *, *, #37090, .F. ) ;
#27426=B_SPLINE_CURVE_WITH_KNOTS ( 'NONE', 3,
 ( #5950, #14384, #22225, #28591, #9849, #37627, #25304, #12320, #6158, #19118, #3704, #31685, #22627, #602, #22424, #31078 ),
 .UNSPECIFIED., .F., .F.,
 ( 4, 2, 2, 2, 2, 2, 2, 4 ),
 ( 0.002348712775360395008, 0.002642162077394872178, 0.002935611379429349348, 0.003522509983498256850, 0.003815959285532717973, 0.004109408587567179097, 0.004402857889601640221, 0.004696307191636101344 ),
 .UNSPECIFIED. ) ;
#27427=CARTESIAN_POINT ( 'NONE',  ( 26.76647894427393837, 0.8302801056813566838, 4.383954407630289651 ) ) ;
#27428=CARTESIAN_POINT ( 'NONE',  ( 14.78228770234103351, -5.167964840227161183, -2.500001186442457168 ) ) ;
#27432=VECTOR ( 'NONE', #6242, 1000.000000000000000 ) ;
#27433=EDGE_LOOP ( 'NONE', ( #25444, #34409, #30459, #4998, #7414, #27363, #19123, #39321 ) ) ;
#27440=PLANE ( 'NONE',  #5143 ) ;
#27442=CARTESIAN_POINT ( 'NONE',  ( 27.87477497239535396, 2.606304449749688779, 1.085873857364543671 ) ) ;
#27444=DIRECTION ( 'NONE',  ( -0.000000000000000000, -0.000000000000000000, -1.000000000000000000 ) ) ;
#27446=CARTESIAN_POINT ( 'NONE',  ( 23.07038014192270126, 0.3568886247812357304, -5.941770054002118329 ) ) ;
#27451=CARTESIAN_POINT ( 'NONE',  ( 36.13184693646208956, -1.532129719049094119, -5.644433108115570974 ) ) ;
#27453=CARTESIAN_POINT ( 'NONE',  ( 27.35387344454971270, 1.116497774337839477, -4.475331455587648222 ) ) ;
#27454=DIRECTION ( 'NONE',  ( -0.000000000000000000, -0.000000000000000000, -1.000000000000000000 ) ) ;
#27457=CARTESIAN_POINT ( 'NONE',  ( -72.84815947045163398, 2.833900941398741047, 10.96147798754381064 ) ) ;
#27458=EDGE_CURVE ( 'NONE', #12570, #23904, #10435, .T. ) ;
#27461=CARTESIAN_POINT ( 'NONE',  ( 25.25242209220571254, 2.014110669997101422, -4.189051521245521492 ) ) ;
#27468=CARTESIAN_POINT ( 'NONE',  ( 87.12371845299759343, -1.516527252418922833, -4.675789953527256237 ) ) ;
#27470=CARTESIAN_POINT ( 'NONE',  ( 21.67762503442624222, 6.625004204850643674, 3.088539990067460828 ) ) ;
#27479=CARTESIAN_POINT ( 'NONE',  ( 21.71040439744254513, 6.342537115183759511, 3.188214735634443908 ) ) ;
#27486=CARTESIAN_POINT ( 'NONE',  ( 21.04004256178996002, 8.045166779822325864, -2.500000000010173640 ) ) ;
#27492=CARTESIAN_POINT ( 'NONE',  ( 17.39327739772060255, 14.24814301257567273, 2.500000000000000444 ) ) ;
#27493=CARTESIAN_POINT ( 'NONE',  ( 22.40835304001176098, 2.012838380346585243, -8.570566085397546274 ) ) ;
#27495=CARTESIAN_POINT ( 'NONE',  ( -77.90426910868221455, 9.924495015397090114, 8.801360606586941415 ) ) ;
#27496=CARTESIAN_POINT ( 'NONE',  ( 37.06374037821629486, -3.173191448149650373, 5.964198512422226983 ) ) ;
#27498=CARTESIAN_POINT ( 'NONE',  ( -78.36759592796440188, 10.14500944777191371, -6.694231243261347331 ) ) ;
#27508=CARTESIAN_POINT ( 'NONE',  ( 24.37979543224318846, 2.943268363220738149, -3.716964114009788656 ) ) ;
#27509=ORIENTED_EDGE ( 'NONE', *, *, #13335, .T. ) ;
#27511=CARTESIAN_POINT ( 'NONE',  ( 34.93082455767837757, -1.706425845107903960, 5.658197996046836487 ) ) ;
#27515=CARTESIAN_POINT ( 'NONE',  ( 86.38515361113813640, 1.239318396469950123, 5.566871328843018496 ) ) ;
#27517=CARTESIAN_POINT ( 'NONE',  ( 30.63785892209476458, -0.4682215140425676214, 5.751446082446129537 ) ) ;
#27518=CARTESIAN_POINT ( 'NONE',  ( 32.07397980944352156, -0.6787160600116808329, -5.212318280033424678 ) ) ;
#27537=CARTESIAN_POINT ( 'NONE',  ( 21.86457316608978019, 5.764392919207080190, -3.219569754713741183 ) ) ;
#27538=ORIENTED_EDGE ( 'NONE', *, *, #17362, .F. ) ;
#27540=CARTESIAN_POINT ( 'NONE',  ( 24.06190720129734473, 2.407014782553678955, 5.659300396313236448 ) ) ;
#27544=CARTESIAN_POINT ( 'NONE',  ( 87.87138265328074738, -2.102315541244656583, 2.954904511526853295 ) ) ;
#27545=DIRECTION ( 'NONE',  ( 0.000000000000000000, 0.000000000000000000, 1.000000000000000000 ) ) ;
#27550=CARTESIAN_POINT ( 'NONE',  ( 19.69399097454885705, -2.982692120004300840, -3.239409980100296238 ) ) ;
#27552=B_SPLINE_SURFACE_WITH_KNOTS ( 'NONE', 3, 3, ( 
 ( #22357, #38574, #4030, #25628, #25835, #31816, #13466, #16156, #3435, #7291, #38173, #29129, #38780 ),
 ( #22556, #38370, #13678, #19453, #3832, #19658, #15948, #28512, #10167, #35119, #322, #25428, #16352 ),
 ( #37969, #26040, #7094, #35326, #6700, #16548, #19249, #3631, #28720, #23938, #39802, #2147, #14268 ),
 ( #11169, #36311, #27042, #29920, #1341, #30134, #1949, #8082, #23740, #5015, #33450, #39586, #38971 ),
 ( #20648, #39379, #32632, #35918, #33229, #1531, #7697, #17546, #30340, #26839, #11371, #36510, #8283 ),
 ( #5218, #36117, #14467, #4427, #20246, #35717, #20858, #17753, #29721, #14065, #20446, #17342, #23552 ),
 ( #14665, #27236, #11572, #13877, #16951, #7493, #20053, #29529, #26444, #10770, #4619, #1737, #23346 ),
 ( #32828, #17149, #26642, #39176, #10972, #7894, #33025, #4815, #6241, #18785, #37515, #37316, #8696 ),
 ( #33646, #9310, #24560, #2355, #5626, #14874, #28254, #27446, #40397, #40002, #2562, #31159, #8491 ),
 ( #21689, #11772, #24770, #34466, #9114, #21072, #34267, #5421, #6038, #34061, #8900, #24352, #15291 ),
 ( #2766, #27844, #36916, #21276, #15084, #12199, #21483, #24978, #27645, #40603, #5834, #30961, #18573 ),
 ( #2975, #15494, #18374, #28054, #12409, #39076, #17863, #5328, #39289, #1852, #31018, #8186, #14374 ),
 ( #37573, #33553, #18634, #6097, #34326, #26944, #12470, #2055, #12257, #11077, #39486, #1642, #31219 ),
 ( #36414, #20758, #27142, #24046, #30240, #17447, #2827, #27904, #20973, #20550, #23647, #37376, #24831 ),
 ( #36615, #15348, #9370, #7994, #23839, #36214, #40448, #21744, #3039, #33134, #9172, #6301, #4917 ),
 ( #25040, #15557, #14180, #28114, #11276, #40666, #8399, #21954, #30037, #34528, #26750, #18850, #33349 ),
 ( #5125, #17658, #14568, #39694, #11482, #7306, #25643, #15766, #28733, #25848, #29140, #38587, #25244 ),
 ( #31624, #3450, #31423, #28322, #947, #3644, #37774, #3247, #26056, #12877, #35136, #741, #137 ),
 ( #13276, #22162, #38186, #15965, #38383, #37987, #12669, #7109, #9788, #10186, #22968, #13482, #19264 ),
 ( #10393, #13081, #9988, #3849, #9583, #35532, #22568, #34936, #34735, #6513, #19468, #19061, #32041 ),
 ( #16367, #28938, #22772, #35339, #19670, #32248, #33036, #39601, #1160, #4440, #26852, #26656, #39392 ),
 ( #29541, #27461, #33863, #24577, #30356, #8505, #30976, #8711, #21089, #2579, #2373, #18184, #2161 ),
 ( #27859, #12216, #5436, #15307, #9130, #8298, #30775, #37129, #2782, #14891, #40016, #40410, #24788 ),
 ( #5645, #24369, #20874, #5233, #15100, #17769, #14682, #39820, #11588, #24165, #8917, #27660, #40214 ),
 ( #27252, #17976, #30563, #18390, #11997, #21501, #34078, #5852, #39732, #10710, #26578, #1281, #30073 ),
 ( #36447, #26387, #17481, #8429, #7636, #17694, #27175, #8222, #16888, #30274, #17088, #4955, #26783 ),
 ( #13817, #2090, #29470, #39322, #23288, #4562, #20187, #7835, #1885, #14603, #29661, #21008, #11111 ),
 ( #29864, #39524, #11514, #24081, #33168, #1679, #5158, #14008, #20793, #4751, #23682, #11307, #38917 ),
 ( #14410, #36650, #33388, #32772, #4368, #20582, #8025, #35858, #1474, #26980, #10914, #39118, #23872 ),
 ( #36249, #23491, #36057, #20385, #32965, #17286, #14210, #2910, #2287, #33785, #33586, #9250, #9048 ),
 ( #11922, #18309, #15229, #21421, #8637, #37256, #18514, #12130, #11716, #30482, #27990, #15429, #19 ),
 ( #21625, #28190, #39942, #15025, #14812, #31100, #12345, #24918, #27379, #5974, #37651, #36853, #6180 ),
 ( #37453, #5362, #18722, #5562, #34206, #27783, #40337, #24291, #31304, #17901, #24708, #21213, #18103 ),
 ( #37051, #40536, #3128, #30694, #9453, #21828, #2501, #30900, #34408, #15643, #12549, #27588, #25119 ),
 ( #40140, #24497, #8837, #33996, #5771, #2709, #22037, #16634, #19140, #25726, #32131, #31504, #13563 ),
 ( #12751, #9665, #22650, #7185, #35216, #4121, #6987, #29218, #19554, #31913, #6791, #37862, #13166 ),
 ( #622, #38269, #25328, #26135, #10064, #211, #38668, #1028, #34613, #16046, #32323, #6390, #18939 ),
 ( #16445, #22845, #12960, #25525, #19746, #3328, #3724, #28819, #38070, #15846, #28403, #28614, #22252 ),
 ( #34819, #6595, #31707, #3929, #9872, #22447, #3523, #25929, #29020, #35418, #421, #824, #35015 ),
 ( #13355, #19343, #16249, #38463, #10265, #36197, #30016, #1834, #32518, #23631, #14552, #13768, #23821 ),
 ( #14356, #23046, #36397, #23241, #11060, #32913, #4703, #19939, #8170, #35611, #17238, #16838, #10662 ),
 ( #7976, #20739, #35809, #27127, #29811, #7382, #36005, #4897, #33327, #17640, #4316, #20530, #7584 ),
 ( #10466, #29422, #5106, #23439, #1236, #26339, #30220, #20139, #14157, #33116, #38871, #2037, #17428 ),
 ( #32719, #26926, #4515, #39469, #17034, #11256, #29610, #1429, #20332, #7784, #13962, #1622, #26529 ),
 ( #26731, #39063, #10860, #39268, #27734, #24445, #40482, #8587, #15382, #40089, #5720, #34157, #33536 ),
 ( #12293, #33944, #21165, #40289, #2453, #24654, #18258, #17846, #36600, #5926, #8998, #6131, #37406 ),
 ( #33731, #21368, #18667, #15176, #3075, #15593, #30428, #39677, #27327, #2238, #5510, #27537, #21781 ),
 ( #24866, #12077, #36800, #11868, #8378, #9201, #37003, #5310, #18054, #14758, #31256, #39891, #37204 ),
 ( #30643, #18465, #11459, #14977, #21578, #11665, #8784, #2859, #27939, #30851, #2657, #34359, #24027 ),
 ( #20953, #3879, #6544, #10013, #19698, #25876, #3472, #19291, #10216, #28563, #25474, #576, #37605 ),
 ( #9820, #31659, #771, #34564, #15994, #7138, #6336, #22596, #28767, #22399, #13303, #34966, #13115 ),
 ( #6741, #31455, #32273, #4072, #16200, #12906, #28968, #37808, #16395, #371, #31858, #35164, #21988 ),
 ( #38416, #3676, #9613, #25673, #38019, #38216, #18886, #28145, #22796, #35368, #22199, #40699, #12501 ),
 ( #6936, #19500, #25071, #19089, #32074, #9401, #3279, #15801, #28354, #165, #12702, #25276, #35758 ),
 ( #977, #13514, #26084, #38620, #7736, #29563, #13913, #14308, #26482, #7334, #4263, #29367, #7533 ) ),
 .UNSPECIFIED., .F., .F., .F.,
 ( 4, 3, 3, 3, 3, 3, 3, 3, 3, 3, 3, 3, 3, 3, 3, 3, 3, 3, 4 ),
 ( 4, 3, 3, 3, 4 ),
 ( 0.005001841298670386959, 0.005072013119329183903, 0.005142184939987979979, 0.005282528581305572998, 0.005563215863940759037, 0.006124590429211131982, 0.007247339559751877006, 0.008370088690292622896, 0.009492837820833367052, 0.01005421238610373913, 0.01061558695137411121, 0.01089627423400929725, 0.01117696151664448329, 0.01173833608191485710, 0.01286108521245560299, 0.01342245977772597507, 0.01370314706036116111, 0.01384349070167875326, 0.01398383434299634714 ),
 ( 0.000000000000000000, 0.2500000000000000000, 0.5000000000000000000, 0.7500000000000000000, 1.000000000000000000 ),
 .UNSPECIFIED. ) ;
#27555=CARTESIAN_POINT ( 'NONE',  ( 35.33522163555373652, -3.168965096689021266, 5.721313940429516798 ) ) ;
#27557=CARTESIAN_POINT ( 'NONE',  ( 88.23268491810016201, -0.7494148791586221492, 1.919551801057179263 ) ) ;
#27561=CARTESIAN_POINT ( 'NONE',  ( 37.18721867727772690, -2.963692379415546529, 6.000030405913790332 ) ) ;
#27562=CARTESIAN_POINT ( 'NONE',  ( 26.16082219273550891, -2.761323807819567655, 4.289427023688758389 ) ) ;
#27569=ORIENTED_EDGE ( 'NONE', *, *, #32206, .F. ) ;
#27574=CARTESIAN_POINT ( 'NONE',  ( 14.73610008032583885, -5.026708172105184502, 2.500480175786592874 ) ) ;
#27576=CARTESIAN_POINT ( 'NONE',  ( 22.49487306056245828, 2.478889120150127301, 4.939610370497833358 ) ) ;
#27577=CARTESIAN_POINT ( 'NONE',  ( 21.42227782476107123, 8.036706878627773776, -2.736079366572905514 ) ) ;
#27578=EDGE_LOOP ( 'NONE', ( #27176, #30260 ) ) ;
#27585=CARTESIAN_POINT ( 'NONE',  ( 85.58789802481842912, 2.221335288533847319, -3.332472240576935363 ) ) ;
#27588=CARTESIAN_POINT ( 'NONE',  ( 22.03209494260425316, 3.823468488147809374, -4.290561760811918646 ) ) ;
#27589=ORIENTED_EDGE ( 'NONE', *, *, #2049, .T. ) ;
#27591=CARTESIAN_POINT ( 'NONE',  ( 21.85643539959774273, 11.82890447862143546, -1.931159885854170311 ) ) ;
#27595=CARTESIAN_POINT ( 'NONE',  ( 85.03556247682649882, 2.841744791465048880, -1.219259102000758821 ) ) ;
#27600=LINE ( 'NONE', #37063, #40711 ) ;
#27601=CARTESIAN_POINT ( 'NONE',  ( 36.89739936142836996, -3.002644431800062463, -5.965129555963346597 ) ) ;
#27608=CARTESIAN_POINT ( 'NONE',  ( 36.63478925368298178, -2.000665574028761107, 5.847389373914565702 ) ) ;
#27621=CARTESIAN_POINT ( 'NONE',  ( 22.63992908519401581, 4.527459582470855004, 3.136945245597487553 ) ) ;
#27624=CARTESIAN_POINT ( 'NONE',  ( 21.94884155547715920, 5.596816108778505772, -3.078664276110406384 ) ) ;
#27627=CARTESIAN_POINT ( 'NONE',  ( 24.11813316538267316, 0.4652667653683164040, 5.100766439816002418 ) ) ;
#27628=CARTESIAN_POINT ( 'NONE',  ( 14.73630591169358617, -5.028744660188785076, -2.500462426279348893 ) ) ;
#27639=DIRECTION ( 'NONE',  ( 0.1542073060391599970, 0.000000000000000000, -0.9880385148181951571 ) ) ;
#27640=CARTESIAN_POINT ( 'NONE',  ( 32.93308485139972674, -2.920656968542761245, -5.757540729513444866 ) ) ;
#27645=CARTESIAN_POINT ( 'NONE',  ( 22.64608778944036516, 0.3051270519629841194, -6.453714758063171075 ) ) ;
#27649=CARTESIAN_POINT ( 'NONE',  ( 36.84739796419923863, -2.124053305941548953, -5.880516947223020985 ) ) ;
#27659=CARTESIAN_POINT ( 'NONE',  ( 14.75868911325587796, -5.145464069203309343, -2.500012630750525933 ) ) ;
#27660=CARTESIAN_POINT ( 'NONE',  ( 22.03785866058321119, 1.984797309109682217, -5.805693036113302341 ) ) ;
#27668=EDGE_CURVE ( 'NONE', #28242, #6497, #40316, .T. ) ;
#27671=CARTESIAN_POINT ( 'NONE',  ( -70.92837670882107659, -65.19654454972992141, 6.000000000000002665 ) ) ;
#27673=ORIENTED_EDGE ( 'NONE', *, *, #28157, .T. ) ;
#27674=CARTESIAN_POINT ( 'NONE',  ( 22.61684402008435768, 4.633385194857577716, 3.026614357573721215 ) ) ;
#27684=CARTESIAN_POINT ( 'NONE',  ( 21.85643539959780313, -7.722266916079949972, 9.821539774841749448 ) ) ;
#27686=CARTESIAN_POINT ( 'NONE',  ( -78.52360362737910293, 11.36405371355654736, 6.517260701712046078 ) ) ;
#27687=CARTESIAN_POINT ( 'NONE',  ( 35.65372115386870888, -3.750406728026652647, 5.582374933998859312 ) ) ;
#27690=CARTESIAN_POINT ( 'NONE',  ( 31.99016054316349056, -3.341357271039956611, -5.178217504156710227 ) ) ;
#27691=CARTESIAN_POINT ( 'NONE',  ( 23.38648856837436441, 3.560657187999370699, -3.090153159693794116 ) ) ;
#27693=CARTESIAN_POINT ( 'NONE',  ( 15.09522703660796239, 11.91064461445325229, 2.554458953684618283 ) ) ;
#27700=CARTESIAN_POINT ( 'NONE',  ( 19.29296610083087415, 12.44317219469094660, -2.499999999999999556 ) ) ;
#27702=CARTESIAN_POINT ( 'NONE',  ( 37.08720602107538866, -2.368560226880349173, -5.943858709518226036 ) ) ;
#27703=CARTESIAN_POINT ( 'NONE',  ( 25.75309628829585762, 2.097993264449613537, -4.157463482038479263 ) ) ;
#27705=CARTESIAN_POINT ( 'NONE',  ( -69.43806570890772889, -47.31353566070715999, 5.812001725005383257 ) ) ;
#27707=CARTESIAN_POINT ( 'NONE',  ( 34.38864450132898298, -1.330693349609932241, 5.573577685579110153 ) ) ;
#27710=CARTESIAN_POINT ( 'NONE',  ( 85.36258410344761671, 2.204690851838579047, 4.549306268726941660 ) ) ;
#27713=CARTESIAN_POINT ( 'NONE',  ( 35.92909550028735310, -2.111770154685527423, -5.814002319914921557 ) ) ;
#27715=EDGE_LOOP ( 'NONE', ( #4985, #18537, #7771, #22284 ) ) ;
#27718=EDGE_LOOP ( 'NONE', ( #19219, #20172, #19244, #25337, #2846, #39687, #16188, #21600 ) ) ;
#27724=DIRECTION ( 'NONE',  ( -0.000000000000000000, -1.000000000000000000, -0.000000000000000000 ) ) ;
#27731=FACE_OUTER_BOUND ( 'NONE', #2997, .T. ) ;
#27734=CARTESIAN_POINT ( 'NONE',  ( 23.42254319797303452, 3.705070095891317639, -3.277622970724664686 ) ) ;
#27738=CARTESIAN_POINT ( 'NONE',  ( 24.55145103709714505, -1.086933616027371263, 6.883468691731016165 ) ) ;
#27743=CARTESIAN_POINT ( 'NONE',  ( 87.24982552262115121, -1.326261458569501839, 4.881571762780114732 ) ) ;
#27747=CARTESIAN_POINT ( 'NONE',  ( -72.35147488751991318, -46.63281737808343053, 9.898294814228878025 ) ) ;
#27749=CARTESIAN_POINT ( 'NONE',  ( -61.24591834330252027, -23.80776546975053520, -2.500000000000000000 ) ) ;
#27750=CARTESIAN_POINT ( 'NONE',  ( 14.86430981739665746, -4.493068681216141336, -2.516462316360253748 ) ) ;
#27752=DIRECTION ( 'NONE',  ( 1.385724075720358314E-16, -1.000000000000000000, 0.000000000000000000 ) ) ;
#27754=CARTESIAN_POINT ( 'NONE',  ( 34.33173276390347439, -1.489116378852566980, 5.564695232538289460 ) ) ;
#27759=CARTESIAN_POINT ( 'NONE',  ( 36.13337973148855298, -1.529159196477766880, 5.642270371453538047 ) ) ;
#27760=CARTESIAN_POINT ( 'NONE',  ( 21.59288859382414572, -2.652561316991649765, 3.576490509687073160 ) ) ;
#27761=CARTESIAN_POINT ( 'NONE',  ( 17.57044049449111967, -3.218502976824792139, -2.911085957591616591 ) ) ;
#27763=CARTESIAN_POINT ( 'NONE',  ( 14.61802080322610919, 12.62870316934875881, -2.500000000000000000 ) ) ;
#27771=CARTESIAN_POINT ( 'NONE',  ( 22.04733053187323222, 2.939797654462655618, 4.949211021722255133 ) ) ;
#27772=CARTESIAN_POINT ( 'NONE',  ( 14.73664178711200101, 12.61985148690355985, 2.505541970458036616 ) ) ;
#27779=CARTESIAN_POINT ( 'NONE',  ( 87.04213330793400871, 0.5878691963681514920, -4.891134986362597914 ) ) ;
#27783=CARTESIAN_POINT ( 'NONE',  ( 23.26269754767185560, 3.142007143762405086, -3.939437242187847410 ) ) ;
#27785=CARTESIAN_POINT ( 'NONE',  ( -4.890026461918809630, -25.50263309590217276, 27.90461065042423527 ) ) ;
#27786=CARTESIAN_POINT ( 'NONE',  ( 21.85643539959777826, -4.218647804531223677, -15.78683364351815221 ) ) ;
#27790=CARTESIAN_POINT ( 'NONE',  ( 88.38542499104009664, -0.9209797785659445957, 1.969977704346236536 ) ) ;
#27791=CARTESIAN_POINT ( 'NONE',  ( 16.11725891507163766, 15.27317977277692052, -2.500000000000000000 ) ) ;
#27792=AXIS2_PLACEMENT_3D ( 'NONE', #33672, #26666, #10993 ) ;
#27796=CARTESIAN_POINT ( 'NONE',  ( 26.27633885242532585, -3.098738397173856018, 4.268606335983216482 ) ) ;
#27797=DIRECTION ( 'NONE',  ( 1.000000000000000000, 7.232507224765808510E-18, 0.000000000000000000 ) ) ;
#27798=EDGE_CURVE ( 'NONE', #14959, #3867, #35865, .T. ) ;
#27799=CARTESIAN_POINT ( 'NONE',  ( 29.13959756157474246, 0.4692356663346191059, -4.754336961950639484 ) ) ;
#27803=CARTESIAN_POINT ( 'NONE',  ( 21.81833114184418321, 5.350335711903964508, -3.566543258216577250 ) ) ;
#27806=CARTESIAN_POINT ( 'NONE',  ( 37.17273293948297663, -2.956732537645826220, 5.999804286280149945 ) ) ;
#27810=CARTESIAN_POINT ( 'NONE',  ( 88.19592634550657806, -0.7081259057544491142, 2.233392006332136859 ) ) ;
#27811=CARTESIAN_POINT ( 'NONE',  ( -71.86858480636978186, 0.9314695403570354415, -9.956036837141201801 ) ) ;
#27814=ORIENTED_EDGE ( 'NONE', *, *, #449, .T. ) ;
#27815=DIRECTION ( 'NONE',  ( 0.000000000000000000, 0.000000000000000000, -1.000000000000000000 ) ) ;
#27818=CARTESIAN_POINT ( 'NONE',  ( 23.42725932339659423, 3.763513707203086867, 3.172503157220333048 ) ) ;
#27824=B_SPLINE_CURVE_WITH_KNOTS ( 'NONE', 3,
 ( #21200, #36435, #40322, #11294, #33774, #8206, #39511, #20781, #5144, #27574, #33374, #11500, #17677, #5551, #14590, #11703, #33983, #24065 ),
 .UNSPECIFIED., .F., .F.,
 ( 4, 2, 2, 2, 2, 2, 2, 2, 4 ),
 ( -5.999999609784804829E-08, 8.963808126167891594E-05, 0.0001793361625194556759, 0.0003587323250350066208, 0.0005381284875505575657, 0.0006278265688083316557, 0.0006726756094372194055, 0.0006951001297516632262, 0.0007175246500661071553 ),
 .UNSPECIFIED. ) ;
#27840=CARTESIAN_POINT ( 'NONE',  ( 30.81316972100007590, -2.191302700533721115, -5.899179390191041428 ) ) ;
#27844=CARTESIAN_POINT ( 'NONE',  ( 26.67714935503705931, 0.9909774768816611568, -4.380117908427034301 ) ) ;
#27850=CARTESIAN_POINT ( 'NONE',  ( 36.70922304957898064, -3.420571215935285903, -5.875113064356194847 ) ) ;
#27856=CARTESIAN_POINT ( 'NONE',  ( -75.25715755557821751, 8.188700395369970408, 10.38624776870203981 ) ) ;
#27857=CARTESIAN_POINT ( 'NONE',  ( 86.59537683758360060, -0.3992097724244685342, -5.811584838773467432 ) ) ;
#27859=CARTESIAN_POINT ( 'NONE',  ( 25.38987815660813041, 2.286237158485121324, -4.080818507191673383 ) ) ;
#27875=CARTESIAN_POINT ( 'NONE',  ( 21.98910052706983365, 5.614098391567612367, 3.090586958385738825 ) ) ;
#27886=CARTESIAN_POINT ( 'NONE',  ( 22.75155763331752112, -5.137713618528696458, -6.528071535057289765 ) ) ;
#27888=CARTESIAN_POINT ( 'NONE',  ( -71.75673233877098767, 2.217010188227585665, 9.965676783907941427 ) ) ;
#27889=CARTESIAN_POINT ( 'NONE',  ( 34.29746155415688236, -3.857051845548268521, 5.268846866181171151 ) ) ;
#27891=VECTOR ( 'NONE', #13647, 1000.000000000000000 ) ;
#27894=CARTESIAN_POINT ( 'NONE',  ( 33.45155509882757627, -3.250653912085893715, -5.427322220725915969 ) ) ;
#27895=CARTESIAN_POINT ( 'NONE',  ( 34.79242720853928006, -3.835804077954089397, -5.376515837512373608 ) ) ;
#27898=CARTESIAN_POINT ( 'NONE',  ( 15.05256153508802086, 12.14757130736968449, 2.534552796716138978 ) ) ;
#27902=VECTOR ( 'NONE', #22054, 1000.000000000000000 ) ;
#27903=DIRECTION ( 'NONE',  ( -0.000000000000000000, -1.000000000000000000, -0.000000000000000000 ) ) ;
#27904=CARTESIAN_POINT ( 'NONE',  ( 23.11875216611918660, 0.3874244158500451674, -5.890943838375131136 ) ) ;
#27905=CARTESIAN_POINT ( 'NONE',  ( 30.30972199426953040, -3.799155601095605128, -4.460120920599953465 ) ) ;
#27906=CARTESIAN_POINT ( 'NONE',  ( 24.71566706424699689, 3.001517176038623447, -3.434326518345315105 ) ) ;
#27908=CARTESIAN_POINT ( 'NONE',  ( -69.42837670882107659, -47.21594255105944171, 5.809475019311132193 ) ) ;
#27910=CARTESIAN_POINT ( 'NONE',  ( 34.95690096516870682, -1.636465606770671100, 5.662267850096001531 ) ) ;
#27911=DIRECTION ( 'NONE',  ( 1.000000000000000000, 0.000000000000000000, 0.000000000000000000 ) ) ;
#27913=CARTESIAN_POINT ( 'NONE',  ( 88.80901725076027731, -1.591322664339660298, -1.862171775454326550 ) ) ;
#27914=CARTESIAN_POINT ( 'NONE',  ( 29.67925625648019405, 0.9272574953382407559, 4.669903954941619695 ) ) ;
#27915=CARTESIAN_POINT ( 'NONE',  ( 35.98288326577282703, -3.153944312834425556, -5.822397201580947979 ) ) ;
#27917=CARTESIAN_POINT ( 'NONE',  ( 24.58210053396808448, 2.978637365502128542, 3.574180794472539446 ) ) ;
#27925=VECTOR ( 'NONE', #9525, 1000.000000000000000 ) ;
#27931=ADVANCED_FACE ( 'NONE', ( #2293 ), #14819, .T. ) ;
#27932=CIRCLE ( 'NONE', #5574, 3.000000000000002665 ) ;
#27939=CARTESIAN_POINT ( 'NONE',  ( 22.40201758004466015, 4.861284111922041795, -3.110657656184960373 ) ) ;
#27941=DIRECTION ( 'NONE',  ( -1.000000000000000000, -7.232507224765808510E-18, 0.000000000000000000 ) ) ;
#27942=CARTESIAN_POINT ( 'NONE',  ( 24.54460225945253526, -1.054324096271329614, -6.891227800717186547 ) ) ;
#27943=CARTESIAN_POINT ( 'NONE',  ( -77.84099478799700478, -6.330046395677443982, -7.228837368596992441 ) ) ;
#27947=CARTESIAN_POINT ( 'NONE',  ( 87.06687503756165825, -0.7302844941506287935, -5.541598948305895611 ) ) ;
#27954=CARTESIAN_POINT ( 'NONE',  ( 14.92718052254917183, -5.911376862938025667, -2.518629130483756473 ) ) ;
#27955=CARTESIAN_POINT ( 'NONE',  ( 36.44585954531025607, -2.356780152367485393, -5.894655847126518466 ) ) ;
#27959=CARTESIAN_POINT ( 'NONE',  ( 36.44622604588383297, -2.355887491903832398, 5.894713048404869760 ) ) ;
#27962=CARTESIAN_POINT ( 'NONE',  ( 85.13880989351328310, 2.725772392624387308, 0.2960746283792183853 ) ) ;
#27966=CARTESIAN_POINT ( 'NONE',  ( 25.89546385390948657, -2.750212554045368130, 4.248011437199279428 ) ) ;
#27969=CARTESIAN_POINT ( 'NONE',  ( 27.33867765376834313, -4.445383502205745074, -3.667891126866987594 ) ) ;
#27971=ORIENTED_EDGE ( 'NONE', *, *, #2049, .F. ) ;
#27976=CARTESIAN_POINT ( 'NONE',  ( 23.82088032715813242, 2.765655670818042200, 4.014859125618367663 ) ) ;
#27977=CARTESIAN_POINT ( 'NONE',  ( 31.60216379219463789, 0.4244636512702888442, 4.640344443660871399 ) ) ;
#27979=EDGE_CURVE ( 'NONE', #36468, #9338, #4472, .T. ) ;
#27981=CIRCLE ( 'NONE', #33261, 6.000000000000002665 ) ;
#27984=CARTESIAN_POINT ( 'NONE',  ( -70.31448100068961082, 0.01729022305976556789, 5.969247584478902802 ) ) ;
#27985=CARTESIAN_POINT ( 'NONE',  ( 86.15668803663793085, 1.582443350855704978, -4.576617297167563159 ) ) ;
#27990=CARTESIAN_POINT ( 'NONE',  ( 22.23429677150355843, 3.418736078724165850, -4.405329081129731428 ) ) ;
#27992=DIRECTION ( 'NONE',  ( -0.000000000000000000, -0.000000000000000000, -1.000000000000000000 ) ) ;
#27994=CARTESIAN_POINT ( 'NONE',  ( 21.85643539959778892, -12.39743456692229628, -10.22857181343751520 ) ) ;
#27995=CARTESIAN_POINT ( 'NONE',  ( 16.10603109343461981, 15.28195951419911580, 3.145749391472286050 ) ) ;
#27997=CARTESIAN_POINT ( 'NONE',  ( 28.44383639013767962, -4.073698245608341040, -4.060485434070885802 ) ) ;
#28000=CARTESIAN_POINT ( 'NONE',  ( 87.15505355144220800, 0.4610318193416703680, -5.246243280819175681 ) ) ;
#28004=CARTESIAN_POINT ( 'NONE',  ( 21.53101133388948085, -2.979226547270804382, 3.510723884023187136 ) ) ;
#28005=CARTESIAN_POINT ( 'NONE',  ( 25.06775773363566984, 3.218135757308234091, 2.425511022795127758 ) ) ;
#28006=CARTESIAN_POINT ( 'NONE',  ( 22.97036411035692538, 2.781245753741529825, -3.791478878413661047 ) ) ;
#28008=CARTESIAN_POINT ( 'NONE',  ( 21.78047190118184773, 5.616103730238553027, 3.473245441588607374 ) ) ;
#28013=ORIENTED_EDGE ( 'NONE', *, *, #17895, .T. ) ;
#28014=CARTESIAN_POINT ( 'NONE',  ( 37.00785681416889616, -3.244586891125645245, 5.947379696897557189 ) ) ;
#28018=CARTESIAN_POINT ( 'NONE',  ( 87.65927558969256950, -2.189574935990458382, -2.847504520461086486 ) ) ;
#28023=CARTESIAN_POINT ( 'NONE',  ( -72.11214491845440477, -0.3118290589227806775, -9.931028944812110737 ) ) ;
#28024=CARTESIAN_POINT ( 'NONE',  ( 16.66455774270143664, 9.373215685664842312, 2.807305288237325502 ) ) ;
#28029=CARTESIAN_POINT ( 'NONE',  ( 22.40535950346533056, 4.849712323715404061, 3.119056588188622303 ) ) ;
#28033=EDGE_CURVE ( 'NONE', #18658, #36134, #26089, .T. ) ;
#28039=CARTESIAN_POINT ( 'NONE',  ( 15.16793238289938373, 11.41091229596485057, -2.573720704819107308 ) ) ;
#28047=FACE_OUTER_BOUND ( 'NONE', #26376, .T. ) ;
#28048=CARTESIAN_POINT ( 'NONE',  ( 31.44014676667174157, -3.103618331322294921, 5.406754918213918515 ) ) ;
#28049=VECTOR ( 'NONE', #32212, 1000.000000000000114 ) ;
#28050=( BOUNDED_SURFACE ( )  B_SPLINE_SURFACE ( 3, 2, ( 
 ( #30458, #37232, #30879 ),
 ( #30673, #30051, #27763 ),
 ( #15208, #8814, #8613 ),
 ( #36831, #20985, #33563 ) ),
 .UNSPECIFIED., .F., .F., .T. ) 
 B_SPLINE_SURFACE_WITH_KNOTS ( ( 4, 4 ),
 ( 3, 3 ),
 ( 0.000000000000000000, 0.0008754244208249594870 ),
 ( 0.000000000000000000, 1.000000000000000000 ),
 .UNSPECIFIED. ) 
 GEOMETRIC_REPRESENTATION_ITEM ( )  RATIONAL_B_SPLINE_SURFACE ( (
 ( 1.000000000000000000, 0.9970051441236976730, 1.000000000000000000),
 ( 1.000000000000000000, 0.9987001331027346440, 1.000000000000000000),
 ( 1.000000000000000000, 0.9999578578056158573, 1.000000000000000000),
 ( 1.000000000000000000, 1.000000000000000000, 1.000000000000000000) ) ) 
 REPRESENTATION_ITEM ( '' )  SURFACE ( )  );
#28054=CARTESIAN_POINT ( 'NONE',  ( 25.35178780325773218, 0.7567565456469654839, -4.605944304649653986 ) ) ;
#28057=DIRECTION ( 'NONE',  ( 0.000000000000000000, 0.000000000000000000, 1.000000000000000000 ) ) ;
#28060=CARTESIAN_POINT ( 'NONE',  ( 33.66549675240646167, -3.596112717151957572, -5.375207407732099263 ) ) ;
#28068=CARTESIAN_POINT ( 'NONE',  ( 21.47057743101996152, 7.821696842773389058, 2.778301367339317984 ) ) ;
#28070=ORIENTED_EDGE ( 'NONE', *, *, #10593, .F. ) ;
#28078=VECTOR ( 'NONE', #35374, 1000.000000000000000 ) ;
#28083=CARTESIAN_POINT ( 'NONE',  ( 23.44311166670899027, 3.801244202611772760, 3.077376805319965936 ) ) ;
#28084=EDGE_CURVE ( 'NONE', #24333, #7, #7337, .T. ) ;
#28089=CARTESIAN_POINT ( 'NONE',  ( 24.12062818113409435, 0.5588176674967194613, 5.091530623029829172 ) ) ;
#28095=CARTESIAN_POINT ( 'NONE',  ( 21.85643539959777115, 3.923092093126210322, -11.21220060410217734 ) ) ;
#28098=CARTESIAN_POINT ( 'NONE',  ( -73.12593961609827886, 4.566678402415828231, 9.815056785847646736 ) ) ;
#28099=CARTESIAN_POINT ( 'NONE',  ( 37.19253098679411806, -2.880311961911129703, 5.999669043459923579 ) ) ;
#28104=CARTESIAN_POINT ( 'NONE',  ( 36.71933413544295632, -3.459668038622879305, -5.860247842560236009 ) ) ;
#28106=CARTESIAN_POINT ( 'NONE',  ( 14.72178876176509199, 13.26025408016186802, 2.500108498187831430 ) ) ;
#28109=PRODUCT_DEFINITION_FORMATION_WITH_SPECIFIED_SOURCE ( 'ANY', '', #11783, .NOT_KNOWN. ) ;
#28113=CARTESIAN_POINT ( 'NONE',  ( 18.47097006516344564, 13.26508273762688717, -2.500000000000000000 ) ) ;
#28114=CARTESIAN_POINT ( 'NONE',  ( 25.22036471513533584, 0.8962270189713842372, -4.613828365072303761 ) ) ;
#28116=CARTESIAN_POINT ( 'NONE',  ( 24.56079138214657931, 2.730512922303396817, -3.879043415943517203 ) ) ;
#28120=CARTESIAN_POINT ( 'NONE',  ( 21.35934345986309069, 3.587023842369657878, 3.540040143219671531 ) ) ;
#28122=CARTESIAN_POINT ( 'NONE',  ( 88.36353413610991936, -2.347965962749813063, -0.8794284646705250452 ) ) ;
#28123=CARTESIAN_POINT ( 'NONE',  ( 35.48404000816106674, -1.920476918020975754, -5.744540646660859728 ) ) ;
#28125=VECTOR ( 'NONE', #11004, 1000.000000000000000 ) ;
#28126=ORIENTED_EDGE ( 'NONE', *, *, #8300, .T. ) ;
#28127=CARTESIAN_POINT ( 'NONE',  ( 25.60585682308668964, 2.174458409923740287, 4.126442313751081059 ) ) ;
#28129=CARTESIAN_POINT ( 'NONE',  ( -70.92837670882201451, -21.78299143689573469, 6.000000000001379341 ) ) ;
#28139=ORIENTED_EDGE ( 'NONE', *, *, #9483, .F. ) ;
#28142=CARTESIAN_POINT ( 'NONE',  ( 23.06594672544511582, -8.086844732617873177, 2.500000000000001332 ) ) ;
#28144=CARTESIAN_POINT ( 'NONE',  ( 33.89863206464382017, -5.476329442118064605, -0.1430302926928115892 ) ) ;
#28145=CARTESIAN_POINT ( 'NONE',  ( 22.61884710626975092, 4.600495562082832279, -3.071470106280676404 ) ) ;
#28148=CARTESIAN_POINT ( 'NONE',  ( 24.23947115566313926, 0.8503125907183233245, 6.739520400040675874 ) ) ;
#28149=CARTESIAN_POINT ( 'NONE',  ( -75.99771073292856727, -5.502405136523671025, -8.621866671386070990 ) ) ;
#28152=CARTESIAN_POINT ( 'NONE',  ( 84.32222422711384979, 2.914578286995431977, 1.930349914595605343 ) ) ;
#28153=CARTESIAN_POINT ( 'NONE',  ( 14.96986543946197479, 12.33094088818544698, 2.523832330313138250 ) ) ;
#28157=EDGE_CURVE ( 'NONE', #12484, #24796, #13916, .T. ) ;
#28159=CARTESIAN_POINT ( 'NONE',  ( 31.38401102386968589, -3.643146459872906195, -4.878133479856779253 ) ) ;
#28160=CARTESIAN_POINT ( 'NONE',  ( 34.92827436638099670, -1.713443684080601992, -5.657799977018275861 ) ) ;
#28163=CARTESIAN_POINT ( 'NONE',  ( 29.10048579223744980, 0.3561570061246891461, 4.748232624423857295 ) ) ;
#28165=CARTESIAN_POINT ( 'NONE',  ( 86.80434382515846892, 0.8549656295913086179, -5.002690157204635391 ) ) ;
#28169=CARTESIAN_POINT ( 'NONE',  ( -69.61748845350692250, -47.87187071230540170, 9.913994275702524561 ) ) ;
#28172=CARTESIAN_POINT ( 'NONE',  ( 25.89164700572842293, -5.102322433750814845, -3.184945769527233850 ) ) ;
#28174=CARTESIAN_POINT ( 'NONE',  ( -80.90861860399088812, 11.45717611192839591, 0.6283086135788885640 ) ) ;
#28175=EDGE_LOOP ( 'NONE', ( #1228, #27343, #3060 ) ) ;
#28176=ADVANCED_FACE ( 'NONE', ( #26488 ), #610, .F. ) ;
#28178=CARTESIAN_POINT ( 'NONE',  ( 35.63425396194121220, -3.169062201350007157, 5.767985167086449927 ) ) ;
#28180=CARTESIAN_POINT ( 'NONE',  ( 22.68890514319382135, 2.782549721596407455, 4.545382121805146447 ) ) ;
#28181=DIRECTION ( 'NONE',  ( 1.000000000000000000, 8.966158204770716457E-16, 0.000000000000000000 ) ) ;
#28190=CARTESIAN_POINT ( 'NONE',  ( 24.18717966629001737, 2.859004644576334631, -3.837239278320205838 ) ) ;
#28191=EDGE_LOOP ( 'NONE', ( #23911, #21135, #29154, #1715 ) ) ;
#28193=CARTESIAN_POINT ( 'NONE',  ( 21.85643539959776760, 10.44946649885084966, 7.640826779728119078 ) ) ;
#28198=CARTESIAN_POINT ( 'NONE',  ( 85.12050554930138446, 2.746332700819607453, -1.966258668667607123 ) ) ;
#28199=EDGE_LOOP ( 'NONE', ( #30677, #4735, #24313, #20429 ) ) ;
#28201=CARTESIAN_POINT ( 'NONE',  ( 18.27257696809985177, -3.066843069763234286, 3.029022186580533127 ) ) ;
#28203=CARTESIAN_POINT ( 'NONE',  ( 29.10272931528550799, 0.3625471829554103298, -4.748582780455301133 ) ) ;
#28204=CARTESIAN_POINT ( 'NONE',  ( -12.99139449055068596, 10.37661300689600097, 2.500000000000000000 ) ) ;
#28208=EDGE_CURVE ( 'NONE', #23822, #25264, #24405, .T. ) ;
#28212=CARTESIAN_POINT ( 'NONE',  ( 25.73261264963540995, 2.635811757010384504, 3.523854048240384618 ) ) ;
#28216=CARTESIAN_POINT ( 'NONE',  ( 87.69516453960757474, -2.233259521322014329, -2.657756335895389288 ) ) ;
#28221=DIRECTION ( 'NONE',  ( 1.000000000000000000, 0.000000000000000000, 0.000000000000000000 ) ) ;
#28227=EDGE_LOOP ( 'NONE', ( #34255, #24342 ) ) ;
#28228=CARTESIAN_POINT ( 'NONE',  ( 22.39794005767262064, 4.875138222190518178, 3.100870480539395402 ) ) ;
#28239=CARTESIAN_POINT ( 'NONE',  ( 16.69750073655492528, 9.540205430295099376, -2.812446839157479506 ) ) ;
#28242=VERTEX_POINT ( 'NONE', #31207 ) ;
#28248=DIRECTION ( 'NONE',  ( 0.000000000000000000, 0.000000000000000000, -1.000000000000000000 ) ) ;
#28250=CARTESIAN_POINT ( 'NONE',  ( 30.28570682881508702, -1.586248365680131167, -6.023113166707004140 ) ) ;
#28252=CARTESIAN_POINT ( 'NONE',  ( 30.10852511091080430, -6.281056253467228956, 2.499999999999994671 ) ) ;
#28254=CARTESIAN_POINT ( 'NONE',  ( 23.59795352485724962, 0.4334124443017954853, -5.517309192317882527 ) ) ;
#28262=CARTESIAN_POINT ( 'NONE',  ( 20.85070742889012152, 4.522926380425460025, -2.940039916530858832 ) ) ;
#28264=CARTESIAN_POINT ( 'NONE',  ( -17.69482985384421880, -42.37473357531882101, 2.500000000000000000 ) ) ;
#28267=EDGE_CURVE ( 'NONE', #35921, #17878, #14258, .T. ) ;
#28269=CARTESIAN_POINT ( 'NONE',  ( 22.56436664557526584, -9.049820346388647962, 2.499999999999999112 ) ) ;
#28285=CARTESIAN_POINT ( 'NONE',  ( 23.14409375757164256, 4.053802376405804431, 3.062998084521663333 ) ) ;
#28291=CARTESIAN_POINT ( 'NONE',  ( 23.62020001075898179, 0.4737404876348103588, 5.490607732800076413 ) ) ;
#28295=ORIENTED_EDGE ( 'NONE', *, *, #117, .T. ) ;
#28300=VERTEX_POINT ( 'NONE', #8741 ) ;
#28301=CARTESIAN_POINT ( 'NONE',  ( 21.85643539959777470, -4.742028430345498258, -11.91557605213902882 ) ) ;
#28304=CARTESIAN_POINT ( 'NONE',  ( -77.44400633864859174, 9.722113372229207684, 9.166479153956517578 ) ) ;
#28305=CARTESIAN_POINT ( 'NONE',  ( 37.04442315954803178, -3.197375157205383456, 5.958390354492890673 ) ) ;
#28307=DIRECTION ( 'NONE',  ( -0.000000000000000000, 1.000000000000000000, -0.000000000000000000 ) ) ;
#28308=EDGE_LOOP ( 'NONE', ( #17024, #22325, #6319, #27814 ) ) ;
#28310=CARTESIAN_POINT ( 'NONE',  ( 30.68983369444830345, -3.022615581088325509, -4.996288803099273146 ) ) ;
#28311=CARTESIAN_POINT ( 'NONE',  ( 33.94754086493713174, -0.4854118941598933867, -5.118189633504289127 ) ) ;
#28314=CARTESIAN_POINT ( 'NONE',  ( 19.11796579935018059, 7.216354979127149960, 3.190218951375439982 ) ) ;
#28316=CARTESIAN_POINT ( 'NONE',  ( 29.63236135128273929, -3.802766571116140248, 4.424495427163341432 ) ) ;
#28322=CARTESIAN_POINT ( 'NONE',  ( 25.02876953629550272, 1.120990461282832751, -4.601145122132357379 ) ) ;
#28323=CARTESIAN_POINT ( 'NONE',  ( 32.15421574055506682, -3.772606034914804951, -4.832894874862167178 ) ) ;
#28325=CARTESIAN_POINT ( 'NONE',  ( 26.61849259059863826, 1.625058386879766559, -4.334342491016723642 ) ) ;
#28328=CARTESIAN_POINT ( 'NONE',  ( 36.98982775529254496, -2.542815128719615014, 5.977429629229624730 ) ) ;
#28330=CARTESIAN_POINT ( 'NONE',  ( 87.91375683397511409, -1.031045523906674033, -4.794500835981626352 ) ) ;
#28334=CARTESIAN_POINT ( 'NONE',  ( 25.35519752494395362, 2.304653593253668031, 4.072349217575649938 ) ) ;
#28336=DIRECTION ( 'NONE',  ( 0.9999026450364576490, 0.01395351027862084051, 0.000000000000000000 ) ) ;
#28339=CARTESIAN_POINT ( 'NONE',  ( 0.000000000000000000, 13.37661300689600097, 2.500000000000000000 ) ) ;
#28340=DIRECTION ( 'NONE',  ( 0.000000000000000000, -0.000000000000000000, -1.000000000000000000 ) ) ;
#28343=CARTESIAN_POINT ( 'NONE',  ( -70.92837670882107659, -23.80776546975053165, 0.000000000000000000 ) ) ;
#28345=CARTESIAN_POINT ( 'NONE',  ( 14.74516149782244057, 13.12656125137344532, 2.499999999999999556 ) ) ;
#28353=CARTESIAN_POINT ( 'NONE',  ( 11.29080664838498649, 1.564594260697056104E-15, 6.000000000000000000 ) ) ;
#28354=CARTESIAN_POINT ( 'NONE',  ( 22.38437366705409204, 4.924138827339338498, -3.063762403727182448 ) ) ;
#28357=B_SPLINE_CURVE_WITH_KNOTS ( 'NONE', 3,
 ( #5306, #39265, #39060, #4511, #11056, #20527 ),
 .UNSPECIFIED., .F., .F.,
 ( 4, 2, 4 ),
 ( 8.484391014525137476E-05, 0.003152276965141869499, 0.006219710020138487054 ),
 .UNSPECIFIED. ) ;
#28360=CARTESIAN_POINT ( 'NONE',  ( -76.83524845872202036, -4.539336671474099028, -9.585163668414178773 ) ) ;
#28361=CARTESIAN_POINT ( 'NONE',  ( -70.92837670882107659, -23.80776546975053520, 0.000000000000000000 ) ) ;
#28363=CARTESIAN_POINT ( 'NONE',  ( 87.88829317789571860, -2.466143857431153830, 1.215092630805642671 ) ) ;
#28367=CARTESIAN_POINT ( 'NONE',  ( 25.01357312920399778, 3.324376023134533842, -1.959542026491533750 ) ) ;
#28373=CARTESIAN_POINT ( 'NONE',  ( 30.19003827612802482, -2.952522945788203845, 4.918283640461378781 ) ) ;
#28376=CARTESIAN_POINT ( 'NONE',  ( 34.77313873784321885, -3.161490297579837350, 5.633587310215530053 ) ) ;
#28377=CARTESIAN_POINT ( 'NONE',  ( 87.92727933775610438, -0.4063688358931643041, -3.816426586085390760 ) ) ;
#28380=CARTESIAN_POINT ( 'NONE',  ( -4.444218661349752963, -35.94265729135299381, -6.000000000000000000 ) ) ;
#28386=CARTESIAN_POINT ( 'NONE',  ( -79.57508400964319151, -6.640697488684422112, 5.040913395559038612 ) ) ;
#28390=CARTESIAN_POINT ( 'NONE',  ( 24.75830837035764276, 3.019210359990082804, 3.350572556515618583 ) ) ;
#28392=CARTESIAN_POINT ( 'NONE',  ( 25.61003942877132289, 2.172251185455080780, 4.127339093466678044 ) ) ;
#28395=ORIENTED_EDGE ( 'NONE', *, *, #8811, .T. ) ;
#28403=CARTESIAN_POINT ( 'NONE',  ( 22.19554510023723637, 4.144875652714271830, -3.913740728431892801 ) ) ;
#28405=CARTESIAN_POINT ( 'NONE',  ( 21.85643539959774984, 10.28856666709980594, -7.862822601098399034 ) ) ;
#28410=CARTESIAN_POINT ( 'NONE',  ( 87.09859342968812257, 0.5244505078549105415, -5.068689133590885909 ) ) ;
#28413=LINE ( 'NONE', #12759, #9717 ) ;
#28414=VERTEX_POINT ( 'NONE', #7095 ) ;
#28415=CARTESIAN_POINT ( 'NONE',  ( 19.70671233036541281, -2.908903325760366698, 3.265966001044424249 ) ) ;
#28417=CARTESIAN_POINT ( 'NONE',  ( 35.78597716193907274, -3.162283487670411120, -5.791665241885592508 ) ) ;
#28419=CARTESIAN_POINT ( 'NONE',  ( -4.890026461918814071, -8.228598103685714525E-16, 6.000000000000000000 ) ) ;
#28424=CARTESIAN_POINT ( 'NONE',  ( 29.47104931226115099, -2.981108624964739828, 4.806068023836186143 ) ) ;
#28427=CARTESIAN_POINT ( 'NONE',  ( 36.71885878822434535, -3.457450448323470038, 5.861098606071526440 ) ) ;
#28432=CARTESIAN_POINT ( 'NONE',  ( 87.86569408387285307, -0.3371933557188040997, -3.487338236652987700 ) ) ;
#28436=ORIENTED_EDGE ( 'NONE', *, *, #4123, .F. ) ;
#28439=EDGE_LOOP ( 'NONE', ( #15613, #38444, #23831, #15219 ) ) ;
#28440=CARTESIAN_POINT ( 'NONE',  ( 23.99719617098446989, 3.301072601594968070, 3.381232105112813358 ) ) ;
#28445=ORIENTED_EDGE ( 'NONE', *, *, #14099, .F. ) ;
#28447=CARTESIAN_POINT ( 'NONE',  ( -71.59377001835473209, -45.76911956692035943, 5.963683625267878874 ) ) ;
#28449=CARTESIAN_POINT ( 'NONE',  ( 15.09416660562139789, 11.91275931974590030, -2.554301580912084368 ) ) ;
#28456=FACE_OUTER_BOUND ( 'NONE', #34958, .T. ) ;
#28457=DIRECTION ( 'NONE',  ( 0.000000000000000000, -0.000000000000000000, -1.000000000000000000 ) ) ;
#28460=CARTESIAN_POINT ( 'NONE',  ( 16.92333500577657190, 7.515569495004324807, 3.484773800360644991 ) ) ;
#28461=CARTESIAN_POINT ( 'NONE',  ( 28.22557690513166762, 1.384627073958520249, -4.541740331631825001 ) ) ;
#28462=DIRECTION ( 'NONE',  ( 0.000000000000000000, -0.000000000000000000, 1.000000000000000000 ) ) ;
#28470=CARTESIAN_POINT ( 'NONE',  ( 36.15893501698462842, -3.359997738205348750, -5.843264819365881380 ) ) ;
#28473=CARTESIAN_POINT ( 'NONE',  ( 21.50460961888511946, -2.679762898963643281, -3.562712440612756826 ) ) ;
#28475=CARTESIAN_POINT ( 'NONE',  ( -77.49308833732668234, 9.745258916933323690, 9.129529565702688032 ) ) ;
#28476=CIRCLE ( 'NONE', #25189, 12.73502530973474300 ) ;
#28479=CARTESIAN_POINT ( 'NONE',  ( 31.33294556979534917, -2.944313455537491464, 5.096661964955516488 ) ) ;
#28481=B_SPLINE_CURVE_WITH_KNOTS ( 'NONE', 3,
 ( #31625, #5894, #3451, #5686, #18229, #34328, #2624, #15143, #27702, #40255, #12041, #15349, #18432, #31020, #2828, #40449, #12258, #24832, #37377, #9173, #21745, #6098, #948, #3645, #35340, #28734, #28939, #25849, #13082, #29141, #22969, #548, #22773, #32249, #4045, #19265, #10187, #35533, #16169, #13483, #7110, #13278, #3850, #25644, #19671, #742, #38384, #6715, #26057, #34937, #16560, #31831, #38588, #10394, #38187, #22370, #9990, #22569, #35137, #6911, #32042, #19469, #16368, #14368, #14562, #11881, #18063 ),
 .UNSPECIFIED., .F., .F.,
 ( 4, 2, 1, 1, 2, 2, 2, 1, 2, 2, 1, 2, 1, 2, 2, 1, 2, 1, 1, 2, 2, 1, 1, 2, 2, 1, 1, 2, 2, 1, 1, 2, 2, 2, 1, 1, 2, 2, 1, 1, 1, 2, 4 ),
 ( 0.1786650602234007013, 0.1800047485722283680, 0.1813444369210560347, 0.1840238136187113960, 0.1893825670140220629, 0.2001000738046433691, 0.2054588271999540083, 0.2067985155487815918, 0.2074683597231953835, 0.2081382038976091753, 0.2108175805952658133, 0.2215350873858937530, 0.2268938407812077229, 0.2295732174788646940, 0.2322525941765216650, 0.2429701009671495771, 0.2644051145484054288, 0.2751226213390333131, 0.2804813747343473107, 0.2811512189087614910, 0.2818210630831757268, 0.2831607514320052532, 0.2858401281296641949, 0.3072751417109392813, 0.3501451688734893430, 0.3715801824547648735, 0.3822976892454029718, 0.3836373775942326647, 0.3849770659430624686, 0.3876564426407219655, 0.3930151960360420138, 0.4358852231986006798, 0.5216252775237169015, 0.5644953046862750679, 0.5859303182675540400, 0.5886096949652139809, 0.5892795391396290494, 0.5899493833140440069, 0.5912890716628744769, 0.5966478250581968013, 0.6073653318488412278, 0.6931053861739944200, 0.8645854948243009153 ),
 .UNSPECIFIED. ) ;
#28485=VERTEX_POINT ( 'NONE', #38371 ) ;
#28488=CARTESIAN_POINT ( 'NONE',  ( 24.19994416937476700, 2.844775240750135215, 3.845692126280272571 ) ) ;
#28493=CARTESIAN_POINT ( 'NONE',  ( 21.71163078881388486, 6.331898811992721754, 3.191961573981963340 ) ) ;
#28497=ORIENTED_EDGE ( 'NONE', *, *, #19028, .T. ) ;
#28499=CARTESIAN_POINT ( 'NONE',  ( 22.69308311670009815, 0.3336789988226459558, 6.387223081350540177 ) ) ;
#28509=CARTESIAN_POINT ( 'NONE',  ( 25.50874925706157725, -4.568791516319697266, 1.869930813790659618 ) ) ;
#28511=CARTESIAN_POINT ( 'NONE',  ( -71.81805169721867799, 3.553745898376941437, 9.960391718072360234 ) ) ;
#28512=CARTESIAN_POINT ( 'NONE',  ( 23.04769018874944919, 0.3307018522552950812, -5.968051205461429198 ) ) ;
#28518=CARTESIAN_POINT ( 'NONE',  ( 35.83241067984241113, -3.730005543395272571, -5.623145078173256373 ) ) ;
#28520=DIRECTION ( 'NONE',  ( 1.682730792515357087E-16, -1.000000000000000000, 0.000000000000000000 ) ) ;
#28525=CARTESIAN_POINT ( 'NONE',  ( -72.84815947045233031, 2.429809908889422498, 10.96147798754374669 ) ) ;
#28529=CARTESIAN_POINT ( 'NONE',  ( 10.58508780786439374, 19.59913305159139441, 2.500000000000000000 ) ) ;
#28530=CARTESIAN_POINT ( 'NONE',  ( 11.29080664838498649, 1.564594260697056104E-15, -2.500000000000000000 ) ) ;
#28535=CARTESIAN_POINT ( 'NONE',  ( 87.67494654488285732, -1.518266458920173312, 4.408571129606221994 ) ) ;
#28537=EDGE_LOOP ( 'NONE', ( #9793, #33587, #42, #17751 ) ) ;
#28538=CARTESIAN_POINT ( 'NONE',  ( 24.52463446364352251, 2.971563934966741094, 3.617821987212675783 ) ) ;
#28540=EDGE_CURVE ( 'NONE', #15683, #25264, #7070, .T. ) ;
#28545=CARTESIAN_POINT ( 'NONE',  ( -12.99139449055068241, -10.90558813203967148, 6.000000000000000000 ) ) ;
#28560=CARTESIAN_POINT ( 'NONE',  ( 27.68079990455899875, -4.321696173663788443, 3.781977261579025917 ) ) ;
#28563=CARTESIAN_POINT ( 'NONE',  ( 22.20314648110986866, 5.198427163008500607, -3.120655278281623257 ) ) ;
#28570=CARTESIAN_POINT ( 'NONE',  ( -80.20246960484742260, -5.670552041663467158, -3.761216877785253931 ) ) ;
#28574=CARTESIAN_POINT ( 'NONE',  ( 86.71282820137585645, -0.9518751250403653108, -5.452277641718156431 ) ) ;
#28578=CARTESIAN_POINT ( 'NONE',  ( 24.91801205947951559, 3.522942266573565018, -0.6749513148134329565 ) ) ;
#28584=CARTESIAN_POINT ( 'NONE',  ( 33.68717198159223614, -3.103543658905335345, 5.464095933698846608 ) ) ;
#28586=VECTOR ( 'NONE', #784, 1000.000000000000000 ) ;
#28587=CARTESIAN_POINT ( 'NONE',  ( 85.29288036551089647, 2.552713125850948117, 2.517437320556888736 ) ) ;
#28590=CARTESIAN_POINT ( 'NONE',  ( -62.14171895907916365, -49.48408358960642062, 4.951123000344127334 ) ) ;
#28591=CARTESIAN_POINT ( 'NONE',  ( -70.53845072783826708, -45.66527594205425089, 9.992858605650345893 ) ) ;
#28592=CARTESIAN_POINT ( 'NONE',  ( 21.67760900250310030, 6.625191744556888196, -3.088480972488703458 ) ) ;
#28597=CARTESIAN_POINT ( 'NONE',  ( -77.44913293113614827, -6.200972306469667572, 7.584227517916080963 ) ) ;
#28602=CARTESIAN_POINT ( 'NONE',  ( 22.53775728690858315, 1.439289773552580254, 5.787755947322271055 ) ) ;
#28609=CARTESIAN_POINT ( 'NONE',  ( 85.70158270174225379, 2.093639263612781409, 3.671950081750952055 ) ) ;
#28614=CARTESIAN_POINT ( 'NONE',  ( 22.01308812227411593, 4.306436655154639581, -3.976313850738264044 ) ) ;
#28617=CARTESIAN_POINT ( 'NONE',  ( 21.85643539959778181, 10.07385928288181987, 4.538892979079195200 ) ) ;
#28625=CARTESIAN_POINT ( 'NONE',  ( 84.90669483503786807, 2.936226605105188625, 1.856525974524364297 ) ) ;
#28626=VERTEX_POINT ( 'NONE', #17548 ) ;
#28629=CARTESIAN_POINT ( 'NONE',  ( 14.77909459087315724, -5.590190921940234148, 2.503920376596091124 ) ) ;
#28630=CARTESIAN_POINT ( 'NONE',  ( 20.42596845097466129, 3.670375344256894934, -3.394364399325110693 ) ) ;
#28632=CARTESIAN_POINT ( 'NONE',  ( -72.84815947045271400, 2.214050502457695746, 10.96147798754371472 ) ) ;
#28635=CARTESIAN_POINT ( 'NONE',  ( 32.01160973108229513, -3.695318852608926008, 4.882771644002913192 ) ) ;
#28638=CARTESIAN_POINT ( 'NONE',  ( 21.73770031614145992, 4.234352576155473002, 2.806692369165114442 ) ) ;
#28642=VECTOR ( 'NONE', #36277, 1000.000000000000000 ) ;
#28643=CARTESIAN_POINT ( 'NONE',  ( 87.73404314631468992, -0.1893167741230248335, -3.839138754766225237 ) ) ;
#28650=ORIENTED_EDGE ( 'NONE', *, *, #2019, .F. ) ;
#28651=AXIS2_PLACEMENT_3D ( 'NONE', #11568, #1945, #39798 ) ;
#28656=ORIENTED_EDGE ( 'NONE', *, *, #1562, .F. ) ;
#28661=CARTESIAN_POINT ( 'NONE',  ( 15.23622953457498497, 11.45049469319151214, -2.584380127111126413 ) ) ;
#28666=VERTEX_POINT ( 'NONE', #17150 ) ;
#28667=CARTESIAN_POINT ( 'NONE',  ( 16.11725891508299924, 15.27317977276803873, 2.500000000000000000 ) ) ;
#28671=CARTESIAN_POINT ( 'NONE',  ( 16.54830199238246990, 9.917958269357011858, 2.500000000000051514 ) ) ;
#28672=CARTESIAN_POINT ( 'NONE',  ( 30.28570682881508702, -1.586248365680131167, -6.023113166707004140 ) ) ;
#28680=CARTESIAN_POINT ( 'NONE',  ( 23.23260763512989158, 3.379986173245406178, -3.619755483646863503 ) ) ;
#28686=CARTESIAN_POINT ( 'NONE',  ( 28.66920249112477848, -4.024975064351027143, -4.110187144531254333 ) ) ;
#28688=DIRECTION ( 'NONE',  ( -1.000000000000000000, 0.000000000000000000, 0.000000000000000000 ) ) ;
#28690=DIRECTION ( 'NONE',  ( 0.000000000000000000, -0.000000000000000000, -1.000000000000000000 ) ) ;
#28692=ADVANCED_FACE ( 'NONE', ( #33452 ), #17754, .T. ) ;
#28695=CARTESIAN_POINT ( 'NONE',  ( 30.81211655921321935, -3.351903339995823128, 4.959630491910277605 ) ) ;
#28696=CARTESIAN_POINT ( 'NONE',  ( 22.03914767488266691, 3.561355022793854630, 4.473374508569111896 ) ) ;
#28705=ORIENTED_EDGE ( 'NONE', *, *, #14972, .F. ) ;
#28707=CARTESIAN_POINT ( 'NONE',  ( 24.71218170711417272, 0.6478519780817281193, 4.786773077597882953 ) ) ;
#28716=CARTESIAN_POINT ( 'NONE',  ( 22.31703049540045924, 6.264542857755036387, 0.009563241200241559548 ) ) ;
#28719=CARTESIAN_POINT ( 'NONE',  ( -74.87858385344040357, 7.803706760580113588, 9.233433073997890261 ) ) ;
#28720=CARTESIAN_POINT ( 'NONE',  ( 22.60587387393427150, 0.2865033312617634720, -6.509150990572208251 ) ) ;
#28725=CARTESIAN_POINT ( 'NONE',  ( 28.74843373310636707, -3.747644898664072688, -4.540536534472360941 ) ) ;
#28726=CARTESIAN_POINT ( 'NONE',  ( 37.10943087117655637, -2.404357389779887555, -5.951804628107819184 ) ) ;
#28727=DIRECTION ( 'NONE',  ( 1.000000000000000000, 1.682730792515357087E-16, -0.000000000000000000 ) ) ;
#28728=CARTESIAN_POINT ( 'NONE',  ( 16.37363295469527102, 9.900998059239732640, 2.761899439026373582 ) ) ;
#28730=CARTESIAN_POINT ( 'NONE',  ( 30.59788246744356854, -3.614912645528273849, 4.745426083186703003 ) ) ;
#28733=CARTESIAN_POINT ( 'NONE',  ( 22.77327910074270889, 0.4820626211097077118, -6.224882446762404875 ) ) ;
#28734=CARTESIAN_POINT ( 'NONE',  ( 36.20303916938638622, -1.578649729842889649, -5.665109327158619479 ) ) ;
#28738=EDGE_CURVE ( 'NONE', #28626, #36858, #4621, .T. ) ;
#28742=EDGE_CURVE ( 'NONE', #39711, #11084, #24353, .T. ) ;
#28744=CARTESIAN_POINT ( 'NONE',  ( 84.45327006356104960, 2.923007647743876447, -2.091752339247905823 ) ) ;
#28747=CARTESIAN_POINT ( 'NONE',  ( 24.59812680050050915, 2.980866690065322011, 3.560245512678282598 ) ) ;
#28753=ORIENTED_EDGE ( 'NONE', *, *, #12314, .T. ) ;
#28754=ORIENTED_EDGE ( 'NONE', *, *, #7287, .T. ) ;
#28765=CARTESIAN_POINT ( 'NONE',  ( 21.85643539959772497, -14.97654459006671068, 3.851724272136834326 ) ) ;
#28767=CARTESIAN_POINT ( 'NONE',  ( 22.39454719451790510, 4.886617018807966950, -3.092752845356960822 ) ) ;
#28775=CARTESIAN_POINT ( 'NONE',  ( -77.24581433579317036, -6.124437853233426488, -7.754200975113157313 ) ) ;
#28779=CARTESIAN_POINT ( 'NONE',  ( 87.05329302184628659, -1.423768201249274945, 4.835531253876708568 ) ) ;
#28780=DIRECTION ( 'NONE',  ( 1.000000000000000000, 0.000000000000000000, 0.000000000000000000 ) ) ;
#28783=EDGE_CURVE ( 'NONE', #25658, #2020, #21074, .T. ) ;
#28787=CARTESIAN_POINT ( 'NONE',  ( -12.99139449055068241, -10.90558813203967148, 6.000000000000000000 ) ) ;
#28789=CARTESIAN_POINT ( 'NONE',  ( 36.99314941111227739, -2.718566000083574519, 5.980073666940257660 ) ) ;
#28795=CARTESIAN_POINT ( 'NONE',  ( 87.05115134601746263, 0.5777397079708905814, 5.111878656935144427 ) ) ;
#28798=CARTESIAN_POINT ( 'NONE',  ( 14.71586241334793677, -5.063781084897545526, 2.500000000000000444 ) ) ;
#28801=CARTESIAN_POINT ( 'NONE',  ( 14.77291369204805882, 13.25874409045904301, -2.500174547565549243 ) ) ;
#28805=CARTESIAN_POINT ( 'NONE',  ( -71.75719754330091860, 2.253829733506131472, 9.965625675682359130 ) ) ;
#28806=ORIENTED_EDGE ( 'NONE', *, *, #1016, .T. ) ;
#28809=CARTESIAN_POINT ( 'NONE',  ( 24.50968518362478576, 2.239917399590349856, 4.180759367608843924 ) ) ;
#28810=ORIENTED_EDGE ( 'NONE', *, *, #1697, .T. ) ;
#28813=CIRCLE ( 'NONE', #35387, 3.000000000000002665 ) ;
#28819=CARTESIAN_POINT ( 'NONE',  ( 22.78500653003857934, 3.697042830259541724, -3.776378161709064152 ) ) ;
#28821=ORIENTED_EDGE ( 'NONE', *, *, #38805, .T. ) ;
#28823=CARTESIAN_POINT ( 'NONE',  ( 21.85643539959773207, -8.152057848754798997, -9.377623736650162911 ) ) ;
#28824=CARTESIAN_POINT ( 'NONE',  ( 21.87751110072621685, 4.134169920257987130, -2.121951800785348841 ) ) ;
#28827=CARTESIAN_POINT ( 'NONE',  ( 88.47081344899795852, -1.206222823704210301, -3.524641158899461058 ) ) ;
#28828=ORIENTED_EDGE ( 'NONE', *, *, #22395, .T. ) ;
#28829=CARTESIAN_POINT ( 'NONE',  ( 14.77315594796436926, 13.19392823276591464, 2.499999999999996891 ) ) ;
#28831=CARTESIAN_POINT ( 'NONE',  ( 28.89967557733805137, -2.887797800998441744, 4.716891333775404149 ) ) ;
#28832=CARTESIAN_POINT ( 'NONE',  ( 29.11494709149169324, -3.933151727299639244, 4.208129513927731935 ) ) ;
#28833=CARTESIAN_POINT ( 'NONE',  ( 29.10199195035972153, 0.3604134132878261121, -4.748467696825394491 ) ) ;
#28841=CARTESIAN_POINT ( 'NONE',  ( 31.99136750572645482, -3.506164123272953681, 5.093361180844341085 ) ) ;
#28844=CARTESIAN_POINT ( 'NONE',  ( 33.68505034223440475, -3.839218838710527049, 5.138863580400442110 ) ) ;
#28850=LINE ( 'NONE', #38100, #1792 ) ;
#28852=CARTESIAN_POINT ( 'NONE',  ( -62.92837670882106238, 0.7293679304675904085, 6.000000000000000000 ) ) ;
#28854=VERTEX_POINT ( 'NONE', #15702 ) ;
#28859=EDGE_LOOP ( 'NONE', ( #829, #3939, #35218, #17248, #19169 ) ) ;
#28863=CARTESIAN_POINT ( 'NONE',  ( 16.14962678690648090, 10.32852357150096090, -2.711842976054151144 ) ) ;
#28866=DIRECTION ( 'NONE',  ( 0.000000000000000000, 1.000000000000000000, 0.000000000000000000 ) ) ;
#28867=CYLINDRICAL_SURFACE ( 'NONE', #21485, 24.28220113893567600 ) ;
#28868=CARTESIAN_POINT ( 'NONE',  ( 22.63302891745040668, 3.893813116402496277, -3.738829563077739504 ) ) ;
#28871=CARTESIAN_POINT ( 'NONE',  ( 12.97258478262502202, 9.268119072443660400, 3.480631332370867970 ) ) ;
#28873=CARTESIAN_POINT ( 'NONE',  ( 28.93850508814251299, -1.888738275646064668, -5.863986819262115624 ) ) ;
#28875=CARTESIAN_POINT ( 'NONE',  ( -12.99139449055068241, -10.90558813203967148, 6.000000000000000000 ) ) ;
#28880=CARTESIAN_POINT ( 'NONE',  ( 33.66554628656592030, -3.445943206981954443, -5.444051220130533331 ) ) ;
#28888=CARTESIAN_POINT ( 'NONE',  ( 21.85955896937255716, -14.20251193623180441, 2.500000000000000444 ) ) ;
#28889=ADVANCED_FACE ( 'NONE', ( #37318 ), #8493, .T. ) ;
#28890=CARTESIAN_POINT ( 'NONE',  ( 31.70306142352022505, -2.958976183629556278, 5.154427495215030852 ) ) ;
#28898=CARTESIAN_POINT ( 'NONE',  ( 22.39762075202990133, 3.875352353137541339, 3.942491037406270049 ) ) ;
#28903=CARTESIAN_POINT ( 'NONE',  ( 22.61545699184745217, 4.619227728608865213, 3.050121107112468977 ) ) ;
#28904=DIRECTION ( 'NONE',  ( -0.05950379560742589252, 0.006463183370434484251, 0.9982071556390637035 ) ) ;
#28909=CARTESIAN_POINT ( 'NONE',  ( 23.07063981287367582, 0.3569738237481424048, 5.941516061105353685 ) ) ;
#28915=AXIS2_PLACEMENT_3D ( 'NONE', #26281, #13106, #34957 ) ;
#28921=CARTESIAN_POINT ( 'NONE',  ( 23.93232801731964443, 3.995115622954060530, -2.300403959411237320 ) ) ;
#28923=ORIENTED_EDGE ( 'NONE', *, *, #5875, .T. ) ;
#28924=CARTESIAN_POINT ( 'NONE',  ( -76.80627534794649591, -4.528701127649712888, 9.610004701533378935 ) ) ;
#28925=CARTESIAN_POINT ( 'NONE',  ( -17.27251170661583402, -8.656638842136340273, 6.000000000000000000 ) ) ;
#28929=AXIS2_PLACEMENT_3D ( 'NONE', #17680, #36640, #33377 ) ;
#28930=CARTESIAN_POINT ( 'NONE',  ( 28.79870369017745446, -3.878292931925462650, -4.349375427024083862 ) ) ;
#28931=CARTESIAN_POINT ( 'NONE',  ( 37.00971988778469068, -2.249531826949414892, -5.913225602219081445 ) ) ;
#28932=DIRECTION ( 'NONE',  ( -1.682730792515357087E-16, 1.000000000000000000, 0.000000000000000000 ) ) ;
#28933=CARTESIAN_POINT ( 'NONE',  ( 18.48730018318043022, 7.939472255012167246, 3.062856037497708073 ) ) ;
#28937=CARTESIAN_POINT ( 'NONE',  ( -17.69482985384421880, -29.56993018339339940, -6.000000000000000000 ) ) ;
#28938=CARTESIAN_POINT ( 'NONE',  ( 25.45843029652522205, 1.868879512192637593, -4.233311170609479035 ) ) ;
#28939=CARTESIAN_POINT ( 'NONE',  ( 36.01008099166774201, -1.464911901215198764, -5.613471295053200194 ) ) ;
#28947=CARTESIAN_POINT ( 'NONE',  ( 86.42019152727894493, 0.2271775462534226520, 6.017476335466618309 ) ) ;
#28950=CARTESIAN_POINT ( 'NONE',  ( -73.96100403028097503, 6.544720006936636025, -10.78617274266811776 ) ) ;
#28952=CARTESIAN_POINT ( 'NONE',  ( 14.61802081865033642, 12.33286846116140900, 3.500000000000000444 ) ) ;
#28955=DIRECTION ( 'NONE',  ( -0.000000000000000000, -0.000000000000000000, -1.000000000000000000 ) ) ;
#28957=ORIENTED_EDGE ( 'NONE', *, *, #18673, .F. ) ;
#28967=CARTESIAN_POINT ( 'NONE',  ( 33.72876834755415842, -4.609435595580992029, -3.994862081233153006 ) ) ;
#28968=CARTESIAN_POINT ( 'NONE',  ( 22.88108605422135966, 4.308698648288653565, -3.098481689044433551 ) ) ;
#28970=EDGE_CURVE ( 'NONE', #40686, #9974, #16694, .T. ) ;
#28975=CARTESIAN_POINT ( 'NONE',  ( -72.64415850718684453, -1.673418234781224534, -9.853848402383640348 ) ) ;
#28979=CARTESIAN_POINT ( 'NONE',  ( 84.10435792013542766, 3.012680099502687892, -0.4953216543819284889 ) ) ;
#28981=CARTESIAN_POINT ( 'NONE',  ( -69.92837670882107659, -65.19654454972992141, 5.916079783099617906 ) ) ;
#28983=CARTESIAN_POINT ( 'NONE',  ( 1.700390093233090871, -29.56993018339339940, 27.90461065042423527 ) ) ;
#28984=CARTESIAN_POINT ( 'NONE',  ( 32.83305986583096114, -0.9452946091439576870, 5.330791081253222430 ) ) ;
#28990=EDGE_LOOP ( 'NONE', ( #4561, #30593, #23846, #23275, #7173 ) ) ;
#28991=CARTESIAN_POINT ( 'NONE',  ( 34.92978150137876270, -1.709224254641393159, 5.658035201884869636 ) ) ;
#28993=CARTESIAN_POINT ( 'NONE',  ( 88.42181306311033495, -0.9618525881974497871, -1.725133412809377598 ) ) ;
#28998=ORIENTED_EDGE ( 'NONE', *, *, #18334, .F. ) ;
#29002=CARTESIAN_POINT ( 'NONE',  ( -80.87788611484333501, -6.601209159344090693, 1.087894082802069562 ) ) ;
#29007=DIRECTION ( 'NONE',  ( 0.000000000000000000, 1.000000000000000000, 0.000000000000000000 ) ) ;
#29008=CARTESIAN_POINT ( 'NONE',  ( 24.02675112551502323, 1.887447688529081402, 4.512062677995031024 ) ) ;
#29020=CARTESIAN_POINT ( 'NONE',  ( 22.56869731596198392, 3.964702178913764641, -3.727352237020760573 ) ) ;
#29024=CARTESIAN_POINT ( 'NONE',  ( 21.85643539959778892, 8.438975622634238505, -5.206363084432100052 ) ) ;
#29025=CARTESIAN_POINT ( 'NONE',  ( 21.86257038569385003, 3.862145465805826738, 3.386728275820227729 ) ) ;
#29026=ORIENTED_EDGE ( 'NONE', *, *, #14099, .T. ) ;
#29029=CARTESIAN_POINT ( 'NONE',  ( 86.54367451126900335, 1.050056116286632646, -5.670096781828877219 ) ) ;
#29031=DIRECTION ( 'NONE',  ( -0.000000000000000000, -0.000000000000000000, -1.000000000000000000 ) ) ;
#29033=CARTESIAN_POINT ( 'NONE',  ( 35.95092945659100536, -2.121302639717296046, 5.817410036852332489 ) ) ;
#29035=CARTESIAN_POINT ( 'NONE',  ( 35.33511003955339902, -3.170233155793333868, -5.721296523174722815 ) ) ;
#29037=CARTESIAN_POINT ( 'NONE',  ( 84.10567841564332525, 3.011090578911546967, -0.2542956616254711255 ) ) ;
#29042=CARTESIAN_POINT ( 'NONE',  ( 29.48001143125632240, -3.085193311930952031, 4.807466779239847554 ) ) ;
#29045=CARTESIAN_POINT ( 'NONE',  ( 35.36813255412664603, -3.791872901862796130, 5.511222840556704305 ) ) ;
#29057=CARTESIAN_POINT ( 'NONE',  ( 21.88221554822858295, 5.657183511159394662, 3.265289024689040254 ) ) ;
#29070=DIRECTION ( 'NONE',  ( -0.000000000000000000, -0.000000000000000000, -1.000000000000000000 ) ) ;
#29072=CARTESIAN_POINT ( 'NONE',  ( 22.77354003839862884, 3.736677582877315995, -3.760759721776010700 ) ) ;
#29074=CARTESIAN_POINT ( 'NONE',  ( 86.13511395365257783, 1.606676384832600224, -4.558527568769633831 ) ) ;
#29075=CARTESIAN_POINT ( 'NONE',  ( 27.17726507492083599, 0.7866376163037266389, 5.581651230154481169 ) ) ;
#29077=DIRECTION ( 'NONE',  ( 1.000000000000000000, 0.000000000000000000, 0.000000000000000000 ) ) ;
#29084=CARTESIAN_POINT ( 'NONE',  ( 34.12028950839226127, -3.462206709392819715, -5.516488667911798593 ) ) ;
#29089=DIRECTION ( 'NONE',  ( -1.000000000000000000, 0.000000000000000000, 0.000000000000000000 ) ) ;
#29091=CARTESIAN_POINT ( 'NONE',  ( 31.96342931950348643, -2.972543090938732036, 5.195064202404578779 ) ) ;
#29093=CARTESIAN_POINT ( 'NONE',  ( 22.97035745888615565, 2.781248465002744474, 3.791477840290978563 ) ) ;
#29099=DIRECTION ( 'NONE',  ( -1.000000000000000000, 0.000000000000000000, 0.000000000000000000 ) ) ;
#29100=CARTESIAN_POINT ( 'NONE',  ( 23.92691214014465473, 2.953265760775589666, 3.829296936384404049 ) ) ;
#29106=CARTESIAN_POINT ( 'NONE',  ( 22.61499008964769430, 4.623430995783932573, 3.044749204892538863 ) ) ;
#29108=CARTESIAN_POINT ( 'NONE',  ( 16.07163779223724731, -3.513190516767646709, 2.694550467567401686 ) ) ;
#29113=CARTESIAN_POINT ( 'NONE',  ( 22.30438977958806035, 0.2664073136237887218, 7.087798616884243508 ) ) ;
#29118=ORIENTED_EDGE ( 'NONE', *, *, #16861, .F. ) ;
#29119=EDGE_CURVE ( 'NONE', #16957, #23963, #8463, .T. ) ;
#29120=DIRECTION ( 'NONE',  ( -0.000000000000000000, -1.000000000000000000, -0.000000000000000000 ) ) ;
#29124=CARTESIAN_POINT ( 'NONE',  ( 25.48535437492803624, -4.309695067542732794, -2.926019122942394191 ) ) ;
#29128=CARTESIAN_POINT ( 'NONE',  ( -79.66837676813406688, -6.645208303062806188, 4.876177452525313427 ) ) ;
#29129=CARTESIAN_POINT ( 'NONE',  ( 21.77775980223391628, 0.1997282058778115377, -8.433602713107923421 ) ) ;
#29131=CARTESIAN_POINT ( 'NONE',  ( 20.91912229527441269, 4.580706636100547513, -2.655338311533547380 ) ) ;
#29140=CARTESIAN_POINT ( 'NONE',  ( 22.13241655903548377, 0.4569658243204014481, -7.207667138002770812 ) ) ;
#29141=CARTESIAN_POINT ( 'NONE',  ( 35.56739675845194881, -1.226987158729853533, -5.500502591869192770 ) ) ;
#29148=CARTESIAN_POINT ( 'NONE',  ( 84.54687988124997844, 2.467165036067117789, -3.672804150685311964 ) ) ;
#29150=CARTESIAN_POINT ( 'NONE',  ( -77.82107608900516027, 9.895938843071389712, -8.879257655445593755 ) ) ;
#29151=B_SPLINE_CURVE_WITH_KNOTS ( 'NONE', 3,
 ( #24525, #36474, #21654, #37076, #27006, #8456, #15257, #30301, #39552, #20819 ),
 .UNSPECIFIED., .F., .F.,
 ( 4, 2, 2, 2, 4 ),
 ( 0.000000000000000000, 0.0003911417017416531365, 0.0007822834034833063815, 0.001173425105224959681, 0.001564566806966613197 ),
 .UNSPECIFIED. ) ;
#29154=ORIENTED_EDGE ( 'NONE', *, *, #27798, .F. ) ;
#29158=CARTESIAN_POINT ( 'NONE',  ( 37.19747299874393320, -2.841585884120807481, 5.999818732555961098 ) ) ;
#29167=CARTESIAN_POINT ( 'NONE',  ( 21.85643539959779247, -15.31483402087699197, 0.9306824932977513232 ) ) ;
#29175=CARTESIAN_POINT ( 'NONE',  ( -71.81612654988926181, 3.537828150600389687, -9.960561527263866566 ) ) ;
#29179=CARTESIAN_POINT ( 'NONE',  ( 86.38407091574619301, -0.4420343715668084150, 5.843987706619403255 ) ) ;
#29187=FACE_OUTER_BOUND ( 'NONE', #18347, .T. ) ;
#29189=CARTESIAN_POINT ( 'NONE',  ( 32.78089741354497022, -0.9280409695437186191, 5.322649869020279922 ) ) ;
#29192=CARTESIAN_POINT ( 'NONE',  ( 86.85660104221420852, 0.7962678431171816840, 5.176869783008884340 ) ) ;
#29200=CARTESIAN_POINT ( 'NONE',  ( -72.37627261349332741, -1.026670002906238333, 9.895491078337210311 ) ) ;
#29207=CARTESIAN_POINT ( 'NONE',  ( 24.35809287307254323, 1.975542649453049693, 4.376866090386280383 ) ) ;
#29218=CARTESIAN_POINT ( 'NONE',  ( 22.80705867304895307, 3.513075761590381152, -3.907165907269140703 ) ) ;
#29221=ORIENTED_EDGE ( 'NONE', *, *, #35353, .F. ) ;
#29222=CARTESIAN_POINT ( 'NONE',  ( 21.85643539959780313, 0.1435845899245215551, -12.62009698158557747 ) ) ;
#29223=CARTESIAN_POINT ( 'NONE',  ( 20.05068032855264448, 11.88301801997804397, 1.993596777106166673 ) ) ;
#29224=VERTEX_POINT ( 'NONE', #11933 ) ;
#29227=CARTESIAN_POINT ( 'NONE',  ( 86.10913233486274976, 1.283334762834210441, -5.698406565159564785 ) ) ;
#29232=CARTESIAN_POINT ( 'NONE',  ( 21.52073695273352882, -2.639896720919388873, 3.565229501100848353 ) ) ;
#29235=CARTESIAN_POINT ( 'NONE',  ( 32.03545946682555723, -3.767761596829544146, 4.810237983490988967 ) ) ;
#29236=CARTESIAN_POINT ( 'NONE',  ( 14.78316203198160039, -5.958431814372524116, -2.513667985851932407 ) ) ;
#29237=CARTESIAN_POINT ( 'NONE',  ( 35.78601669305616184, -3.163418368850383189, -5.791671411672478342 ) ) ;
#29239=CARTESIAN_POINT ( 'NONE',  ( 84.59056625886891823, 2.408269107882004878, 3.818220528950529324 ) ) ;
#29246=CARTESIAN_POINT ( 'NONE',  ( 37.18669192317609884, -2.963439294260284296, 6.000022183381657825 ) ) ;
#29251=CARTESIAN_POINT ( 'NONE',  ( 87.38843002206890276, -1.854803145455693913, 3.937212981888271734 ) ) ;
#29252=ADVANCED_FACE ( 'NONE', ( #3734 ), #20069, .F. ) ;
#29256=CARTESIAN_POINT ( 'NONE',  ( 33.45749450797183044, -3.829747548865578555, 5.093667367007288505 ) ) ;
#29260=AXIS2_PLACEMENT_3D ( 'NONE', #36014, #1631, #14171 ) ;
#29269=ORIENTED_EDGE ( 'NONE', *, *, #8966, .F. ) ;
#29277=CARTESIAN_POINT ( 'NONE',  ( 27.90799128822289177, 2.452171383980988661, -2.014541967423249424 ) ) ;
#29280=CARTESIAN_POINT ( 'NONE',  ( -79.82037350764412054, -5.590114488123880676, -6.712154371197549985 ) ) ;
#29283=CARTESIAN_POINT ( 'NONE',  ( 35.80541780769373617, -3.523238331632154274, -5.749476952422626574 ) ) ;
#29289=CARTESIAN_POINT ( 'NONE',  ( 22.04556973325361113, -11.44728196981451696, -2.500000000000000000 ) ) ;
#29292=CIRCLE ( 'NONE', #18096, 7.744449365083023729 ) ;
#29296=CARTESIAN_POINT ( 'NONE',  ( 34.77027720814614042, -3.601453098587749313, 5.565789519727438517 ) ) ;
#29302=LINE ( 'NONE', #1115, #27891 ) ;
#29304=CARTESIAN_POINT ( 'NONE',  ( 23.70161070757133359, 3.021634694769598450, 3.856184811640798848 ) ) ;
#29314=CARTESIAN_POINT ( 'NONE',  ( 27.42275297525273814, 1.007386247029351978, 4.486341073878296726 ) ) ;
#29315=CARTESIAN_POINT ( 'NONE',  ( 14.61802081865040748, -4.461995682952455411, -2.500000000000015987 ) ) ;
#29319=CARTESIAN_POINT ( 'NONE',  ( -12.99139449055068241, 13.37661300689600097, 6.000000000000000000 ) ) ;
#29320=AXIS2_PLACEMENT_3D ( 'NONE', #11955, #24117, #20827 ) ;
#29323=CARTESIAN_POINT ( 'NONE',  ( 22.37806265499392566, 3.168015787195890720, 7.828147373443384183 ) ) ;
#29326=CARTESIAN_POINT ( 'NONE',  ( -80.34222039028743723, -6.644459708051462243, 3.397825296345740043 ) ) ;
#29331=CARTESIAN_POINT ( 'NONE',  ( 34.14217736537160164, -3.847370433800512135, -5.235592723209181898 ) ) ;
#29332=CARTESIAN_POINT ( 'NONE',  ( 30.73796255296185365, -3.302600333584832626, -4.965265549407608781 ) ) ;
#29339=CARTESIAN_POINT ( 'NONE',  ( 14.77315594796849574, 13.19392823276453441, -2.500000000000005773 ) ) ;
#29344=EDGE_CURVE ( 'NONE', #13934, #28626, #28413, .T. ) ;
#29345=CARTESIAN_POINT ( 'NONE',  ( 21.73878006178032507, 6.093844739303823310, -3.276015879424795330 ) ) ;
#29346=CARTESIAN_POINT ( 'NONE',  ( 85.28131701390645958, 1.700283277630491030, -5.218886290300497777 ) ) ;
#29347=EDGE_CURVE ( 'NONE', #23963, #2909, #33594, .T. ) ;
#29350=CARTESIAN_POINT ( 'NONE',  ( -78.73873693005447194, 10.21307840320916860, -8.022592256280697498 ) ) ;
#29359=CARTESIAN_POINT ( 'NONE',  ( 14.72270832792595030, 13.21629034704322336, -2.500000000000005773 ) ) ;
#29365=CARTESIAN_POINT ( 'NONE',  ( 33.84040353105311283, -5.117034793841976459, -2.696338666777271076 ) ) ;
#29367=CARTESIAN_POINT ( 'NONE',  ( 21.83032690866058800, 5.963236517223874600, -3.135749234919836148 ) ) ;
#29370=ORIENTED_EDGE ( 'NONE', *, *, #37764, .T. ) ;
#29373=CARTESIAN_POINT ( 'NONE',  ( -74.60868374468475395, -4.441676580721787282, -9.303113757966089636 ) ) ;
#29391=CARTESIAN_POINT ( 'NONE',  ( 36.78945405456298801, -3.041985858871208315, 5.948282080159894569 ) ) ;
#29393=CARTESIAN_POINT ( 'NONE',  ( 85.75411537215676105, 2.034632074852215311, 4.270953678727185121 ) ) ;
#29407=EDGE_LOOP ( 'NONE', ( #27971, #19974, #4943, #34828, #1162 ) ) ;
#29413=CARTESIAN_POINT ( 'NONE',  ( 21.86392410096259198, 0.3939289551572383030, 7.936696350653804188 ) ) ;
#29416=DIRECTION ( 'NONE',  ( 0.000000000000000000, -0.000000000000000000, -1.000000000000000000 ) ) ;
#29419=LINE ( 'NONE', #16441, #5375 ) ;
#29422=CARTESIAN_POINT ( 'NONE',  ( 24.24423223564896546, 3.110186912964516548, -3.522988159190304280 ) ) ;
#29424=DIRECTION ( 'NONE',  ( -1.000000000000000000, 0.000000000000000000, 0.000000000000000000 ) ) ;
#29425=CARTESIAN_POINT ( 'NONE',  ( 22.33830324658017830, 5.012815666754769417, -5.469126444728273029 ) ) ;
#29426=CARTESIAN_POINT ( 'NONE',  ( 21.85970433026865223, 3.598116536247359498, -3.919871293595560413 ) ) ;
#29429=B_SPLINE_CURVE_WITH_KNOTS ( 'NONE', 3,
 ( #29774, #39434, #24207, #1796, #1591, #36769, #21133, #14122, #14941, #33700, #5479, #40058, #26699, #39235, #11023, #11225, #23792, #36367, #8136, #20706, #5075, #17604, #2004, #14524, #27810, #37287, #37678, #31736, #2736, #12379, #22071, #21658, #12165, #37892, #12779, #10445, #1009, #31534, #34642, #18969, #19921, #31127, #28432, #22278, #34847, #24738, #15875, #7363, #6007, #28643, #240, #9080, #6416 ),
 .UNSPECIFIED., .F., .F.,
 ( 4, 1, 2, 2, 1, 1, 1, 1, 2, 2, 1, 1, 1, 1, 1, 2, 2, 1, 1, 1, 1, 2, 2, 1, 1, 1, 1, 1, 2, 2, 1, 1, 1, 1, 1, 1, 2, 2, 4 ),
 ( 0.5000000000000000000, 0.5312500000000078826, 0.5351562500000083267, 0.5390625000000087708, 0.5468750000000084377, 0.5546875000000081046, 0.5585937500000075495, 0.5605468750000069944, 0.5615234375000062172, 0.5625000000000054401, 0.5937500000000077716, 0.6093750000000086597, 0.6171875000000089928, 0.6210937500000092149, 0.6230468750000091038, 0.6240234375000089928, 0.6250000000000089928, 0.6875000000000114353, 0.7187500000000128786, 0.7343750000000134337, 0.7421875000000137668, 0.7460937500000138778, 0.7500000000000139888, 0.8125000000000164313, 0.8437500000000177636, 0.8593750000000184297, 0.8671875000000188738, 0.8710937500000190958, 0.8730468750000193179, 0.8750000000000196509, 0.9062500000000235367, 0.9218750000000255351, 0.9296875000000268674, 0.9335937500000273115, 0.9355468750000275335, 0.9365234375000272005, 0.9370117187500273115, 0.9375000000000275335, 1.000000000000000000 ),
 .UNSPECIFIED. ) ;
#29435=CARTESIAN_POINT ( 'NONE',  ( 32.47467932546493330, -3.787890779724774948, 4.892967751047994973 ) ) ;
#29436=FACE_OUTER_BOUND ( 'NONE', #37494, .T. ) ;
#29437=CARTESIAN_POINT ( 'NONE',  ( 33.62755378216321844, -1.232175040594724713, -5.454791071804911518 ) ) ;
#29441=CARTESIAN_POINT ( 'NONE',  ( 30.20718958106393615, -3.692124001418715551, -4.611238308815850395 ) ) ;
#29447=ORIENTED_EDGE ( 'NONE', *, *, #9667, .F. ) ;
#29448=CARTESIAN_POINT ( 'NONE',  ( 35.22017179206324755, -1.048857254921915949, 5.412365112790203270 ) ) ;
#29449=CARTESIAN_POINT ( 'NONE',  ( 15.01262998282573946, -3.946207525411958184, 2.549482009284877115 ) ) ;
#29451=CARTESIAN_POINT ( 'NONE',  ( 86.73589842370522263, -0.9811105784606377611, 5.402284631838752738 ) ) ;
#29459=CARTESIAN_POINT ( 'NONE',  ( 22.30551760662672223, 4.735879390933545707, 3.387776000085759964 ) ) ;
#29463=CARTESIAN_POINT ( 'NONE',  ( 14.72123706662768505, -4.461995682952463405, -2.504003097347854645 ) ) ;
#29470=CARTESIAN_POINT ( 'NONE',  ( 24.20640518876499669, 2.566492102625094418, -4.042989007339715890 ) ) ;
#29477=CARTESIAN_POINT ( 'NONE',  ( 32.63594197759655913, -2.548278591510585667, -5.894033951951210604 ) ) ;
#29478=EDGE_CURVE ( 'NONE', #2897, #37746, #39906, .T. ) ;
#29481=CARTESIAN_POINT ( 'NONE',  ( 22.82081674902891066, -6.972797972010963186, 0.5552882429563011923 ) ) ;
#29484=ORIENTED_EDGE ( 'NONE', *, *, #27148, .F. ) ;
#29487=CARTESIAN_POINT ( 'NONE',  ( 36.94812879981065379, -2.593733626342286769, -5.973047111718997826 ) ) ;
#29496=CARTESIAN_POINT ( 'NONE',  ( 36.18524227031805651, -3.553218394490209597, 5.771100729284209585 ) ) ;
#29503=CARTESIAN_POINT ( 'NONE',  ( 30.87059228904019648, -3.396537768743968844, 4.950897058115855565 ) ) ;
#29507=CARTESIAN_POINT ( 'NONE',  ( -58.92473026143653669, 13.37661300689600274, -2.500000000000000000 ) ) ;
#29509=CARTESIAN_POINT ( 'NONE',  ( 21.71254722604186327, 6.323917084280038736, 3.194779952286587399 ) ) ;
#29516=CARTESIAN_POINT ( 'NONE',  ( 26.73338393872905527, 0.9282423383602553812, 4.382137618851254857 ) ) ;
#29525=CARTESIAN_POINT ( 'NONE',  ( 26.57131730419879290, 2.962615056577905026, -1.092182624680714254 ) ) ;
#29528=CARTESIAN_POINT ( 'NONE',  ( -79.67547651979579371, -5.606679663933569202, 4.861676929742372089 ) ) ;
#29529=CARTESIAN_POINT ( 'NONE',  ( 23.06098311254805466, 0.3526106142807417521, -5.951280228554626461 ) ) ;
#29533=ORIENTED_EDGE ( 'NONE', *, *, #23741, .T. ) ;
#29534=CARTESIAN_POINT ( 'NONE',  ( 37.17621594122605444, -2.565172031526568919, -5.981066268316136636 ) ) ;
#29541=CARTESIAN_POINT ( 'NONE',  ( 25.62812034757272173, 2.162893437960721865, -4.131162739758373448 ) ) ;
#29545=CARTESIAN_POINT ( 'NONE',  ( 84.33668400229728945, 2.728897857615574019, 2.746074863882507877 ) ) ;
#29548=CARTESIAN_POINT ( 'NONE',  ( 26.60736997101286505, 1.631599532540721542, 4.332120141861649287 ) ) ;
#29560=CARTESIAN_POINT ( 'NONE',  ( 18.96853221647454646, 7.708738308554112351, -3.077308032275870797 ) ) ;
#29562=FACE_OUTER_BOUND ( 'NONE', #39912, .T. ) ;
#29563=CARTESIAN_POINT ( 'NONE',  ( 23.14181338739152238, 4.049881389590580305, -3.073623331090673538 ) ) ;
#29569=CARTESIAN_POINT ( 'NONE',  ( 14.61802081865032932, -4.461849342347350422, 2.499999999999997780 ) ) ;
#29571=CARTESIAN_POINT ( 'NONE',  ( -74.03934154708541371, -3.833512911058256645, -9.504820148027839366 ) ) ;
#29581=CARTESIAN_POINT ( 'NONE',  ( -17.27251170661583402, -8.656638842136340273, -6.000000000000000000 ) ) ;
#29585=CARTESIAN_POINT ( 'NONE',  ( 29.10122315827134898, 0.3582907782008117326, 4.748347708226712705 ) ) ;
#29588=CARTESIAN_POINT ( 'NONE',  ( 85.02879235234962607, 2.798117532367836446, 2.624272742801059710 ) ) ;
#29589=AXIS2_PLACEMENT_3D ( 'NONE', #34524, #13079, #135 ) ;
#29601=CARTESIAN_POINT ( 'NONE',  ( 24.90975462926189010, 3.541767663397652033, 0.6518453417789448201 ) ) ;
#29603=CARTESIAN_POINT ( 'NONE',  ( 23.61787448442827753, 0.7654929067543206900, 5.373130871398858588 ) ) ;
#29606=CARTESIAN_POINT ( 'NONE',  ( 14.69558838330753936, -3.003688195628454238, 6.000000000000001776 ) ) ;
#29610=CARTESIAN_POINT ( 'NONE',  ( 22.91810752083389602, 4.152906525941994609, -3.257904903544968978 ) ) ;
#29612=CARTESIAN_POINT ( 'NONE',  ( -71.90221254882203539, -0.5206366332505392158, 5.920661432671355584 ) ) ;
#29615=CARTESIAN_POINT ( 'NONE',  ( 22.32365817596653557, 5.835156701882857178, 3.488260158266504263 ) ) ;
#29617=CARTESIAN_POINT ( 'NONE',  ( 21.85643539959776760, 3.765123657700408355, 3.918568846604040257 ) ) ;
#29623=CARTESIAN_POINT ( 'NONE',  ( 85.16823716249373888, 2.433965874742513247, 4.055466505201608562 ) ) ;
#29625=ORIENTED_EDGE ( 'NONE', *, *, #4448, .F. ) ;
#29626=CARTESIAN_POINT ( 'NONE',  ( -80.66010496297788279, -5.648439302891065772, 5.209062318100336597 ) ) ;
#29629=CARTESIAN_POINT ( 'NONE',  ( 21.50482873268578743, -2.719662516908865069, -3.562746638620634343 ) ) ;
#29630=CARTESIAN_POINT ( 'NONE',  ( 32.77912487546454656, -0.9333593928079626512, -5.322373221583833747 ) ) ;
#29631=DIRECTION ( 'NONE',  ( -1.000000000000000000, -1.165409145176969993E-16, 0.000000000000000000 ) ) ;
#29637=CARTESIAN_POINT ( 'NONE',  ( -18.48280404870591553, -63.98126818465317456, 2.500000000000000000 ) ) ;
#29639=ORIENTED_EDGE ( 'NONE', *, *, #15939, .T. ) ;
#29641=CARTESIAN_POINT ( 'NONE',  ( 34.79231454646104993, -3.833543758068950869, 5.378533583580677124 ) ) ;
#29644=CARTESIAN_POINT ( 'NONE',  ( 33.43971231075012440, -3.588053834546123255, 5.336497937005737491 ) ) ;
#29645=CARTESIAN_POINT ( 'NONE',  ( 86.83589974223885122, -1.124279187257583912, 5.239974236049660838 ) ) ;
#29651=CARTESIAN_POINT ( 'NONE',  ( -60.15914593959029588, -52.45670913645259503, -2.307692307692302158 ) ) ;
#29654=CARTESIAN_POINT ( 'NONE',  ( 22.97383871700119684, 3.759880532170991607, 3.599142388413823390 ) ) ;
#29661=CARTESIAN_POINT ( 'NONE',  ( 22.26111053501417913, 2.653359810932870211, -4.982668050499428958 ) ) ;
#29662=CARTESIAN_POINT ( 'NONE',  ( -89.00859394718983708, 2.429809908903242555, 12.50000000000000000 ) ) ;
#29664=CARTESIAN_POINT ( 'NONE',  ( 26.91150311004617990, 1.351951412127374130, -4.406588936121679900 ) ) ;
#29669=CARTESIAN_POINT ( 'NONE',  ( 88.32659454254844889, -0.8548986265586405731, 1.105665148257566566 ) ) ;
#29670=CARTESIAN_POINT ( 'NONE',  ( 33.51852797086635150, -3.949141208872448683, 4.993608438669980387 ) ) ;
#29672=CARTESIAN_POINT ( 'NONE',  ( -72.41861705067529442, -46.92014984782673537, 9.888354608821900982 ) ) ;
#29675=CARTESIAN_POINT ( 'NONE',  ( 8.290806648384990041, -35.94265729135299381, 6.000000000000000000 ) ) ;
#29678=CARTESIAN_POINT ( 'NONE',  ( 36.80679559313785632, -3.101469264525490654, -5.950988646661206083 ) ) ;
#29684=VERTEX_POINT ( 'NONE', #27143 ) ;
#29685=CARTESIAN_POINT ( 'NONE',  ( 35.97282836976979326, -1.842333002647675633, 5.810885693563370147 ) ) ;
#29696=CARTESIAN_POINT ( 'NONE',  ( 0.6783104270758654186, -48.60743831809499227, 6.000000000000000000 ) ) ;
#29700=CARTESIAN_POINT ( 'NONE',  ( 23.14061585149417510, 4.042732116653498409, 3.088342274992314618 ) ) ;
#29702=CARTESIAN_POINT ( 'NONE',  ( 17.93706920410982875, -3.171549663534191321, 2.963851838818105211 ) ) ;
#29709=CARTESIAN_POINT ( 'NONE',  ( 21.73424372594157816, 0.2275660760974567987, 9.075264012513089895 ) ) ;
#29710=CARTESIAN_POINT ( 'NONE',  ( 14.77222812468959035, -4.461995682952466957, -2.511961485181824383 ) ) ;
#29716=CARTESIAN_POINT ( 'NONE',  ( 91.69672933337632514, -4.640393979863029372, 6.000000000000001776 ) ) ;
#29717=CARTESIAN_POINT ( 'NONE',  ( 27.13744335700502219, 0.8961374054434056990, -5.485310518450965844 ) ) ;
#29720=CARTESIAN_POINT ( 'NONE',  ( -79.44656165559027272, -5.517286240398389552, 7.192311668639653988 ) ) ;
#29721=CARTESIAN_POINT ( 'NONE',  ( 22.61462763620000160, 0.2954212214349751786, -6.495682540442993869 ) ) ;
#29725=CARTESIAN_POINT ( 'NONE',  ( 25.73195067821911763, 2.635022193550605074, -3.526316274269030160 ) ) ;
#29726=CARTESIAN_POINT ( 'NONE',  ( 4.588767459758324848E-15, -39.37473357531881391, 6.000000000000000000 ) ) ;
#29733=ORIENTED_EDGE ( 'NONE', *, *, #7068, .T. ) ;
#29737=VERTEX_POINT ( 'NONE', #9807 ) ;
#29738=CARTESIAN_POINT ( 'NONE',  ( 85.17103880321602105, 1.638380925414154587, -5.247232096711407223 ) ) ;
#29744=CARTESIAN_POINT ( 'NONE',  ( -4.890026461918809630, -25.50263309590217276, 6.000000000000001776 ) ) ;
#29753=ADVANCED_FACE ( 'NONE', ( #32061 ), #6321, .F. ) ;
#29758=CARTESIAN_POINT ( 'NONE',  ( 21.85643539959775694, 3.570402768353612810, -13.15459721397892423 ) ) ;
#29763=CARTESIAN_POINT ( 'NONE',  ( 14.75543128875859722, -5.142877266070694731, 2.500000000018098856 ) ) ;
#29764=CARTESIAN_POINT ( 'NONE',  ( -72.95888282680236614, 1.037983118628833745, -10.95077940476028644 ) ) ;
#29771=CARTESIAN_POINT ( 'NONE',  ( 27.43879754216082389, 0.9604377377020558715, 4.488885984917203587 ) ) ;
#29774=CARTESIAN_POINT ( 'NONE',  ( 86.46043323462474461, 1.241262327860113590, 4.894917242394325463 ) ) ;
#29778=CARTESIAN_POINT ( 'NONE',  ( 35.33524896685774053, -3.237440951119502142, 5.721318206140924900 ) ) ;
#29780=EDGE_CURVE ( 'NONE', #22791, #6415, #18249, .T. ) ;
#29783=CARTESIAN_POINT ( 'NONE',  ( 87.25532471891827413, 0.3484024848758522364, -5.186905954794287510 ) ) ;
#29784=EDGE_CURVE ( 'NONE', #11160, #13150, #1641, .T. ) ;
#29792=PLANE ( 'NONE',  #40458 ) ;
#29793=EDGE_CURVE ( 'NONE', #5201, #2909, #39778, .T. ) ;
#29796=EDGE_CURVE ( 'NONE', #35457, #37237, #18147, .T. ) ;
#29799=CARTESIAN_POINT ( 'NONE',  ( 8.290806648384990041, -25.50263309590217276, 27.90461065042423527 ) ) ;
#29801=CARTESIAN_POINT ( 'NONE',  ( 22.17211141822430420, 0.6012630956800495419, 7.008217722012737738 ) ) ;
#29806=CARTESIAN_POINT ( 'NONE',  ( 82.38753728249152175, 5.816132372599501110, -6.000000000000000888 ) ) ;
#29807=DIRECTION ( 'NONE',  ( 0.000000000000000000, -0.000000000000000000, -1.000000000000000000 ) ) ;
#29811=CARTESIAN_POINT ( 'NONE',  ( 23.41598892685735578, 3.603782756865482106, -3.423970361731152323 ) ) ;
#29814=CARTESIAN_POINT ( 'NONE',  ( 21.85643539959775694, 0.06084538214464753347, 12.63034898425695296 ) ) ;
#29815=CARTESIAN_POINT ( 'NONE',  ( 21.86951112228125282, 3.097095171886816711, 3.923778634572944846 ) ) ;
#29816=CARTESIAN_POINT ( 'NONE',  ( 16.63788116708428078, 9.878167618073407041, 2.500000000000023537 ) ) ;
#29818=CARTESIAN_POINT ( 'NONE',  ( 85.76120202873109122, 1.723374722402979620, 5.285180586055219898 ) ) ;
#29822=CARTESIAN_POINT ( 'NONE',  ( -81.51102537425536809, -5.630155644727341979, 2.768663238321263265 ) ) ;
#29824=CARTESIAN_POINT ( 'NONE',  ( 21.78047233922835346, 5.616103166486084319, -3.473245622192032034 ) ) ;
#29825=CARTESIAN_POINT ( 'NONE',  ( 19.67202969158519821, -2.692786188159640659, -3.276694021844582583 ) ) ;
#29826=CARTESIAN_POINT ( 'NONE',  ( 36.79718629682508180, -2.556927207590028672, -5.949488883569893360 ) ) ;
#29837=ORIENTED_EDGE ( 'NONE', *, *, #39077, .T. ) ;
#29838=CARTESIAN_POINT ( 'NONE',  ( 32.06910790505158104, 0.2527932190318202266, 4.727196575052298400 ) ) ;
#29841=CARTESIAN_POINT ( 'NONE',  ( 86.62542987116634663, -0.8173961967003109397, 5.560941923137655785 ) ) ;
#29856=CARTESIAN_POINT ( 'NONE',  ( 22.68640543563817857, 4.358088089980108215, 3.272418636457262053 ) ) ;
#29861=CARTESIAN_POINT ( 'NONE',  ( 28.29477944214842822, -2.858814435932810483, -4.622482662410751786 ) ) ;
#29864=CARTESIAN_POINT ( 'NONE',  ( 24.65008494010616147, 2.678007333153050951, -3.905301012187318843 ) ) ;
#29866=CARTESIAN_POINT ( 'NONE',  ( 14.77500745536057813, -5.175466302041957789, 2.500000552286355759 ) ) ;
#29867=CARTESIAN_POINT ( 'NONE',  ( -60.92837670882106238, -23.80776546975053165, 0.000000000000000000 ) ) ;
#29868=CARTESIAN_POINT ( 'NONE',  ( -80.92837670882107659, 2.429809908903242555, 12.50000000000000000 ) ) ;
#29871=CARTESIAN_POINT ( 'NONE',  ( 85.27007178914716690, 2.578332801382848594, -1.917248250713118773 ) ) ;
#29872=CARTESIAN_POINT ( 'NONE',  ( 32.92332271219583362, -2.910100397871670186, 5.759571882993297365 ) ) ;
#29874=CARTESIAN_POINT ( 'NONE',  ( -71.68313049177861274, -45.80610001491483985, 9.973116064590190177 ) ) ;
#29876=CARTESIAN_POINT ( 'NONE',  ( -73.47531904699276595, -0.7173371340867340518, -10.88120764735859680 ) ) ;
#29877=CARTESIAN_POINT ( 'NONE',  ( 14.81039496248155629, -5.583982002385155852, 2.503401465924845137 ) ) ;
#29878=B_SPLINE_CURVE_WITH_KNOTS ( 'NONE', 3,
 ( #32721, #38465, #29612, #38670, #16636, #17240, #10468, #1431, #20532, #39065 ),
 .UNSPECIFIED., .F., .F.,
 ( 4, 2, 2, 2, 4 ),
 ( 1.084202172485504434E-19, 0.0003915841590506208693, 0.0007831683181012415217, 0.001174752477151862120, 0.001566336636202482393 ),
 .UNSPECIFIED. ) ;
#29880=CARTESIAN_POINT ( 'NONE',  ( 33.45607284416932004, -3.169907100080228801, -5.428027324148745336 ) ) ;
#29886=CARTESIAN_POINT ( 'NONE',  ( 36.47586202471227779, -3.472083087333631468, 5.836410874819898176 ) ) ;
#29901=CARTESIAN_POINT ( 'NONE',  ( 23.43270483355060563, 3.786512555878049024, 3.121339484469592307 ) ) ;
#29905=CARTESIAN_POINT ( 'NONE',  ( 29.25516034266419396, -9.786766584782256473, -2.500000000000003997 ) ) ;
#29906=EDGE_LOOP ( 'NONE', ( #28828, #4016 ) ) ;
#29908=CARTESIAN_POINT ( 'NONE',  ( 23.05353214843946574, 0.3448042878357789331, 5.959785611882738365 ) ) ;
#29909=CARTESIAN_POINT ( 'NONE',  ( 14.75295547215416292, -4.607810090512766799, -2.508621623712387283 ) ) ;
#29912=CARTESIAN_POINT ( 'NONE',  ( 37.09585205635672622, -3.161667249977912597, -5.975077866033308815 ) ) ;
#29914=CARTESIAN_POINT ( 'NONE',  ( 14.69558838330753936, 10.99631180437154399, -6.000000000000000888 ) ) ;
#29915=CARTESIAN_POINT ( 'NONE',  ( 27.88065694771982450, 2.580388505813413502, -1.055963728923108524 ) ) ;
#29919=CARTESIAN_POINT ( 'NONE',  ( -81.24448366233951901, -5.645114717358096001, 3.737607825908031867 ) ) ;
#29920=CARTESIAN_POINT ( 'NONE',  ( 25.40499790527096380, 0.6691154281967053308, -4.599878778758904829 ) ) ;
#29925=CARTESIAN_POINT ( 'NONE',  ( 35.82496331154815294, -3.676156692585681895, -5.658730661258451811 ) ) ;
#29940=CARTESIAN_POINT ( 'NONE',  ( 85.83023444425720072, 0.8841707150779518631, 5.891289308415252890 ) ) ;
#29948=CARTESIAN_POINT ( 'NONE',  ( 23.44524387940805354, 3.803759871792764091, 3.069313877683408354 ) ) ;
#29952=B_SPLINE_CURVE_WITH_KNOTS ( 'NONE', 3,
 ( #11105, #16881, #29463, #17277 ),
 .UNSPECIFIED., .F., .F.,
 ( 4, 4 ),
 ( 0.000000000000000000, 1.000000000000000000 ),
 .UNSPECIFIED. ) ;
#29956=CARTESIAN_POINT ( 'NONE',  ( 37.14378633834282795, -2.493312693697226301, 5.967573678773149481 ) ) ;
#29962=DIRECTION ( 'NONE',  ( -0.000000000000000000, 0.000000000000000000, -1.000000000000000000 ) ) ;
#29964=CARTESIAN_POINT ( 'NONE',  ( 17.36972370856863535, 14.26801361678851343, 2.499999999999999112 ) ) ;
#29965=CARTESIAN_POINT ( 'NONE',  ( 21.85643539959775694, 5.983772091205654675, 13.40455955530236487 ) ) ;
#29968=CARTESIAN_POINT ( 'NONE',  ( -81.79890681550139675, 10.46299657128043492, 0.6911394749367770762 ) ) ;
#29969=DIRECTION ( 'NONE',  ( 0.000000000000000000, 1.000000000000000000, 0.000000000000000000 ) ) ;
#29970=CARTESIAN_POINT ( 'NONE',  ( -76.50781846841695710, 9.203653447225347506, -9.788468040724580987 ) ) ;
#29971=CARTESIAN_POINT ( 'NONE',  ( 37.11062810659152689, -2.402986199528067246, -5.951436016291230757 ) ) ;
#29976=CARTESIAN_POINT ( 'NONE',  ( 31.16472951934800406, -0.3606997634973788669, 5.070407781962654958 ) ) ;
#29985=CARTESIAN_POINT ( 'NONE',  ( 34.77093152648067331, -3.235628152337162167, 5.633242821496846631 ) ) ;
#29989=CARTESIAN_POINT ( 'NONE',  ( 85.81943862418182789, 1.961257897749014045, -4.406084401447566634 ) ) ;
#29991=CARTESIAN_POINT ( 'NONE',  ( 27.43879703630890887, 0.9604363013853572939, -4.488885905966782275 ) ) ;
#30002=DIRECTION ( 'NONE',  ( 0.000000000000000000, 0.000000000000000000, 1.000000000000000000 ) ) ;
#30004=CARTESIAN_POINT ( 'NONE',  ( 23.18405951893644001, 0.8525072515736740186, 5.603743966958759870 ) ) ;
#30011=LINE ( 'NONE', #2033, #25602 ) ;
#30016=CARTESIAN_POINT ( 'NONE',  ( 22.97618870714912731, 3.739651848979420379, -3.615343062961793752 ) ) ;
#30020=CIRCLE ( 'NONE', #35315, 9.804803391925412726 ) ;
#30021=CARTESIAN_POINT ( 'NONE',  ( 22.49677218534670331, -0.6234722885575160189, 9.207484322151008982 ) ) ;
#30023=CARTESIAN_POINT ( 'NONE',  ( 21.89858680185338358, 3.819795204994611559, -2.126311674337833413 ) ) ;
#30027=CARTESIAN_POINT ( 'NONE',  ( 84.83925925549863223, 2.817044135119172399, -2.844581780382558378 ) ) ;
#30034=CARTESIAN_POINT ( 'NONE',  ( 31.38022914977189259, -3.594042512269271850, -4.917870897524577067 ) ) ;
#30035=CARTESIAN_POINT ( 'NONE',  ( 34.33233530168753589, -1.487613377254970226, -5.564789273131927949 ) ) ;
#30037=CARTESIAN_POINT ( 'NONE',  ( 22.73363516861961742, 0.4005846852146681680, -6.310066893263544863 ) ) ;
#30040=CARTESIAN_POINT ( 'NONE',  ( 36.79674047955164440, -2.557473896570829908, 5.949419303002247972 ) ) ;
#30041=VECTOR ( 'NONE', #14133, 1000.000000000000000 ) ;
#30045=CARTESIAN_POINT ( 'NONE',  ( 36.71942053932279748, -3.459622343616183038, 5.860272900448393329 ) ) ;
#30049=CARTESIAN_POINT ( 'NONE',  ( 16.12381318270590924, -3.547307913324281081, -2.701813617103016263 ) ) ;
#30051=CARTESIAN_POINT ( 'NONE',  ( 14.67325355196851255, 12.62073864644707299, -2.499999999995972111 ) ) ;
#30054=FACE_OUTER_BOUND ( 'NONE', #28537, .T. ) ;
#30059=DIRECTION ( 'NONE',  ( 1.000000000000000000, 0.000000000000000000, 0.000000000000000000 ) ) ;
#30060=ORIENTED_EDGE ( 'NONE', *, *, #14385, .F. ) ;
#30061=CARTESIAN_POINT ( 'NONE',  ( -60.15914593959029588, -52.45670913645259503, 2.307692307692319478 ) ) ;
#30064=CARTESIAN_POINT ( 'NONE',  ( 21.82594131963945827, 4.890129326492636430, 3.822364013852876496 ) ) ;
#30067=VERTEX_POINT ( 'NONE', #40589 ) ;
#30073=CARTESIAN_POINT ( 'NONE',  ( 21.83838922799100146, 2.382728257201017996, -5.693891273926298346 ) ) ;
#30082=CARTESIAN_POINT ( 'NONE',  ( 88.26779375368444391, -0.7888507896528732521, -1.681504516799547710 ) ) ;
#30083=CARTESIAN_POINT ( 'NONE',  ( 32.02118327030063227, -4.941963151977918578, 1.942379491845174444 ) ) ;
#30094=EDGE_CURVE ( 'NONE', #6701, #40686, #33090, .T. ) ;
#30095=CARTESIAN_POINT ( 'NONE',  ( 36.46945287769039368, -2.309416368423244936, -5.898338157251335367 ) ) ;
#30098=B_SPLINE_CURVE_WITH_KNOTS ( 'NONE', 3,
 ( #29991, #11033, #4874, #23611, #14331, #33303, #5083, #8354, #21345, #36576, #27518, #17615, #36177, #36981, #8763, #20505, #33089, #26902, #11235, #30194, #2014, #21557, #25255, #28123, #8972, #27713, #18861, #15571, #31229, #15156, #5905, #40678, #25052, #3458, #3051, #31636, #2636, #18444, #40266, #15359, #31031, #2838, #22175, #31434, #27915, #9381, #12482, #40461, #6312, #37584, #21967, #34539, #12051, #24630 ),
 .UNSPECIFIED., .F., .F.,
 ( 4, 1, 1, 1, 2, 2, 1, 1, 1, 1, 1, 1, 2, 2, 1, 1, 1, 1, 1, 1, 1, 1, 2, 2, 1, 1, 1, 1, 2, 2, 1, 1, 1, 1, 1, 2, 2, 1, 1, 1, 1, 4 ),
 ( 0.3081789993805284511, 0.4811342495358507110, 0.4919439526705583487, 0.4973488042379122787, 0.4987000171297506501, 0.5000512300215890216, 0.5027536558052657645, 0.5243730620746801518, 0.5676118746135082604, 0.6108506871523364801, 0.6216603902870434517, 0.6243628160707210828, 0.6247006192936801483, 0.6250384225166392138, 0.6257140289625566787, 0.6270652418543913864, 0.6324700934217306614, 0.6540894996910853187, 0.7405671247685048364, 0.7459719763358438893, 0.7486744021195133048, 0.7493500085654295484, 0.7496878117883878367, 0.7500256150113457920, 0.7513768279031767250, 0.7621865310378237446, 0.7838059373071175617, 0.8054253435764113789, 0.8108301951437346666, 0.8135326209273960885, 0.8162350467110577323, 0.8270447498457029756, 0.8702835623842855028, 0.8729859881679464806, 0.8743372010597769695, 0.8746750042827347027, 0.8750128075056922139, 0.8756884139516074583, 0.8810932655189296359, 0.8919029686535726587, 0.9135223749228589263, 1.000000000000000000 ),
 .UNSPECIFIED. ) ;
#30102=CARTESIAN_POINT ( 'NONE',  ( 35.56290024310237641, -1.640810893426935646, 5.744602770279306547 ) ) ;
#30115=CARTESIAN_POINT ( 'NONE',  ( 21.83113904852917031, 5.958251073797080188, 3.138007096634494619 ) ) ;
#30118=CARTESIAN_POINT ( 'NONE',  ( 24.20404138067665656, -8.556376197523151816, -2.500000000000003997 ) ) ;
#30121=CARTESIAN_POINT ( 'NONE',  ( 24.74193054586557139, 0.5345309101367632376, 4.782337473183671861 ) ) ;
#30128=CARTESIAN_POINT ( 'NONE',  ( 66.41194937274630661, -13.65448019739280028, -6.000000000000000000 ) ) ;
#30129=CARTESIAN_POINT ( 'NONE',  ( 24.23947115566313926, 0.8503125907183233245, 6.739520400040675874 ) ) ;
#30130=CYLINDRICAL_SURFACE ( 'NONE', #28651, 1.000000000000000888 ) ;
#30132=ORIENTED_EDGE ( 'NONE', *, *, #34324, .T. ) ;
#30133=CARTESIAN_POINT ( 'NONE',  ( -80.93488167894386720, -6.594418668544227202, -0.1886647716054447033 ) ) ;
#30134=CARTESIAN_POINT ( 'NONE',  ( 24.12180912460078730, 0.4861797095442714767, -5.096561526129780972 ) ) ;
#30139=CARTESIAN_POINT ( 'NONE',  ( 34.63540570288399323, -0.7851885325132845761, -5.278762693032814646 ) ) ;
#30143=LINE ( 'NONE', #14477, #37669 ) ;
#30145=CARTESIAN_POINT ( 'NONE',  ( -72.99783146927553901, 4.029110416273074868, 10.94627121662267122 ) ) ;
#30146=VECTOR ( 'NONE', #34277, 1000.000000000000000 ) ;
#30152=CARTESIAN_POINT ( 'NONE',  ( 86.92455237868826146, -1.249784692553891574, -5.093375875629621241 ) ) ;
#30162=CARTESIAN_POINT ( 'NONE',  ( 16.61473287052537273, 9.888383995183708919, -2.499999999999976019 ) ) ;
#30166=CARTESIAN_POINT ( 'NONE',  ( 22.63566524836003069, 3.890655838760145979, 3.739241026276091340 ) ) ;
#30167=CARTESIAN_POINT ( 'NONE',  ( -72.42837670882107659, -47.11702805680359063, 5.809475019311127753 ) ) ;
#30168=CARTESIAN_POINT ( 'NONE',  ( 18.53067622772632461, 13.20527538885293062, 2.499999999999999556 ) ) ;
#30169=CARTESIAN_POINT ( 'NONE',  ( 21.85643539959774984, 9.043776176932434296, -7.298091200098202336 ) ) ;
#30170=ORIENTED_EDGE ( 'NONE', *, *, #12314, .F. ) ;
#30171=CARTESIAN_POINT ( 'NONE',  ( -80.19809822935498289, 11.50978792661036998, 3.773274132804689263 ) ) ;
#30172=CARTESIAN_POINT ( 'NONE',  ( 14.74178471286434622, -5.124043802339638631, 2.500000000000000444 ) ) ;
#30173=CARTESIAN_POINT ( 'NONE',  ( -73.70430257933739426, 6.071219537989406057, -10.84014157372769382 ) ) ;
#30180=FACE_OUTER_BOUND ( 'NONE', #26964, .T. ) ;
#30187=CARTESIAN_POINT ( 'NONE',  ( 37.04435200418730290, -2.893112835670054395, 5.988065069928986794 ) ) ;
#30192=CARTESIAN_POINT ( 'NONE',  ( 88.43294427370824451, -0.9743556922601576131, -2.623293804462837553 ) ) ;
#30193=CARTESIAN_POINT ( 'NONE',  ( 33.80908501075300165, -4.930824710404003497, 3.361253013157701197 ) ) ;
#30194=CARTESIAN_POINT ( 'NONE',  ( 33.64208751344185089, -1.232828649894890605, -5.457059412070498716 ) ) ;
#30208=CARTESIAN_POINT ( 'NONE',  ( 23.17509331881612056, 0.5418487631251007741, 5.782618900065904732 ) ) ;
#30215=CARTESIAN_POINT ( 'NONE',  ( 14.69558838330753758, 3.996311804371543985, -6.000000000000000000 ) ) ;
#30220=CARTESIAN_POINT ( 'NONE',  ( 22.92659693992655079, 4.107476889741620951, -3.299805457877865056 ) ) ;
#30225=CARTESIAN_POINT ( 'NONE',  ( 22.32844273176644379, 5.552903595841022444, -4.279453667248723114 ) ) ;
#30231=CARTESIAN_POINT ( 'NONE',  ( 86.57035376367728929, -0.007661497531101129840, -5.962853773335548446 ) ) ;
#30233=VERTEX_POINT ( 'NONE', #19584 ) ;
#30237=CARTESIAN_POINT ( 'NONE',  ( 16.05059429624258271, -3.466255778341811755, -2.706403111257027039 ) ) ;
#30238=CARTESIAN_POINT ( 'NONE',  ( 33.68724495179844070, -3.100361039176545486, -5.464107322465908467 ) ) ;
#30240=CARTESIAN_POINT ( 'NONE',  ( 24.69561352525090214, 0.6721404258068209847, -4.790969045266487036 ) ) ;
#30241=CARTESIAN_POINT ( 'NONE',  ( 29.95669672263519701, -3.739584766489346013, -4.529080000040674570 ) ) ;
#30242=ORIENTED_EDGE ( 'NONE', *, *, #38245, .F. ) ;
#30243=CARTESIAN_POINT ( 'NONE',  ( 22.91740499742190096, 2.643278788709220617, 3.783213328018341759 ) ) ;
#30245=CARTESIAN_POINT ( 'NONE',  ( 32.03825560683729634, -2.979144026594910066, -5.206742654223620370 ) ) ;
#30247=EDGE_LOOP ( 'NONE', ( #8663, #15430 ) ) ;
#30248=CARTESIAN_POINT ( 'NONE',  ( 34.63832540556266792, -0.7796590688174727113, 5.272668787675296009 ) ) ;
#30250=CARTESIAN_POINT ( 'NONE',  ( 14.61802081865033642, 12.33286846116284252, -2.500000000000000000 ) ) ;
#30253=DIRECTION ( 'NONE',  ( -0.000000000000000000, 0.000000000000000000, -1.000000000000000000 ) ) ;
#30256=EDGE_LOOP ( 'NONE', ( #36586, #25475 ) ) ;
#30260=ORIENTED_EDGE ( 'NONE', *, *, #15774, .T. ) ;
#30262=ORIENTED_EDGE ( 'NONE', *, *, #14631, .T. ) ;
#30263=CARTESIAN_POINT ( 'NONE',  ( 22.71203523026179028, 4.249011684457585147, 3.358792741310332008 ) ) ;
#30272=FACE_OUTER_BOUND ( 'NONE', #18290, .T. ) ;
#30274=CARTESIAN_POINT ( 'NONE',  ( 22.49685282670636255, 2.447218780948473782, -4.963950670329193571 ) ) ;
#30276=CARTESIAN_POINT ( 'NONE',  ( -12.99139449055068241, 13.37661300689600097, 2.500000000000000000 ) ) ;
#30280=CARTESIAN_POINT ( 'NONE',  ( 88.23268491810016201, -0.7494148791586221492, 1.919551801057179263 ) ) ;
#30281=CARTESIAN_POINT ( 'NONE',  ( 33.90241230359465874, -5.503808810968542353, 0.4955917775451662566 ) ) ;
#30284=CARTESIAN_POINT ( 'NONE',  ( 18.28173501743642859, -3.120125090614966012, 3.013464740560008348 ) ) ;
#30286=CARTESIAN_POINT ( 'NONE',  ( 34.12754808946520058, -3.289252972442476164, -5.532827275885577656 ) ) ;
#30294=CARTESIAN_POINT ( 'NONE',  ( -69.62739392171840791, -46.36406956038555194, 5.857517722768268875 ) ) ;
#30297=CARTESIAN_POINT ( 'NONE',  ( 37.15955769875629500, -2.950428308811992029, 5.999626784867526652 ) ) ;
#30301=CARTESIAN_POINT ( 'NONE',  ( -71.19065411851930492, 0.1907566484747143243, 9.997285688091771760 ) ) ;
#30302=DIRECTION ( 'NONE',  ( 0.000000000000000000, -0.000000000000000000, -1.000000000000000000 ) ) ;
#30304=DIRECTION ( 'NONE',  ( 1.000000000000000000, 0.000000000000000000, 0.000000000000000000 ) ) ;
#30305=EDGE_CURVE ( 'NONE', #16957, #12163, #10620, .T. ) ;
#30307=CARTESIAN_POINT ( 'NONE',  ( 14.77222812468937363, 12.33286846116137347, 2.511961485181785747 ) ) ;
#30308=CARTESIAN_POINT ( 'NONE',  ( -80.31292318400757324, 11.50538633170450176, 3.479145684545672523 ) ) ;
#30312=CARTESIAN_POINT ( 'NONE',  ( 22.18671130633063271, 5.268486589209644855, 3.076124624071696623 ) ) ;
#30320=ORIENTED_EDGE ( 'NONE', *, *, #24370, .T. ) ;
#30323=CARTESIAN_POINT ( 'NONE',  ( 24.74514331060581185, 0.5825920455569916223, 4.777508842034277059 ) ) ;
#30324=CARTESIAN_POINT ( 'NONE',  ( 14.66195011488853517, -4.891470949017669767, -2.500000000000007550 ) ) ;
#30329=B_SPLINE_CURVE_WITH_KNOTS ( 'NONE', 3,
 ( #28142, #3072, #40696, #18049, #12074, #21985, #34561, #30641, #6331, #25273, #2449, #24651, #8992, #18882, #31452, #19289, #38213, #32270, #7135, #28560, #19086, #10010, #31656 ),
 .UNSPECIFIED., .F., .F.,
 ( 4, 2, 2, 2, 1, 2, 2, 1, 2, 2, 1, 2, 4 ),
 ( 0.000000000000000000, 0.1556967518389709704, 0.2335451277584564278, 0.2530072217383279587, 0.2724693157181994896, 0.3113935036779426069, 0.4670902555169128001, 0.4865523494967844975, 0.4962833964867204295, 0.5011489199816884232, 0.5060144434766563615, 0.5449386314364057515, 0.6227870073559045316 ),
 .UNSPECIFIED. ) ;
#30334=CARTESIAN_POINT ( 'NONE',  ( 14.69558838330753758, 3.996311804371543985, -6.000000000000000000 ) ) ;
#30335=CARTESIAN_POINT ( 'NONE',  ( 28.43092716748534343, -1.248584762127236569, 6.041969456467763955 ) ) ;
#30340=CARTESIAN_POINT ( 'NONE',  ( 22.61176954047653709, 0.2940635019282091256, -6.499681003685747527 ) ) ;
#30346=CARTESIAN_POINT ( 'NONE',  ( -72.23853693793628850, -47.87307048379776120, 9.914091297619886944 ) ) ;
#30347=CARTESIAN_POINT ( 'NONE',  ( 37.10367516289256429, -3.125626235160924526, -5.976315389033000081 ) ) ;
#30356=CARTESIAN_POINT ( 'NONE',  ( 24.14678853894412214, 1.668812993869833283, -4.589722933970846519 ) ) ;
#30357=ORIENTED_EDGE ( 'NONE', *, *, #16861, .T. ) ;
#30358=CARTESIAN_POINT ( 'NONE',  ( -70.00483706461088218, -48.31492315352122802, 5.930144077445180351 ) ) ;
#30361=ORIENTED_EDGE ( 'NONE', *, *, #1296, .F. ) ;
#30373=CARTESIAN_POINT ( 'NONE',  ( 22.38977015051906250, -3.087247959475952541, 3.600891321702764269 ) ) ;
#30383=CARTESIAN_POINT ( 'NONE',  ( 17.44014759849567398, 14.20845974933103051, 2.500000000000000444 ) ) ;
#30384=CARTESIAN_POINT ( 'NONE',  ( 21.85643539959773207, -2.491245572580281564, -14.29094192267194607 ) ) ;
#30386=CARTESIAN_POINT ( 'NONE',  ( -80.70858810156305196, 11.48226577419836225, 2.235992612072733365 ) ) ;
#30387=CARTESIAN_POINT ( 'NONE',  ( 14.74659717070468723, -5.121692793854265346, 2.499999999975831333 ) ) ;
#30388=CARTESIAN_POINT ( 'NONE',  ( -74.02042637766889754, 8.682579473379398394, -9.514814749544530770 ) ) ;
#30390=CARTESIAN_POINT ( 'NONE',  ( 35.36840502023477484, -3.795127586234050110, -5.508707976554834573 ) ) ;
#30392=CARTESIAN_POINT ( 'NONE',  ( 14.82426946740453921, 12.80491062889915099, 2.505159076423423503 ) ) ;
#30394=CARTESIAN_POINT ( 'NONE',  ( -69.95448302925287010, -0.5208875146770525211, 9.952591258774150518 ) ) ;
#30402=CARTESIAN_POINT ( 'NONE',  ( 25.29913702416237342, 1.743601996224051431, 4.154940213198440091 ) ) ;
#30403=CARTESIAN_POINT ( 'NONE',  ( 84.57067941792149668, 3.126724152278200997, 0.3173792860121260051 ) ) ;
#30407=CARTESIAN_POINT ( 'NONE',  ( -69.92837670882106238, -20.91541721511087815, 5.916079783099611689 ) ) ;
#30412=ADVANCED_FACE ( 'NONE', ( #32280 ), #16594, .T. ) ;
#30417=CARTESIAN_POINT ( 'NONE',  ( 23.10229947436055298, 0.3735801593563349843, 5.909219875391088728 ) ) ;
#30428=CARTESIAN_POINT ( 'NONE',  ( 22.89526542370903073, 4.247657506257562332, -3.165813468130866948 ) ) ;
#30431=CARTESIAN_POINT ( 'NONE',  ( 23.92067639343244778, 4.177307434159622801, 1.236145424036337426 ) ) ;
#30433=DIRECTION ( 'NONE',  ( 1.000000000000000000, 8.959828616340678715E-16, 0.000000000000000000 ) ) ;
#30435=CARTESIAN_POINT ( 'NONE',  ( 85.74309555164268204, 1.026708856660649705, -5.825338620068188256 ) ) ;
#30438=DIRECTION ( 'NONE',  ( -7.232507224765808510E-18, 1.000000000000000000, 0.000000000000000000 ) ) ;
#30441=CARTESIAN_POINT ( 'NONE',  ( 19.68627602041497582, -2.909546155338069262, -3.262843111110074190 ) ) ;
#30443=FACE_OUTER_BOUND ( 'NONE', #35916, .T. ) ;
#30447=VERTEX_POINT ( 'NONE', #8127 ) ;
#30448=CARTESIAN_POINT ( 'NONE',  ( 34.77322202883802760, -3.158692642683334384, 5.633600309789820848 ) ) ;
#30451=CARTESIAN_POINT ( 'NONE',  ( 87.55151927672237377, 0.01570269930849589254, 4.249584817138070569 ) ) ;
#30455=CARTESIAN_POINT ( 'NONE',  ( 20.92045951437903994, 4.581793376609706314, 2.649698315330352827 ) ) ;
#30456=CARTESIAN_POINT ( 'NONE',  ( -69.46781065323600046, -47.51068050472974136, 9.893050960843961406 ) ) ;
#30458=CARTESIAN_POINT ( 'NONE',  ( 14.77222812468926705, 12.33286846116276614, -2.511961485181769316 ) ) ;
#30459=ORIENTED_EDGE ( 'NONE', *, *, #38760, .F. ) ;
#30469=CARTESIAN_POINT ( 'NONE',  ( -62.92837670882109080, -52.49535338866469658, 6.000000000000000000 ) ) ;
#30472=CARTESIAN_POINT ( 'NONE',  ( 22.76958335768329178, 3.831392003152646275, 3.677966780943355385 ) ) ;
#30478=CARTESIAN_POINT ( 'NONE',  ( 20.90243674393227025, -2.659970222288498665, -3.468728799870355317 ) ) ;
#30482=CARTESIAN_POINT ( 'NONE',  ( 22.43736279192665961, 3.331640513653970181, -4.315273480065289213 ) ) ;
#30484=DIRECTION ( 'NONE',  ( -5.786005779812646808E-17, 1.000000000000000000, 0.000000000000000000 ) ) ;
#30489=CARTESIAN_POINT ( 'NONE',  ( 85.14289959633329374, 2.721178644307868044, -0.4516327360412458747 ) ) ;
#30493=CARTESIAN_POINT ( 'NONE',  ( 26.28542322345758819, -3.293173076614191785, 4.155233155835949432 ) ) ;
#30497=CARTESIAN_POINT ( 'NONE',  ( 21.25657147360305288, 3.328712036232781557, -3.524000089216284159 ) ) ;
#30507=CARTESIAN_POINT ( 'NONE',  ( 35.36787417293467684, -3.789710888759190155, 5.512881233678236015 ) ) ;
#30510=FACE_BOUND ( 'NONE', #12532, .T. ) ;
#30516=EDGE_LOOP ( 'NONE', ( #9833, #28753, #33665, #564 ) ) ;
#30517=FACE_OUTER_BOUND ( 'NONE', #2255, .T. ) ;
#30520=CARTESIAN_POINT ( 'NONE',  ( 24.02218326506362089, 3.317473792240205999, 3.324804558572830526 ) ) ;
#30523=AXIS2_PLACEMENT_3D ( 'NONE', #5189, #17720, #30304 ) ;
#30524=AXIS2_PLACEMENT_3D ( 'NONE', #38865, #29416, #10656 ) ;
#30528=CARTESIAN_POINT ( 'NONE',  ( 22.60590637795996116, 0.2865873366347984619, 6.509088009623860138 ) ) ;
#30529=CARTESIAN_POINT ( 'NONE',  ( 14.68777614925489772, -4.612119195195942822, -2.500000000000232259 ) ) ;
#30534=CARTESIAN_POINT ( 'NONE',  ( 36.29481586213307764, -3.617251867669180498, -5.744675751259891605 ) ) ;
#30539=CARTESIAN_POINT ( 'NONE',  ( 37.83867290611771494, -6.084034091406928191, 6.000000000000000000 ) ) ;
#30540=CARTESIAN_POINT ( 'NONE',  ( 29.93139500891458127, 0.4880113553092989553, -5.118255730029571460 ) ) ;
#30550=CARTESIAN_POINT ( 'NONE',  ( -71.02745642956452343, -48.61702805680358352, 10.00000000000001066 ) ) ;
#30552=CARTESIAN_POINT ( 'NONE',  ( 30.88168762873399587, 0.6966114428816204684, -4.496783944086453211 ) ) ;
#30553=CARTESIAN_POINT ( 'NONE',  ( 30.88127119532873976, -3.422338893432233853, -4.937978149253780202 ) ) ;
#30554=CARTESIAN_POINT ( 'NONE',  ( 53.63097637064826273, -5.819101496702492327, -6.000000000000000888 ) ) ;
#30559=EDGE_CURVE ( 'NONE', #35445, #15320, #25440, .T. ) ;
#30562=CARTESIAN_POINT ( 'NONE',  ( 14.77500326541903952, -5.175625724643098557, -2.499997102511863911 ) ) ;
#30563=CARTESIAN_POINT ( 'NONE',  ( 24.36356524659568024, 2.395873619741290206, -4.116030573549343430 ) ) ;
#30565=ORIENTED_EDGE ( 'NONE', *, *, #20110, .T. ) ;
#30571=CARTESIAN_POINT ( 'NONE',  ( 85.92174427069515730, 0.4035765525155806666, 6.008818417626160979 ) ) ;
#30583=VERTEX_POINT ( 'NONE', #12460 ) ;
#30585=CARTESIAN_POINT ( 'NONE',  ( 15.99304537737771703, 7.920163261466188764, -3.484773916741529476 ) ) ;
#30590=CARTESIAN_POINT ( 'NONE',  ( 23.53282518156592573, 3.062426620546339073, 3.879264531747849354 ) ) ;
#30593=ORIENTED_EDGE ( 'NONE', *, *, #34749, .F. ) ;
#30594=CARTESIAN_POINT ( 'NONE',  ( 21.85643539959774273, 9.172641120068929510, -1.679843024921975347 ) ) ;
#30596=CARTESIAN_POINT ( 'NONE',  ( -80.58817961249317818, 10.50547908170135791, 5.356801284506212291 ) ) ;
#30598=CIRCLE ( 'NONE', #3670, 0.9999999999999991118 ) ;
#30600=CARTESIAN_POINT ( 'NONE',  ( -76.08100811359271631, 8.922477016430406138, -8.599497118620481828 ) ) ;
#30604=CARTESIAN_POINT ( 'NONE',  ( 14.86299874107311325, 12.06992840946315937, 2.526128435164121111 ) ) ;
#30610=CARTESIAN_POINT ( 'NONE',  ( -70.92837670882107659, -23.80776546975053520, -10.00000000000000533 ) ) ;
#30612=EDGE_CURVE ( 'NONE', #4540, #3011, #4438, .T. ) ;
#30613=CARTESIAN_POINT ( 'NONE',  ( 25.67085356133009810, 2.140750286663625879, -4.140177559339564439 ) ) ;
#30616=CARTESIAN_POINT ( 'NONE',  ( 35.45469368754801565, -1.911696930450387688, 5.739960443585752969 ) ) ;
#30620=AXIS2_PLACEMENT_3D ( 'NONE', #11740, #14436, #24318 ) ;
#30621=CARTESIAN_POINT ( 'NONE',  ( 88.31640312351544253, -1.506181138579067103, 3.771763452802144201 ) ) ;
#30622=CARTESIAN_POINT ( 'NONE',  ( 33.69128717328723610, -4.440785898112559416, 4.348130384999381981 ) ) ;
#30627=CARTESIAN_POINT ( 'NONE',  ( 86.05684172526336795, 1.348548140555935193, 5.632715373612032117 ) ) ;
#30633=CARTESIAN_POINT ( 'NONE',  ( 87.04213330793400871, 0.5878691963681514920, -4.891134986362597914 ) ) ;
#30635=CARTESIAN_POINT ( 'NONE',  ( 21.81854301884185432, 0.2747606569782626851, 8.209505977014627476 ) ) ;
#30641=CARTESIAN_POINT ( 'NONE',  ( 24.97205702378243330, -5.748183807572947224, 2.896408662958795066 ) ) ;
#30642=CYLINDRICAL_SURFACE ( 'NONE', #36670, 7.744449365083023729 ) ;
#30643=CARTESIAN_POINT ( 'NONE',  ( 24.69630075600026231, 2.999063368822487252, -3.452992298664733006 ) ) ;
#30646=AXIS2_PLACEMENT_3D ( 'NONE', #40662, #34520, #6297 ) ;
#30648=CARTESIAN_POINT ( 'NONE',  ( 21.82633783062472688, 5.573671403123425350, 3.484773800359227014 ) ) ;
#30651=CARTESIAN_POINT ( 'NONE',  ( 84.34456690318765482, 2.887654542466673746, -2.101772343363317752 ) ) ;
#30652=CARTESIAN_POINT ( 'NONE',  ( 17.34292908646689568, 9.186004740436843008, 2.849848300167282744 ) ) ;
#30656=ORIENTED_EDGE ( 'NONE', *, *, #3110, .F. ) ;
#30657=FACE_OUTER_BOUND ( 'NONE', #24690, .T. ) ;
#30658=CARTESIAN_POINT ( 'NONE',  ( 14.73050576274141932, -5.057416755502635475, -2.496373688475125974 ) ) ;
#30659=ADVANCED_FACE ( 'NONE', ( #327 ), #31198, .T. ) ;
#30660=CARTESIAN_POINT ( 'NONE',  ( 31.71708122509442873, -0.5641260517970680954, -5.156615624320846969 ) ) ;
#30661=CARTESIAN_POINT ( 'NONE',  ( 1.700390093233090871, -29.56993018339339940, -6.000000000000001776 ) ) ;
#30664=CARTESIAN_POINT ( 'NONE',  ( 34.77318038334062322, -3.160091470131585645, 5.633593810002675006 ) ) ;
#30665=CARTESIAN_POINT ( 'NONE',  ( -17.69482985384421880, -42.37473357531882101, 6.000000000000000000 ) ) ;
#30666=ORIENTED_EDGE ( 'NONE', *, *, #22009, .F. ) ;
#30669=CARTESIAN_POINT ( 'NONE',  ( 37.18695530022691287, -2.963565836837915413, 6.000026294647724079 ) ) ;
#30671=B_SPLINE_CURVE_WITH_KNOTS ( 'NONE', 3,
 ( #19816, #35483, #495, #22521, #25594, #13232, #891, #29289, #35089, #20011, #19622, #31780, #22720, #22913, #13637, #10535, #13030, #13427, #9938, #6863, #6664, #26002, #31990, #1105 ),
 .UNSPECIFIED., .F., .F.,
 ( 4, 1, 1, 1, 1, 1, 1, 2, 2, 1, 1, 1, 1, 1, 1, 2, 2, 4 ),
 ( 0.000000000000000000, 0.2500000000000391354, 0.3750000000000583422, 0.4375000000000676681, 0.4687500000000721645, 0.4843750000000747735, 0.4921875000000763833, 0.4960937500000768829, 0.5000000000000773825, 0.6250000000000768274, 0.6875000000000761613, 0.7187500000000758282, 0.7343750000000756062, 0.7421875000000754952, 0.7460937500000754952, 0.7480468750000754952, 0.7500000000000753841, 1.000000000000000000 ),
 .UNSPECIFIED. ) ;
#30672=CARTESIAN_POINT ( 'NONE',  ( 15.01265474174107162, -4.182841212154375654, -2.538985411732104236 ) ) ;
#30673=CARTESIAN_POINT ( 'NONE',  ( 14.72830186849878942, 12.61371249419844176, -2.505105730542713349 ) ) ;
#30677=ORIENTED_EDGE ( 'NONE', *, *, #24881, .T. ) ;
#30684=CARTESIAN_POINT ( 'NONE',  ( 23.87849444185487258, 2.668685871580891877, 4.066325986815254367 ) ) ;
#30685=CARTESIAN_POINT ( 'NONE',  ( 14.73750015949773484, 12.90700633731061409, 2.501527175807433334 ) ) ;
#30691=CARTESIAN_POINT ( 'NONE',  ( 26.95243645308021385, -2.795055227801056308, -4.412977574278784232 ) ) ;
#30694=CARTESIAN_POINT ( 'NONE',  ( 23.69828321319373288, 3.038820287558408051, -3.842211770153025174 ) ) ;
#30698=CARTESIAN_POINT ( 'NONE',  ( 21.85643539959777826, -13.51165962708896728, -8.254727072381385256 ) ) ;
#30699=DIRECTION ( 'NONE',  ( 0.000000000000000000, -1.000000000000000000, -0.000000000000000000 ) ) ;
#30704=CARTESIAN_POINT ( 'NONE',  ( 88.52897200822518187, -1.082218601420786186, 0.1993289098281435523 ) ) ;
#30707=CARTESIAN_POINT ( 'NONE',  ( 18.27718096362622546, -3.093593596032681248, 3.021173953333614826 ) ) ;
#30709=CARTESIAN_POINT ( 'NONE',  ( -16.27783086239806210, 25.90100547710869705, 2.500000000000000000 ) ) ;
#30711=CARTESIAN_POINT ( 'NONE',  ( 37.04663327496000846, -2.800723657629412777, -5.988421117405737348 ) ) ;
#30716=VECTOR ( 'NONE', #26210, 1000.000000000000000 ) ;
#30718=CARTESIAN_POINT ( 'NONE',  ( -69.73579169773952913, -46.20201783773000415, 5.880545134273299723 ) ) ;
#30720=CARTESIAN_POINT ( 'NONE',  ( 36.10471242579632190, -1.581987752735663166, 5.680909380111648588 ) ) ;
#30725=DIRECTION ( 'NONE',  ( 0.000000000000000000, 1.000000000000000000, 0.000000000000000000 ) ) ;
#30728=CARTESIAN_POINT ( 'NONE',  ( -80.88560043480099182, -6.600306782100017422, -1.015383303423792460 ) ) ;
#30730=ORIENTED_EDGE ( 'NONE', *, *, #15054, .T. ) ;
#30733=ORIENTED_EDGE ( 'NONE', *, *, #6102, .T. ) ;
#30734=CARTESIAN_POINT ( 'NONE',  ( 23.42568583973897844, 3.752714481185509765, 3.194445122559177452 ) ) ;
#30741=CARTESIAN_POINT ( 'NONE',  ( 22.28825410457798384, 0.2534056759817530091, 7.122325049175724843 ) ) ;
#30742=CARTESIAN_POINT ( 'NONE',  ( 14.76691882379872034, -5.164572653182437634, -2.499999999999999556 ) ) ;
#30744=AXIS2_PLACEMENT_3D ( 'NONE', #35448, #9485, #3553 ) ;
#30756=CARTESIAN_POINT ( 'NONE',  ( 29.97449823033972649, -1.245471885678776980, 6.039028575696650414 ) ) ;
#30758=CARTESIAN_POINT ( 'NONE',  ( -62.92837670882106238, 3.729367930467588632, -6.000000000000000000 ) ) ;
#30762=CARTESIAN_POINT ( 'NONE',  ( -18.27651686900387418, -64.04014080848075707, 2.500000000000000000 ) ) ;
#30766=CARTESIAN_POINT ( 'NONE',  ( 36.65987745959532162, -1.958086723934334694, -5.826241878318064060 ) ) ;
#30775=CARTESIAN_POINT ( 'NONE',  ( 23.40345427751441321, 1.751723352111926424, -4.892213115278092772 ) ) ;
#30777=CARTESIAN_POINT ( 'NONE',  ( 14.61802081865033820, -4.461849342347350422, 2.500000000000000000 ) ) ;
#30781=ORIENTED_EDGE ( 'NONE', *, *, #19818, .F. ) ;
#30788=LINE ( 'NONE', #8520, #1509 ) ;
#30790=CARTESIAN_POINT ( 'NONE',  ( 24.07321278147298926, 3.353042105641798720, 3.188969774653739986 ) ) ;
#30791=EDGE_CURVE ( 'NONE', #2537, #30233, #851, .T. ) ;
#30799=AXIS2_PLACEMENT_3D ( 'NONE', #3291, #9626, #35178 ) ;
#30803=CARTESIAN_POINT ( 'NONE',  ( 21.85643539959778181, 8.766930670454163632, 4.215001190429523703 ) ) ;
#30809=CARTESIAN_POINT ( 'NONE',  ( -74.79361657344986725, 7.703038357672896019, -10.55606559225674879 ) ) ;
#30810=DIRECTION ( 'NONE',  ( 0.000000000000000000, -0.000000000000000000, -1.000000000000000000 ) ) ;
#30811=CARTESIAN_POINT ( 'NONE',  ( 35.73144206629780228, -1.302429614601412711, -5.536403668628991248 ) ) ;
#30813=CARTESIAN_POINT ( 'NONE',  ( 14.83438443416239316, 12.32204325522479138, 2.521662480531097206 ) ) ;
#30817=CARTESIAN_POINT ( 'NONE',  ( 18.48160911996360056, 13.25447782660471852, -2.499999999999999556 ) ) ;
#30819=CARTESIAN_POINT ( 'NONE',  ( 24.71965336222647736, 2.638756212794581835, -3.924200964849605011 ) ) ;
#30822=CARTESIAN_POINT ( 'NONE',  ( 33.65798956961368305, -1.144971352236924922, 5.459541312528853219 ) ) ;
#30826=CARTESIAN_POINT ( 'NONE',  ( 86.19964454037233281, 1.163379821962233107, 5.771090254565081068 ) ) ;
#30827=CARTESIAN_POINT ( 'NONE',  ( -71.54227241695252815, -21.58327309683471995, 5.969247584478902802 ) ) ;
#30835=ORIENTED_EDGE ( 'NONE', *, *, #40287, .T. ) ;
#30851=CARTESIAN_POINT ( 'NONE',  ( 22.20701262861088310, 5.183280470103047932, -3.129361004166391069 ) ) ;
#30854=CARTESIAN_POINT ( 'NONE',  ( 26.59415400691353071, 2.826550869980146707, -2.084159418869949043 ) ) ;
#30858=CARTESIAN_POINT ( 'NONE',  ( 86.28404140065768502, 0.1054103399587360407, 6.008803426180587159 ) ) ;
#30859=CARTESIAN_POINT ( 'NONE',  ( 21.78047190118184773, 5.616103730238553027, 3.473245441588607374 ) ) ;
#30866=CARTESIAN_POINT ( 'NONE',  ( 33.96709741332558252, -3.701672533693765921, -5.338239117359374397 ) ) ;
#30870=CARTESIAN_POINT ( 'NONE',  ( 36.14147691053851474, -3.141484228563025116, 5.847149575448376879 ) ) ;
#30872=DIRECTION ( 'NONE',  ( -0.000000000000000000, -0.000000000000000000, -1.000000000000000000 ) ) ;
#30875=ORIENTED_EDGE ( 'NONE', *, *, #29784, .F. ) ;
#30877=CARTESIAN_POINT ( 'NONE',  ( 35.36839093531861522, -3.794034914966402106, 5.509564447435172596 ) ) ;
#30878=CARTESIAN_POINT ( 'NONE',  ( 19.07693085987039439, -3.073520552340138767, -3.127448232901508085 ) ) ;
#30879=CARTESIAN_POINT ( 'NONE',  ( 14.61802081865033465, 12.33286846116284252, -2.500000000000000000 ) ) ;
#30887=CARTESIAN_POINT ( 'NONE',  ( 23.18504663067065863, 2.575852116297360883, 4.415027062329348162 ) ) ;
#30888=CARTESIAN_POINT ( 'NONE',  ( 20.70168030145549309, 10.21427254645072402, -2.500000000000002220 ) ) ;
#30900=CARTESIAN_POINT ( 'NONE',  ( 22.82378969653115419, 3.379723621962007929, -4.000272552100319956 ) ) ;
#30901=EDGE_LOOP ( 'NONE', ( #39192, #24240, #13380, #40375 ) ) ;
#30902=CARTESIAN_POINT ( 'NONE',  ( 21.85643539959780313, 0.4758835581198413989, -14.20546615820951963 ) ) ;
#30904=CARTESIAN_POINT ( 'NONE',  ( 16.12938719714403746, 15.26369590458471315, -1.887449634882855110 ) ) ;
#30908=CARTESIAN_POINT ( 'NONE',  ( 85.56873805237422914, 2.242856678970356565, 3.827793690346343869 ) ) ;
#30909=CARTESIAN_POINT ( 'NONE',  ( 11.29080664838499182, -35.94265729135299381, 6.000000000000000000 ) ) ;
#30912=CARTESIAN_POINT ( 'NONE',  ( 26.28072973217529906, -3.205359020229657574, 4.210232032756980658 ) ) ;
#30914=CARTESIAN_POINT ( 'NONE',  ( 34.93036046862505373, -1.707846917307844770, -5.658125563726033924 ) ) ;
#30917=FACE_OUTER_BOUND ( 'NONE', #17061, .T. ) ;
#30921=CARTESIAN_POINT ( 'NONE',  ( -69.93716145283299568, -45.98695738452880732, 5.917975389153444787 ) ) ;
#30923=CARTESIAN_POINT ( 'NONE',  ( 33.04854646635354243, -0.2660208435476467681, 5.100183431173213044 ) ) ;
#30934=ORIENTED_EDGE ( 'NONE', *, *, #27200, .T. ) ;
#30935=CARTESIAN_POINT ( 'NONE',  ( -7.890026461918812295, -8.913725925455491250, 6.000000000000000000 ) ) ;
#30938=CARTESIAN_POINT ( 'NONE',  ( 21.73371426548433050, 6.130834824796253635, 3.264951269434681613 ) ) ;
#30943=ORIENTED_EDGE ( 'NONE', *, *, #28738, .F. ) ;
#30957=CARTESIAN_POINT ( 'NONE',  ( 33.73883514186113075, -4.630787605642836091, -3.992050560354765576 ) ) ;
#30961=CARTESIAN_POINT ( 'NONE',  ( 21.80351395196640141, 0.2459331218041709566, -8.291272508738018132 ) ) ;
#30966=CARTESIAN_POINT ( 'NONE',  ( 27.78116730204126839, 1.798541041528136653, -4.024397514413323051 ) ) ;
#30967=CARTESIAN_POINT ( 'NONE',  ( 30.88935601760522687, -3.446417099803610551, -4.925634463943371344 ) ) ;
#30974=CARTESIAN_POINT ( 'NONE',  ( 8.290806648384990041, 0.000000000000000000, 6.000000000000000000 ) ) ;
#30975=CARTESIAN_POINT ( 'NONE',  ( 21.49308418680749710, 7.713898994826276834, 2.801309206857172995 ) ) ;
#30976=CARTESIAN_POINT ( 'NONE',  ( 23.46066938646308841, 1.523794879705043792, -5.010722692604085537 ) ) ;
#30978=EDGE_CURVE ( 'NONE', #26946, #11923, #33542, .T. ) ;
#30984=CARTESIAN_POINT ( 'NONE',  ( 87.47409246771869107, -1.962666243356603557, 3.672687813029068771 ) ) ;
#30992=CARTESIAN_POINT ( 'NONE',  ( 24.07681195139318930, 3.355352448838379242, 3.179409747024673827 ) ) ;
#30994=CIRCLE ( 'NONE', #32949, 6.000000000000002665 ) ;
#30995=EDGE_CURVE ( 'NONE', #10306, #22791, #14929, .T. ) ;
#30998=CARTESIAN_POINT ( 'NONE',  ( 16.81957533019866702, 9.797912850251352168, -2.500000000000367706 ) ) ;
#31004=CARTESIAN_POINT ( 'NONE',  ( 22.39040353993711108, 2.683735211801196563, -8.168217153243197970 ) ) ;
#31006=CARTESIAN_POINT ( 'NONE',  ( -76.09017072707489149, 8.929435588302428783, 8.593849483394778943 ) ) ;
#31007=CARTESIAN_POINT ( 'NONE',  ( 36.96316948681300119, -3.289061831793972157, 5.933911304578510126 ) ) ;
#31008=CARTESIAN_POINT ( 'NONE',  ( 1.700390093233090871, -29.56993018339339940, 6.000000000000000000 ) ) ;
#31009=CARTESIAN_POINT ( 'NONE',  ( -80.96054980827190661, 10.55948373611085778, -0.1886338521618539932 ) ) ;
#31010=CARTESIAN_POINT ( 'NONE',  ( 30.68921806961705556, -2.925807085693435727, -4.996192719944245297 ) ) ;
#31011=CARTESIAN_POINT ( 'NONE',  ( 37.18663386580139729, -2.963620350049941177, -6.000007560707241616 ) ) ;
#31013=CARTESIAN_POINT ( 'NONE',  ( 14.79496864341336604, 12.68087409683664823, 2.510197516273051654 ) ) ;
#31018=CARTESIAN_POINT ( 'NONE',  ( 22.01630332033667514, 0.2560055906900143841, -7.605423277453922104 ) ) ;
#31020=CARTESIAN_POINT ( 'NONE',  ( 36.85527851974480029, -2.080028804847991353, -5.860598804419308472 ) ) ;
#31021=CARTESIAN_POINT ( 'NONE',  ( 24.66063408182436945, 2.989447463104236036, -3.506463971955919412 ) ) ;
#31025=CARTESIAN_POINT ( 'NONE',  ( 29.17643449372946307, 0.5759355299653177163, 4.760086256117967984 ) ) ;
#31029=CARTESIAN_POINT ( 'NONE',  ( 88.66616934308579800, -1.912773240965560673, 2.173515562489431563 ) ) ;
#31030=CARTESIAN_POINT ( 'NONE',  ( -71.92837670882107659, -20.78299143688747819, 5.916079783099617906 ) ) ;
#31031=CARTESIAN_POINT ( 'NONE',  ( 37.03859629130157316, -3.000568126192123319, -5.987166751730718772 ) ) ;
#31033=ORIENTED_EDGE ( 'NONE', *, *, #21440, .F. ) ;
#31034=CARTESIAN_POINT ( 'NONE',  ( 24.73897951283172247, 3.010565050160694422, 3.390208192849414548 ) ) ;
#31044=ORIENTED_EDGE ( 'NONE', *, *, #40046, .T. ) ;
#31050=CARTESIAN_POINT ( 'NONE',  ( 33.89871771371753084, -5.477042562592300712, 0.06951882857151732431 ) ) ;
#31051=EDGE_LOOP ( 'NONE', ( #31953, #22281, #19141, #22452 ) ) ;
#31053=VECTOR ( 'NONE', #25141, 1000.000000000000000 ) ;
#31054=CARTESIAN_POINT ( 'NONE',  ( -78.00837106247750796, -5.149560780178712882, -7.068249347921222281 ) ) ;
#31057=CARTESIAN_POINT ( 'NONE',  ( 86.17157777234386629, 0.6269314577163517255, 5.990399513018050293 ) ) ;
#31062=EDGE_CURVE ( 'NONE', #21833, #15683, #33336, .T. ) ;
#31065=CARTESIAN_POINT ( 'NONE',  ( 19.70092807311216987, -3.044756132290810768, -3.216959551844232656 ) ) ;
#31069=CARTESIAN_POINT ( 'NONE',  ( 33.68728320403869247, -3.101957757517421754, 5.464113292652290177 ) ) ;
#31076=CARTESIAN_POINT ( 'NONE',  ( 14.74006167184663241, -5.120305118510855458, 2.499999999999999556 ) ) ;
#31077=CARTESIAN_POINT ( 'NONE',  ( 16.62281228516970799, -3.166379901436700006, 2.800789899971793062 ) ) ;
#31078=CARTESIAN_POINT ( 'NONE',  ( -69.42837670882107659, -47.11702805680359063, 9.886859966642603581 ) ) ;
#31079=AXIS2_PLACEMENT_3D ( 'NONE', #25055, #18865, #28336 ) ;
#31088=CARTESIAN_POINT ( 'NONE',  ( 22.24090466686359946, 3.269623998474210591, 4.510814169736189427 ) ) ;
#31094=CARTESIAN_POINT ( 'NONE',  ( -70.79776717266595654, 0.2170085631123328807, 5.999999999999970690 ) ) ;
#31095=PLANE ( 'NONE',  #18353 ) ;
#31096=CARTESIAN_POINT ( 'NONE',  ( -80.92837670882107659, 2.429809908903242555, 12.50000000000000000 ) ) ;
#31100=CARTESIAN_POINT ( 'NONE',  ( 23.27552172775332551, 3.086263684135279295, -3.977210565842318246 ) ) ;
#31103=CARTESIAN_POINT ( 'NONE',  ( 21.85643539959774273, -7.673977846683588844, 14.52234238348545681 ) ) ;
#31107=CARTESIAN_POINT ( 'NONE',  ( 87.92727933775610438, -0.4063688358931643041, -3.816426586085390760 ) ) ;
#31111=CARTESIAN_POINT ( 'NONE',  ( 23.83988866691774078, -2.865115883751661929, 3.921967457249267319 ) ) ;
#31113=CARTESIAN_POINT ( 'NONE',  ( 36.89759893298676019, -3.003103866610235873, -5.965160703931689845 ) ) ;
#31116=EDGE_CURVE ( 'NONE', #10579, #39042, #18909, .T. ) ;
#31117=CARTESIAN_POINT ( 'NONE',  ( 21.89888535303197870, 5.088844031853470895, -3.617585142307979673 ) ) ;
#31119=CARTESIAN_POINT ( 'NONE',  ( -69.58118028693378676, -46.45007417365150815, 5.846929218950453588 ) ) ;
#31120=ADVANCED_FACE ( 'NONE', ( #18676 ), #19299, .T. ) ;
#31123=CARTESIAN_POINT ( 'NONE',  ( 35.83223476015841413, -3.727955879379408533, 5.624514018808150162 ) ) ;
#31127=CARTESIAN_POINT ( 'NONE',  ( 87.98680850476117143, -0.4732348216977415589, -3.104595713354958875 ) ) ;
#31128=CARTESIAN_POINT ( 'NONE',  ( -74.35246078617609555, 9.035812363374233769, -9.396779859613371144 ) ) ;
#31130=DIRECTION ( 'NONE',  ( 0.000000000000000000, -1.000000000000000000, 0.000000000000000000 ) ) ;
#31131=VECTOR ( 'NONE', #3758, 1000.000000000000000 ) ;
#31134=CARTESIAN_POINT ( 'NONE',  ( 23.73628397669238055, 3.550931190053107311, 3.214768951104281847 ) ) ;
#31143=CARTESIAN_POINT ( 'NONE',  ( 14.96406161801628443, 11.85168694806318257, -2.541901741326018982 ) ) ;
#31150=CIRCLE ( 'NONE', #10751, 10.00000000000000888 ) ;
#31155=CARTESIAN_POINT ( 'NONE',  ( 32.01248540970218670, -4.887874588265229470, -2.123135123820048875 ) ) ;
#31156=DIRECTION ( 'NONE',  ( 0.000000000000000000, 1.000000000000000000, 0.000000000000000000 ) ) ;
#31159=CARTESIAN_POINT ( 'NONE',  ( 21.79325021498261705, 0.2292132057495366859, -8.345714203105845996 ) ) ;
#31166=CARTESIAN_POINT ( 'NONE',  ( 37.15677058856715576, -2.581106085008523898, -5.983794649111914943 ) ) ;
#31168=CARTESIAN_POINT ( 'NONE',  ( 28.67087680535204797, -4.024283280459782119, 4.110896467804376009 ) ) ;
#31187=CARTESIAN_POINT ( 'NONE',  ( 21.82973510601959788, 5.967885360353585078, 3.133254696524513605 ) ) ;
#31198=B_SPLINE_SURFACE_WITH_KNOTS ( 'NONE', 5, 3, ( 
 ( #15756, #6087, #22153, #31010, #34725, #34317, #12867 ),
 ( #6504, #5886, #19053, #28310, #2815, #128, #31616 ),
 ( #27894, #18422, #31210, #8950, #2615, #25235, #15134 ),
 ( #3439, #15955, #27690, #12249, #37366, #40246, #12032 ),
 ( #24610, #9162, #3031, #19458, #3839, #28725, #16356 ),
 ( #9780, #34927, #6902, #22362, #25635, #28930, #6705 ),
 ( #32032, #19253, #731, #31822, #3636, #38177, #16161 ),
 ( #537, #13073, #9980, #22559, #35124, #37460, #27997 ) ),
 .UNSPECIFIED., .F., .F., .F.,
 ( 6, 2, 6 ),
 ( 4, 1, 1, 1, 4 ),
 ( 0.000000000000000000, 0.5000000000000000000, 1.000000000000000000 ),
 ( 0.000000000000000000, 0.001659480086290941693, 0.002765800143818236082, 0.004008671076256031980, 0.005388092883604330037 ),
 .UNSPECIFIED. ) ;
#31200=CARTESIAN_POINT ( 'NONE',  ( -70.92837670882106238, -48.61702805680358352, 6.000000000000002665 ) ) ;
#31201=CARTESIAN_POINT ( 'NONE',  ( 22.37440129197860728, 3.331413251109061058, -7.657642981191555620 ) ) ;
#31204=CARTESIAN_POINT ( 'NONE',  ( -75.82730537676935967, 10.26191331253318673, 8.725661018608912300 ) ) ;
#31205=CARTESIAN_POINT ( 'NONE',  ( 14.61802081865033642, -4.660388157181345470, -2.500000000000000000 ) ) ;
#31207=CARTESIAN_POINT ( 'NONE',  ( -69.42837670882107659, -47.11702805680359063, 5.809475019311128641 ) ) ;
#31210=CARTESIAN_POINT ( 'NONE',  ( 32.00046961360993691, -3.138592191753610372, -5.200845236069852717 ) ) ;
#31211=CARTESIAN_POINT ( 'NONE',  ( 35.73199623123087321, -1.301391055416668552, -5.535525800874729008 ) ) ;
#31213=CARTESIAN_POINT ( 'NONE',  ( 14.73041858808750426, 13.02581678099233287, 2.501001369465592372 ) ) ;
#31218=CARTESIAN_POINT ( 'NONE',  ( 18.48595909569426610, 13.25013647629958768, -2.499999999999999112 ) ) ;
#31219=CARTESIAN_POINT ( 'NONE',  ( 21.73669896701832016, 0.3099803614507385396, -8.866688668638362358 ) ) ;
#31221=CARTESIAN_POINT ( 'NONE',  ( 25.67289584648164080, 2.139690751649415024, -4.140607619995577693 ) ) ;
#31225=CARTESIAN_POINT ( 'NONE',  ( 27.44841020286834166, 1.080609055311573252, 4.490386273103699644 ) ) ;
#31228=CARTESIAN_POINT ( 'NONE',  ( 85.61248512101352048, 1.464218027013357570, -5.526712519226341769 ) ) ;
#31229=CARTESIAN_POINT ( 'NONE',  ( 35.95133392841589171, -2.121479879121625167, -5.817473164462794166 ) ) ;
#31231=CARTESIAN_POINT ( 'NONE',  ( 24.42333371043659440, 2.822406383138230002, 3.828119244412326427 ) ) ;
#31233=LINE ( 'NONE', #34139, #40357 ) ;
#31239=AXIS2_PLACEMENT_3D ( 'NONE', #35176, #16010, #28780 ) ;
#31241=EDGE_LOOP ( 'NONE', ( #21225, #195, #23967, #11710 ) ) ;
#31256=CARTESIAN_POINT ( 'NONE',  ( 22.01991341521145173, 5.470200110361999712, -3.165064741469916232 ) ) ;
#31260=CARTESIAN_POINT ( 'NONE',  ( 25.48218379196744721, -4.266488024150952185, 3.117641769822204090 ) ) ;
#31261=CARTESIAN_POINT ( 'NONE',  ( -80.83477924395624825, -5.699948517445438512, -1.424373511022223537 ) ) ;
#31264=CARTESIAN_POINT ( 'NONE',  ( 84.21289197705223728, 3.045783863710543660, -0.4930364517660317802 ) ) ;
#31268=CARTESIAN_POINT ( 'NONE',  ( 17.49771952580762502, -6.259504178003650665, -2.500000000000000444 ) ) ;
#31272=CARTESIAN_POINT ( 'NONE',  ( 85.64493543437410494, 0.8953488218558967038, 5.847730123973997607 ) ) ;
#31274=CARTESIAN_POINT ( 'NONE',  ( 34.92925997322895881, -1.710623459408137759, 5.657953804803885767 ) ) ;
#31291=CARTESIAN_POINT ( 'NONE',  ( 24.63348758885817702, 2.687559539024136246, 3.900614856717827816 ) ) ;
#31300=LINE ( 'NONE', #3122, #24263 ) ;
#31304=CARTESIAN_POINT ( 'NONE',  ( 22.62432447131647706, 3.405416539215757599, -4.114152520097174914 ) ) ;
#31307=CARTESIAN_POINT ( 'NONE',  ( 21.85643539959776760, -14.20048109512665135, 6.697783101734796851 ) ) ;
#31308=CARTESIAN_POINT ( 'NONE',  ( 17.09215160921039356, 14.51084972821218599, 1.912535534561743411 ) ) ;
#31312=CARTESIAN_POINT ( 'NONE',  ( 86.21492201224262431, 1.517032185505227559, -5.007191195300914721 ) ) ;
#31314=CARTESIAN_POINT ( 'NONE',  ( 14.61802081865033642, 12.33286846116140190, 2.500000000000000000 ) ) ;
#31316=CARTESIAN_POINT ( 'NONE',  ( 33.94523891240480395, -3.271630530324667774, 5.504373519622959954 ) ) ;
#31318=CARTESIAN_POINT ( 'NONE',  ( 33.62927951164961371, -1.227240062974174650, -5.455060413628188165 ) ) ;
#31325=CARTESIAN_POINT ( 'NONE',  ( 27.81551784075586298, 1.843619295897225285, 3.908845422569096950 ) ) ;
#31328=ORIENTED_EDGE ( 'NONE', *, *, #4112, .T. ) ;
#31332=CARTESIAN_POINT ( 'NONE',  ( -74.64083662667529495, 9.321351725019315637, -9.286628282490790198 ) ) ;
#31336=DIRECTION ( 'NONE',  ( -1.000000000000000000, -1.165409145176969993E-16, 0.000000000000000000 ) ) ;
#31338=CARTESIAN_POINT ( 'NONE',  ( 22.19901381586180023, 5.214777149643200715, 3.111044880889567210 ) ) ;
#31342=ORIENTED_EDGE ( 'NONE', *, *, #13349, .F. ) ;
#31344=CARTESIAN_POINT ( 'NONE',  ( -71.68163889809667921, -45.81621559017686707, 5.953091488286674782 ) ) ;
#31346=CARTESIAN_POINT ( 'NONE',  ( 14.92465469600171524, 12.09808818448366807, -2.535751338085821427 ) ) ;
#31358=CARTESIAN_POINT ( 'NONE',  ( 29.60215801812428182, 1.109421360397880862, -4.380391640306282142 ) ) ;
#31360=DIRECTION ( 'NONE',  ( 1.000000000000000000, 0.000000000000000000, 0.000000000000000000 ) ) ;
#31368=CARTESIAN_POINT ( 'NONE',  ( 32.00275383920578065, 0.1412686694384412134, -4.903342167364729498 ) ) ;
#31372=LINE ( 'NONE', #5640, #27925 ) ;
#31373=CARTESIAN_POINT ( 'NONE',  ( 87.20660408302002509, 0.2574974038930863407, -5.635807106906071340 ) ) ;
#31374=CARTESIAN_POINT ( 'NONE',  ( 21.87459114891373702, -13.50524245770412257, 2.500000000000000444 ) ) ;
#31389=CARTESIAN_POINT ( 'NONE',  ( 24.06887988145387069, 3.350337168359989626, 3.200280518033681521 ) ) ;
#31394=CARTESIAN_POINT ( 'NONE',  ( 24.12588890033682887, 0.5212924738780745360, 5.092295861883279429 ) ) ;
#31398=ORIENTED_EDGE ( 'NONE', *, *, #38798, .F. ) ;
#31404=CARTESIAN_POINT ( 'NONE',  ( 21.85643539959776049, -11.26069278398387929, -1.499473835228683383 ) ) ;
#31407=CARTESIAN_POINT ( 'NONE',  ( -73.10008652833232645, 0.2745614453624863338, 10.93886590303131534 ) ) ;
#31411=DIRECTION ( 'NONE',  ( 1.000000000000000000, -8.959828616340678715E-16, 0.000000000000000000 ) ) ;
#31412=CARTESIAN_POINT ( 'NONE',  ( 33.68500911095676997, -3.840374874697897845, -5.137585959034770333 ) ) ;
#31415=CARTESIAN_POINT ( 'NONE',  ( 20.61347566090116246, 6.036182562928900985, 3.423629434313151698 ) ) ;
#31418=EDGE_CURVE ( 'NONE', #39042, #21520, #28850, .T. ) ;
#31419=FACE_OUTER_BOUND ( 'NONE', #4736, .T. ) ;
#31423=CARTESIAN_POINT ( 'NONE',  ( 25.52861145932945064, 1.274360088752857889, -4.422354827559902724 ) ) ;
#31424=CARTESIAN_POINT ( 'NONE',  ( 30.92600629254716793, -3.767230967968932198, -4.587853941829935778 ) ) ;
#31425=CARTESIAN_POINT ( 'NONE',  ( 26.61111181199286335, 1.629400868845519490, -4.332867922176739661 ) ) ;
#31429=CARTESIAN_POINT ( 'NONE',  ( 37.11163797912877271, -2.778243138683350821, 5.998008405196137538 ) ) ;
#31433=CARTESIAN_POINT ( 'NONE',  ( 84.36655727669636917, 3.025886916471207222, -1.294691096651311435 ) ) ;
#31434=CARTESIAN_POINT ( 'NONE',  ( 36.00510628997864870, -3.152656186843009412, -5.825865641974139031 ) ) ;
#31436=CARTESIAN_POINT ( 'NONE',  ( 24.71170268252853930, 2.643186313627579054, 3.922093749847886723 ) ) ;
#31438=CARTESIAN_POINT ( 'NONE',  ( 37.19747295490952155, -2.841588721108153415, -5.999818660317219887 ) ) ;
#31439=ORIENTED_EDGE ( 'NONE', *, *, #28208, .F. ) ;
#31443=ORIENTED_EDGE ( 'NONE', *, *, #215, .F. ) ;
#31447=CARTESIAN_POINT ( 'NONE',  ( 14.62858089720432631, 12.62725169013283377, 2.500000000000000000 ) ) ;
#31452=CARTESIAN_POINT ( 'NONE',  ( 27.27118286198125574, -4.471745766876631833, 3.644977776233934819 ) ) ;
#31455=CARTESIAN_POINT ( 'NONE',  ( 24.38063191036968647, 3.152000527247066142, -3.325049431601771133 ) ) ;
#31461=CARTESIAN_POINT ( 'NONE',  ( -81.48936617853665609, -5.631775123504498382, -2.862016309434455952 ) ) ;
#31464=CARTESIAN_POINT ( 'NONE',  ( 87.78960583812504126, -2.347739977990699778, 2.116702103816012759 ) ) ;
#31465=CARTESIAN_POINT ( 'NONE',  ( 24.97740817842744221, 3.110183573126763079, -2.920139942405988620 ) ) ;
#31475=ORIENTED_EDGE ( 'NONE', *, *, #1157, .T. ) ;
#31476=CARTESIAN_POINT ( 'NONE',  ( 33.62750157612018143, -1.232156386184390495, 5.454782923789285753 ) ) ;
#31478=CARTESIAN_POINT ( 'NONE',  ( 85.63852691662546590, 2.164466514264067332, 3.769402685279828358 ) ) ;
#31483=DIRECTION ( 'NONE',  ( 0.000000000000000000, -0.000000000000000000, -1.000000000000000000 ) ) ;
#31486=CARTESIAN_POINT ( 'NONE',  ( 24.89525126181291981, -5.810506762332490638, -2.873249729385407125 ) ) ;
#31488=CARTESIAN_POINT ( 'NONE',  ( -79.12200251776535254, -6.600066278497241257, 5.748117179618010830 ) ) ;
#31492=CARTESIAN_POINT ( 'NONE',  ( 23.63060222782971920, 2.673617165426260822, 4.137625349533057495 ) ) ;
#31493=CARTESIAN_POINT ( 'NONE',  ( 24.75830837035764276, 3.019210359990082804, 3.350572556515618583 ) ) ;
#31497=CARTESIAN_POINT ( 'NONE',  ( -7.890026461918812295, -6.626103207857777159E-16, -6.000000000000000000 ) ) ;
#31504=CARTESIAN_POINT ( 'NONE',  ( 22.02891390162299246, 3.924681071272548838, -4.221871318386710925 ) ) ;
#31505=EDGE_LOOP ( 'NONE', ( #28810, #9775, #25600, #36892 ) ) ;
#31508=CARTESIAN_POINT ( 'NONE',  ( 21.85643539959779602, 5.813509198596546135, -11.62788251339591206 ) ) ;
#31512=CARTESIAN_POINT ( 'NONE',  ( 84.99141033049929206, 2.891338577806874088, -0.4625859348280507155 ) ) ;
#31516=CARTESIAN_POINT ( 'NONE',  ( 19.70069104262061543, -2.834677804756353225, 3.278428930171599198 ) ) ;
#31517=CARTESIAN_POINT ( 'NONE',  ( 34.77301379943533988, -3.161486423658268929, -5.633567810555343058 ) ) ;
#31524=CARTESIAN_POINT ( 'NONE',  ( 32.01160833602948941, -2.960095084777874863, 5.202583703147388050 ) ) ;
#31527=CARTESIAN_POINT ( 'NONE',  ( 37.18616516907447078, -2.963186209105021618, 6.000013960849525319 ) ) ;
#31530=CARTESIAN_POINT ( 'NONE',  ( 87.54002591101105679, -2.043453341785346655, -3.425432998280521613 ) ) ;
#31534=CARTESIAN_POINT ( 'NONE',  ( 88.13815211262131299, -0.6432311452471944913, -2.427475510744327547 ) ) ;
#31538=DIRECTION ( 'NONE',  ( -0.000000000000000000, -0.000000000000000000, -1.000000000000000000 ) ) ;
#31543=CARTESIAN_POINT ( 'NONE',  ( 21.73868531115960678, 6.081862488199073269, 3.283576032310306481 ) ) ;
#31551=CARTESIAN_POINT ( 'NONE',  ( 20.06531201372480311, 6.854292503151608429, -3.230284889801701365 ) ) ;
#31559=CARTESIAN_POINT ( 'NONE',  ( 0.000000000000000000, 0.000000000000000000, -2.500000000000000000 ) ) ;
#31560=CARTESIAN_POINT ( 'NONE',  ( 15.21972599668117709, 10.50943688033427392, 2.499999999998679723 ) ) ;
#31561=CARTESIAN_POINT ( 'NONE',  ( 29.58677136987063960, -0.8116067495284342570, -6.002319972564883699 ) ) ;
#31563=CARTESIAN_POINT ( 'NONE',  ( 14.37591153880835293, -5.022958543253408514, 2.500000000000000444 ) ) ;
#31569=CARTESIAN_POINT ( 'NONE',  ( 33.45255242130070172, -3.771379754131906736, -5.158309509446562302 ) ) ;
#31570=CARTESIAN_POINT ( 'NONE',  ( 20.88448294811174932, 4.552397361489173733, -2.802001057294738917 ) ) ;
#31573=CARTESIAN_POINT ( 'NONE',  ( 19.67572283850595838, -2.760578293782835146, -3.277270426740663378 ) ) ;
#31580=VERTEX_POINT ( 'NONE', #19502 ) ;
#31584=ADVANCED_FACE ( 'NONE', ( #2861 ), #25476, .T. ) ;
#31586=CARTESIAN_POINT ( 'NONE',  ( 22.01541346579904967, 4.834729283906541220, -3.642368534677343117 ) ) ;
#31588=CARTESIAN_POINT ( 'NONE',  ( 21.85643539959776760, -15.29860455024666877, -0.2154785770160333180 ) ) ;
#31589=CARTESIAN_POINT ( 'NONE',  ( 22.38542502781336196, 4.029546766862340590, 3.839276850840922517 ) ) ;
#31593=CARTESIAN_POINT ( 'NONE',  ( 21.71224184863732631, 6.326580208086403978, 3.193838826403248454 ) ) ;
#31600=CARTESIAN_POINT ( 'NONE',  ( 27.16088236247300713, 1.273373388036902920, 4.440073707454521568 ) ) ;
#31608=CARTESIAN_POINT ( 'NONE',  ( 21.85643539959774273, 9.212406492340052822, 1.715677401501900956 ) ) ;
#31609=CARTESIAN_POINT ( 'NONE',  ( 21.85643539959776760, -15.22304117831051862, 1.450816989262757151 ) ) ;
#31610=EDGE_LOOP ( 'NONE', ( #35889, #28126, #13289, #25560, #3270, #28295, #33519 ) ) ;
#31611=CARTESIAN_POINT ( 'NONE',  ( -75.62813303713400614, 8.531731237985169969, 10.23129255942193261 ) ) ;
#31612=DIRECTION ( 'NONE',  ( -1.000000000000000000, 0.000000000000000000, 0.000000000000000000 ) ) ;
#31613=ORIENTED_EDGE ( 'NONE', *, *, #12414, .T. ) ;
#31616=CARTESIAN_POINT ( 'NONE',  ( 28.20719035837850441, -3.294622348659617117, -4.608812267538287877 ) ) ;
#31617=CARTESIAN_POINT ( 'NONE',  ( 34.63778478821021167, -0.7807839475658682193, -5.273897451186136287 ) ) ;
#31619=CARTESIAN_POINT ( 'NONE',  ( 21.58804800731853391, 5.739108358429902523, 3.444525775481035001 ) ) ;
#31621=CARTESIAN_POINT ( 'NONE',  ( 30.67406393699503298, -3.593393542108534344, -4.777508688867102116 ) ) ;
#31624=CARTESIAN_POINT ( 'NONE',  ( 26.56410588169512721, 1.659669406648513368, -4.323734781818131978 ) ) ;
#31625=CARTESIAN_POINT ( 'NONE',  ( 37.19747295490952155, -2.841588721108153415, -5.999818660317219887 ) ) ;
#31628=( BOUNDED_SURFACE ( )  B_SPLINE_SURFACE ( 3, 2, ( 
 ( #16013, #18901, #16211 ),
 ( #38428, #38230, #31878 ),
 ( #3893, #37821, #22213 ),
 ( #16408, #34782, #25687 ),
 ( #21793, #6558, #28578 ),
 ( #13316, #12511, #25290 ),
 ( #3687, #19103, #385 ),
 ( #15813, #22610, #28367 ) ),
 .UNSPECIFIED., .F., .F., .F. ) 
 B_SPLINE_SURFACE_WITH_KNOTS ( ( 4, 2, 2, 4 ),
 ( 3, 3 ),
 ( 0.002497028706408050639, 0.005364503022961082321, 0.006798240181237598379, 0.008231977339514114436 ),
 ( 0.000000000000000000, 1.000000000000000000 ),
 .UNSPECIFIED. ) 
 GEOMETRIC_REPRESENTATION_ITEM ( )  RATIONAL_B_SPLINE_SURFACE ( (
 ( 1.000000000000000000, 0.8503863343361129923, 1.000000000000000000),
 ( 1.000000000000000000, 0.8564594667157611196, 1.000000000000000000),
 ( 1.000000000000000000, 0.8588771854361650915, 1.000000000000000000),
 ( 1.000000000000000000, 0.8588307351573004622, 1.000000000000000000),
 ( 1.000000000000000000, 0.8581754178396920896, 1.000000000000000000),
 ( 1.000000000000000000, 0.8554071838990657817, 1.000000000000000000),
 ( 1.000000000000000000, 0.8533070252407790601, 1.000000000000000000),
 ( 1.000000000000000000, 0.8501577991238667975, 1.000000000000000000) ) ) 
 REPRESENTATION_ITEM ( '' )  SURFACE ( )  );
#31630=CARTESIAN_POINT ( 'NONE',  ( 35.91723242733118582, -1.971476223945344719, 5.812150800470588408 ) ) ;
#31633=CARTESIAN_POINT ( 'NONE',  ( 88.70663687723717317, -1.959581838532896025, -1.901098908833099621 ) ) ;
#31636=CARTESIAN_POINT ( 'NONE',  ( 37.00354821055626076, -2.736456545284593478, -5.981696651089377426 ) ) ;
#31639=CARTESIAN_POINT ( 'NONE',  ( 24.38334378067764163, 2.944219297565202176, 3.714561838593425147 ) ) ;
#31649=CARTESIAN_POINT ( 'NONE',  ( 1.700390093233090871, -29.56993018339339940, 6.000000000000001776 ) ) ;
#31653=ORIENTED_EDGE ( 'NONE', *, *, #18735, .T. ) ;
#31656=CARTESIAN_POINT ( 'NONE',  ( 28.67087680535204797, -4.024283280459782119, 4.110896467804376009 ) ) ;
#31659=CARTESIAN_POINT ( 'NONE',  ( 24.37313411410375963, 3.148815130053465250, -3.340199359379649291 ) ) ;
#31664=CARTESIAN_POINT ( 'NONE',  ( -80.91031161377242142, -5.699894439238891941, -0.6008404087775605085 ) ) ;
#31665=CARTESIAN_POINT ( 'NONE',  ( -17.69482985384421880, -29.56993018339339940, 6.000000000000000000 ) ) ;
#31668=CARTESIAN_POINT ( 'NONE',  ( 85.71231987865445490, 0.7872592507033150389, 5.912482239253596283 ) ) ;
#31669=CARTESIAN_POINT ( 'NONE',  ( 22.37949047700085359, 4.044367784810037669, -2.563457211823029880 ) ) ;
#31678=CARTESIAN_POINT ( 'NONE',  ( 31.71832800154010457, -0.5603227101564068890, 5.156810213938597620 ) ) ;
#31679=CARTESIAN_POINT ( 'NONE',  ( 86.82658554816774199, 0.8299826706514633612, -5.353109082705294952 ) ) ;
#31684=CARTESIAN_POINT ( 'NONE',  ( -69.72909178707443800, -48.03897060390835350, 9.928799107400003265 ) ) ;
#31685=CARTESIAN_POINT ( 'NONE',  ( -69.50501670448861091, -46.63360808430513060, 9.898256799676488527 ) ) ;
#31690=CARTESIAN_POINT ( 'NONE',  ( -80.66421687884188430, -6.623080169578322796, 2.321096592483072651 ) ) ;
#31695=CARTESIAN_POINT ( 'NONE',  ( 23.25599683166147713, 2.300726602830819978, 4.579218281655972334 ) ) ;
#31696=CARTESIAN_POINT ( 'NONE',  ( 33.45749450797183044, -3.829747548865578555, 5.093667367007288505 ) ) ;
#31698=ORIENTED_EDGE ( 'NONE', *, *, #4447, .T. ) ;
#31701=CARTESIAN_POINT ( 'NONE',  ( -69.92837670882107659, -0.7829914368874778541, 5.916079783099612577 ) ) ;
#31703=DIRECTION ( 'NONE',  ( 0.000000000000000000, 0.000000000000000000, 1.000000000000000000 ) ) ;
#31707=CARTESIAN_POINT ( 'NONE',  ( 23.87821936093323316, 3.129464447930911941, -3.683058660101061754 ) ) ;
#31709=CARTESIAN_POINT ( 'NONE',  ( 21.85643539959774273, 8.980655621775115449, -3.220279653634019468 ) ) ;
#31714=CARTESIAN_POINT ( 'NONE',  ( 87.25532471891827413, 0.3484024848758522364, -5.186905954794287510 ) ) ;
#31719=CARTESIAN_POINT ( 'NONE',  ( 14.77519537498673685, -4.508227731834313801, 2.512005464107180952 ) ) ;
#31721=CARTESIAN_POINT ( 'NONE',  ( 36.91112720548292714, -2.639121728185907845, -5.967272118037208806 ) ) ;
#31727=CARTESIAN_POINT ( 'NONE',  ( 30.69436886186574398, -3.339171598047946610, 4.972328070349530726 ) ) ;
#31730=AXIS2_PLACEMENT_3D ( 'NONE', #12426, #24995, #34690 ) ;
#31731=ORIENTED_EDGE ( 'NONE', *, *, #2071, .T. ) ;
#31732=CARTESIAN_POINT ( 'NONE',  ( 36.49318449278427323, -3.558291934896485653, 5.797216874782107787 ) ) ;
#31736=CARTESIAN_POINT ( 'NONE',  ( 88.34504873523731305, -0.8756272516756123947, 0.6794260907704854358 ) ) ;
#31743=CARTESIAN_POINT ( 'NONE',  ( 23.98072841137014777, 3.290854757922614393, 3.413282162417366816 ) ) ;
#31751=CARTESIAN_POINT ( 'NONE',  ( -71.84378200722045449, -45.92474028164770772, 5.930323375109142425 ) ) ;
#31753=CARTESIAN_POINT ( 'NONE',  ( 15.99242138985683681, 10.20549556836962779, -2.702402154696804004 ) ) ;
#31763=CARTESIAN_POINT ( 'NONE',  ( 28.08579234408868786, -0.7886013899455160958, -6.074239229908586779 ) ) ;
#31770=DIRECTION ( 'NONE',  ( 0.000000000000000000, 1.000000000000000000, 0.000000000000000000 ) ) ;
#31772=CARTESIAN_POINT ( 'NONE',  ( -70.92837670882107659, -45.61702805680359063, 6.000000000000002665 ) ) ;
#31773=CARTESIAN_POINT ( 'NONE',  ( 35.61928182240458796, -1.517342461334751036, -5.701831105538472499 ) ) ;
#31778=CARTESIAN_POINT ( 'NONE',  ( -81.79890681550139675, 10.46299657128043314, 0.6911394749367771873 ) ) ;
#31780=CARTESIAN_POINT ( 'NONE',  ( 21.99697979076537990, -11.79337463441197720, -2.500000000000000000 ) ) ;
#31781=CARTESIAN_POINT ( 'NONE',  ( 22.01888982478448042, -11.64019164401367945, 2.500000000000000000 ) ) ;
#31790=CARTESIAN_POINT ( 'NONE',  ( 23.96637146509650407, 2.887031144839279584, 3.870854377651337330 ) ) ;
#31791=B_SPLINE_CURVE_WITH_KNOTS ( 'NONE', 3,
 ( #7565, #32699, #4499, #19529 ),
 .UNSPECIFIED., .F., .F.,
 ( 4, 4 ),
 ( 0.05274299500989229617, 0.1795419177415450984 ),
 .UNSPECIFIED. ) ;
#31796=CARTESIAN_POINT ( 'NONE',  ( 19.46067669853512783, -3.065043108541300132, 3.182343406304090294 ) ) ;
#31803=CARTESIAN_POINT ( 'NONE',  ( 26.60903577415927757, 1.048885659047656960, 4.376956920250358429 ) ) ;
#31809=ADVANCED_FACE ( 'NONE', ( #23777 ), #38451, .F. ) ;
#31812=CARTESIAN_POINT ( 'NONE',  ( 22.81652408475101979, -6.765098194116612618, -2.522738730058198264 ) ) ;
#31815=CARTESIAN_POINT ( 'NONE',  ( -76.06923559113667466, 8.888346553459479438, 10.02136333681344027 ) ) ;
#31816=CARTESIAN_POINT ( 'NONE',  ( 24.11609145789137543, 0.4541001735588878763, -5.103011939257064533 ) ) ;
#31817=ORIENTED_EDGE ( 'NONE', *, *, #19712, .T. ) ;
#31822=CARTESIAN_POINT ( 'NONE',  ( 30.75021987934201206, -3.703070994598137045, -4.640474062878059414 ) ) ;
#31823=CARTESIAN_POINT ( 'NONE',  ( 29.48879446675499949, 1.220267147247336981, -4.220664948178088238 ) ) ;
#31825=CARTESIAN_POINT ( 'NONE',  ( 16.14458128353912869, 10.33471859280096083, 2.711087558826402510 ) ) ;
#31831=CARTESIAN_POINT ( 'NONE',  ( 30.82885584354832886, 0.7157400049436221101, -4.487457763936902211 ) ) ;
#31838=CARTESIAN_POINT ( 'NONE',  ( 87.06807637922989329, 0.009568187950425697044, -5.830412620327568796 ) ) ;
#31840=EDGE_LOOP ( 'NONE', ( #12907, #32324, #8895, #39913, #6171, #15473 ) ) ;
#31841=CARTESIAN_POINT ( 'NONE',  ( 24.58836688147599503, 2.713802262352938310, 3.887621106702806362 ) ) ;
#31857=CARTESIAN_POINT ( 'NONE',  ( 33.85503891423564227, -5.198044821503557067, -2.407580783687792714 ) ) ;
#31858=CARTESIAN_POINT ( 'NONE',  ( 22.00038671397952328, 5.557044130675768301, -3.122614658259094345 ) ) ;
#31869=CARTESIAN_POINT ( 'NONE',  ( -78.21354329911019931, -5.182362620687199772, -8.529621072396848191 ) ) ;
#31877=CARTESIAN_POINT ( 'NONE',  ( -70.92837670882107659, 13.37661300689599742, 0.000000000000000000 ) ) ;
#31878=CARTESIAN_POINT ( 'NONE',  ( 24.93859128955816118, 3.471607954000472507, 1.313953044955986638 ) ) ;
#31881=CARTESIAN_POINT ( 'NONE',  ( 14.61802081865033642, -65.19654454972992141, -3.500000000000000000 ) ) ;
#31886=CARTESIAN_POINT ( 'NONE',  ( 36.63360656337776788, -3.080934146991386235, 5.923958309974630687 ) ) ;
#31889=CARTESIAN_POINT ( 'NONE',  ( 86.52980085923458375, 1.163345319512251841, 5.105528906334227734 ) ) ;
#31892=CARTESIAN_POINT ( 'NONE',  ( 14.77114201464572751, -5.163092950663593861, 2.500000000000000000 ) ) ;
#31894=FACE_OUTER_BOUND ( 'NONE', #38091, .T. ) ;
#31898=VERTEX_POINT ( 'NONE', #17341 ) ;
#31902=CARTESIAN_POINT ( 'NONE',  ( 24.05450016081345055, 3.308680331767146043, 3.188065492737387707 ) ) ;
#31903=CARTESIAN_POINT ( 'NONE',  ( 25.20701090240159559, 1.570586567452724180, 4.374205870625836212 ) ) ;
#31909=CARTESIAN_POINT ( 'NONE',  ( 85.73540692764241555, 2.055646287687114881, 3.760641883467473967 ) ) ;
#31913=CARTESIAN_POINT ( 'NONE',  ( 22.40668529979953405, 3.759187042868666673, -4.020463199049926217 ) ) ;
#31917=CARTESIAN_POINT ( 'NONE',  ( 21.85643539959776760, -10.46150609831112455, 5.349806725441734301 ) ) ;
#31919=CARTESIAN_POINT ( 'NONE',  ( 17.09067283330163178, 14.51200607630100947, 6.135166493427014844E-13 ) ) ;
#31924=CARTESIAN_POINT ( 'NONE',  ( 88.76896161869186130, -1.545781173472005943, 2.128395682968124092 ) ) ;
#31927=ORIENTED_EDGE ( 'NONE', *, *, #26203, .F. ) ;
#31928=CARTESIAN_POINT ( 'NONE',  ( 15.54228167590041387, -3.627593571885062929, 2.632146965663780591 ) ) ;
#31929=CARTESIAN_POINT ( 'NONE',  ( 37.05019957443847289, -2.827376547557467923, 5.988977724690694338 ) ) ;
#31930=CARTESIAN_POINT ( 'NONE',  ( 31.09877180861311174, -3.763035568191606561, 4.622249389808555264 ) ) ;
#31931=CARTESIAN_POINT ( 'NONE',  ( 35.45376175006065722, -1.914248393079300614, -5.739814992201846877 ) ) ;
#31940=CARTESIAN_POINT ( 'NONE',  ( 36.88774144847645431, -3.350387819064732042, 5.910883484843293623 ) ) ;
#31947=CARTESIAN_POINT ( 'NONE',  ( -80.93488670107193172, 11.45404655845930897, -0.2160027379189757291 ) ) ;
#31948=DIRECTION ( 'NONE',  ( -0.000000000000000000, -1.000000000000000000, -0.000000000000000000 ) ) ;
#31953=ORIENTED_EDGE ( 'NONE', *, *, #20915, .F. ) ;
#31954=CARTESIAN_POINT ( 'NONE',  ( 22.45301647707092130, 4.683739370715508166, 3.229772300555033393 ) ) ;
#31961=ORIENTED_EDGE ( 'NONE', *, *, #36491, .F. ) ;
#31965=CARTESIAN_POINT ( 'NONE',  ( 14.82829946762850604, 12.56923040459623131, -2.515064524949301550 ) ) ;
#31968=ORIENTED_EDGE ( 'NONE', *, *, #17621, .F. ) ;
#31973=FACE_OUTER_BOUND ( 'NONE', #4206, .T. ) ;
#31975=CARTESIAN_POINT ( 'NONE',  ( 26.56634348862415251, 2.991955253353971500, -0.5426703667890996341 ) ) ;
#31984=CARTESIAN_POINT ( 'NONE',  ( 36.94055750684482575, -3.101496826522602834, -5.970271882717379519 ) ) ;
#31985=CARTESIAN_POINT ( 'NONE',  ( -61.24591834330252027, -23.80776546975053520, -2.500000000000000000 ) ) ;
#31988=CARTESIAN_POINT ( 'NONE',  ( -78.24496198277260817, 10.07981855400444893, 8.538017541507711528 ) ) ;
#31990=CARTESIAN_POINT ( 'NONE',  ( 21.85643539959775694, -14.32925462369614777, -2.499999999999999112 ) ) ;
#31991=EDGE_CURVE ( 'NONE', #37655, #22978, #19210, .T. ) ;
#31998=CARTESIAN_POINT ( 'NONE',  ( 30.24633204896981198, -2.992142132496548701, 4.927069645183380864 ) ) ;
#31999=CARTESIAN_POINT ( 'NONE',  ( 22.79610047791596728, 3.604602707705051756, 3.842052490992408753 ) ) ;
#32006=EDGE_CURVE ( 'NONE', #15320, #5482, #19807, .T. ) ;
#32007=CARTESIAN_POINT ( 'NONE',  ( 24.40382785946252397, 3.162689046678688332, 3.275147752357558062 ) ) ;
#32013=CARTESIAN_POINT ( 'NONE',  ( 24.73856604073376531, 0.6067268420280569341, 4.778954243596831297 ) ) ;
#32019=EDGE_CURVE ( 'NONE', #31580, #36975, #14270, .T. ) ;
#32023=CARTESIAN_POINT ( 'NONE',  ( 24.08269697565317813, 2.216436711090640888, -5.807619368686713024 ) ) ;
#32026=CARTESIAN_POINT ( 'NONE',  ( -73.03051304180658576, -2.422576877779497817, 9.778627833697271399 ) ) ;
#32028=EDGE_LOOP ( 'NONE', ( #37861, #36725, #31698, #26769, #10065, #7368, #2278 ) ) ;
#32029=DIRECTION ( 'NONE',  ( 0.000000000000000000, 0.000000000000000000, 1.000000000000000000 ) ) ;
#32032=CARTESIAN_POINT ( 'NONE',  ( 33.45255242130070172, -3.771379754131906736, -5.158309509446562302 ) ) ;
#32033=CARTESIAN_POINT ( 'NONE',  ( 23.38581192113748131, 3.559989847120099249, -3.092800859860194596 ) ) ;
#32035=CARTESIAN_POINT ( 'NONE',  ( 18.39192889356358052, 7.837295566124166335, 3.076903332958516479 ) ) ;
#32036=DIRECTION ( 'NONE',  ( 0.01395351027862084224, -0.9999026450364577601, 0.000000000000000000 ) ) ;
#32041=CARTESIAN_POINT ( 'NONE',  ( 21.77265313641114730, 1.017649519091238020, -7.447328431849799202 ) ) ;
#32042=CARTESIAN_POINT ( 'NONE',  ( 29.60103149450674209, 1.174864541282398811, -4.249889681204039427 ) ) ;
#32045=VECTOR ( 'NONE', #32107, 1000.000000000000000 ) ;
#32051=CARTESIAN_POINT ( 'NONE',  ( 84.76444386024292044, 2.549623173165235457, -3.635552437183829699 ) ) ;
#32052=EDGE_CURVE ( 'NONE', #36134, #6701, #18244, .T. ) ;
#32054=CARTESIAN_POINT ( 'NONE',  ( -75.56641529447675509, 8.489127916099096893, -10.26308220464040311 ) ) ;
#32061=FACE_OUTER_BOUND ( 'NONE', #28191, .T. ) ;
#32067=ORIENTED_EDGE ( 'NONE', *, *, #39734, .T. ) ;
#32072=CARTESIAN_POINT ( 'NONE',  ( 33.81879998282443722, -5.004485781189142557, -3.047669085721047111 ) ) ;
#32074=CARTESIAN_POINT ( 'NONE',  ( 23.43185404716432529, 3.785464407461396341, -3.124690735438692801 ) ) ;
#32081=CARTESIAN_POINT ( 'NONE',  ( -72.89874933986990868, 1.445529238484094980, -9.863921881214876564 ) ) ;
#32085=CARTESIAN_POINT ( 'NONE',  ( 86.59537683758360060, -0.3992097724244685342, -5.811584838773467432 ) ) ;
#32086=DIRECTION ( 'NONE',  ( 1.000000000000000000, 0.000000000000000000, 0.000000000000000000 ) ) ;
#32089=CYLINDRICAL_SURFACE ( 'NONE', #13031, 7.744449365083023729 ) ;
#32090=CARTESIAN_POINT ( 'NONE',  ( 33.60298752457206461, -1.218802016134334920, 5.450956913170565521 ) ) ;
#32093=ADVANCED_FACE ( 'NONE', ( #884 ), #23299, .T. ) ;
#32099=CARTESIAN_POINT ( 'NONE',  ( 36.64607077520608414, -2.461557252482897695, 5.925903651678381401 ) ) ;
#32102=CARTESIAN_POINT ( 'NONE',  ( 85.82060591106392167, 1.959946745720340777, 4.199140470389015611 ) ) ;
#32104=ORIENTED_EDGE ( 'NONE', *, *, #27458, .T. ) ;
#32107=DIRECTION ( 'NONE',  ( 0.000000000000000000, 1.000000000000000000, 0.000000000000000000 ) ) ;
#32111=EDGE_CURVE ( 'NONE', #23738, #29737, #7422, .T. ) ;
#32113=CARTESIAN_POINT ( 'NONE',  ( -76.18567808263772179, -5.622137304219937626, 8.514488760352879382 ) ) ;
#32115=ORIENTED_EDGE ( 'NONE', *, *, #33850, .F. ) ;
#32118=CARTESIAN_POINT ( 'NONE',  ( 23.32705478529917187, 2.029264981615857444, 4.738981897168647706 ) ) ;
#32120=VERTEX_POINT ( 'NONE', #7847 ) ;
#32124=CARTESIAN_POINT ( 'NONE',  ( 14.74978830686065301, 12.47633826711700600, -2.508459208900547743 ) ) ;
#32125=CARTESIAN_POINT ( 'NONE',  ( 86.44490267695917396, 1.258706987354809348, 4.883621451348188813 ) ) ;
#32131=CARTESIAN_POINT ( 'NONE',  ( 22.21620953772258744, 3.796930799149246472, -4.142915743477519896 ) ) ;
#32134=CARTESIAN_POINT ( 'NONE',  ( 21.85643539959778181, 1.552649203755968488, -12.31912549844641447 ) ) ;
#32135=CARTESIAN_POINT ( 'NONE',  ( 21.76122352785010605, 6.560793838968803193, 3.350653129119654405 ) ) ;
#32138=CARTESIAN_POINT ( 'NONE',  ( 87.43361094620441065, 0.1481429324132612357, -5.028924837761966415 ) ) ;
#32143=CARTESIAN_POINT ( 'NONE',  ( 14.60763624620907919, -5.047772731472147889, 2.486272941875335984 ) ) ;
#32144=CARTESIAN_POINT ( 'NONE',  ( 33.05017804490641709, -3.814651194816198743, 5.008230371610723708 ) ) ;
#32145=CARTESIAN_POINT ( 'NONE',  ( 21.25451605427406676, 3.323545792246858976, -3.523679291319553375 ) ) ;
#32146=LINE ( 'NONE', #6807, #4946 ) ;
#32151=CARTESIAN_POINT ( 'NONE',  ( 28.39362077150625296, -3.972643944815215988, 4.268989596475896597 ) ) ;
#32152=VECTOR ( 'NONE', #9315, 1000.000000000000000 ) ;
#32155=CARTESIAN_POINT ( 'NONE',  ( 34.63654108703977386, -0.7829625105204697233, 5.276317761283050523 ) ) ;
#32158=CARTESIAN_POINT ( 'NONE',  ( 87.33285498545190251, -1.784623943069521435, 4.108613016059194045 ) ) ;
#32182=CARTESIAN_POINT ( 'NONE',  ( 28.36395155556995817, 1.046816072451675517, -4.961098188302698553 ) ) ;
#32188=DIRECTION ( 'NONE',  ( 0.000000000000000000, 0.000000000000000000, 1.000000000000000000 ) ) ;
#32189=CARTESIAN_POINT ( 'NONE',  ( 37.02986127830654084, -2.495646223213518144, -5.974012795379922025 ) ) ;
#32194=CARTESIAN_POINT ( 'NONE',  ( -8.295002936191391285, 28.24537450226321411, 2.500000000000000000 ) ) ;
#32206=EDGE_CURVE ( 'NONE', #34818, #37831, #23521, .T. ) ;
#32207=CARTESIAN_POINT ( 'NONE',  ( 24.13130278612604940, 2.937171867363354227, 3.784435561684969418 ) ) ;
#32212=DIRECTION ( 'NONE',  ( -0.9999026450364576490, -0.01395351027862084224, 0.000000000000000000 ) ) ;
#32216=CARTESIAN_POINT ( 'NONE',  ( 21.99573204474387467, 0.2403451770729164994, 7.663175214092573739 ) ) ;
#32225=CARTESIAN_POINT ( 'NONE',  ( 24.99136039731803294, -2.601164552868876267, 6.036718378868273227 ) ) ;
#32226=EDGE_CURVE ( 'NONE', #33153, #24052, #16746, .T. ) ;
#32228=ORIENTED_EDGE ( 'NONE', *, *, #37782, .F. ) ;
#32229=CARTESIAN_POINT ( 'NONE',  ( -74.30460642558605855, -2.214477923546239957, 10.70245808945297661 ) ) ;
#32230=CARTESIAN_POINT ( 'NONE',  ( -62.92837670882106238, -52.49535338866468948, -6.000000000000000000 ) ) ;
#32236=CARTESIAN_POINT ( 'NONE',  ( 36.20073155144311272, -3.649434425297155116, -5.718600478983131730 ) ) ;
#32239=CARTESIAN_POINT ( 'NONE',  ( 17.35308537373412108, 8.839742678962347000, 2.914766677163659558 ) ) ;
#32240=DIRECTION ( 'NONE',  ( 0.9999026450364576490, 0.01395351027862084051, 0.000000000000000000 ) ) ;
#32241=CARTESIAN_POINT ( 'NONE',  ( -4.890026461918809630, -25.50263309590217276, 27.90461065042423527 ) ) ;
#32246=ADVANCED_FACE ( 'NONE', ( #15604 ), #32089, .T. ) ;
#32248=CARTESIAN_POINT ( 'NONE',  ( 23.87443714975944431, 1.367339853345398426, -4.872535488811999826 ) ) ;
#32249=CARTESIAN_POINT ( 'NONE',  ( 35.49974038668526077, -1.192779227918109086, -5.483795844434342648 ) ) ;
#32250=DIRECTION ( 'NONE',  ( 1.385724075720358314E-16, -1.000000000000000000, 0.000000000000000000 ) ) ;
#32252=CARTESIAN_POINT ( 'NONE',  ( 86.28404140065768502, 0.1054103399587360407, 6.008803426180587159 ) ) ;
#32253=ADVANCED_FACE ( 'NONE', ( #6756 ), #31628, .F. ) ;
#32255=CARTESIAN_POINT ( 'NONE',  ( -81.82457292829037954, 10.46020204711655843, -0.1745755204938225225 ) ) ;
#32258=DIRECTION ( 'NONE',  ( -0.000000000000000000, -1.000000000000000000, -0.000000000000000000 ) ) ;
#32259=VERTEX_POINT ( 'NONE', #10027 ) ;
#32266=DIRECTION ( 'NONE',  ( -0.000000000000000000, -0.000000000000000000, -1.000000000000000000 ) ) ;
#32269=CARTESIAN_POINT ( 'NONE',  ( 27.40513141245228468, 1.065180075448391772, 4.483631571157760121 ) ) ;
#32270=CARTESIAN_POINT ( 'NONE',  ( 27.37917897173983661, -4.430804881127424544, 3.681097677848294669 ) ) ;
#32272=CARTESIAN_POINT ( 'NONE',  ( 21.85643539959773207, -2.612013071670181041, -15.99649826491319971 ) ) ;
#32273=CARTESIAN_POINT ( 'NONE',  ( 24.04917647243221879, 3.336295066126922393, -3.255249733571578652 ) ) ;
#32274=ORIENTED_EDGE ( 'NONE', *, *, #17278, .T. ) ;
#32277=CARTESIAN_POINT ( 'NONE',  ( -4.266520354791871306, -48.67644278316300444, -2.500000000000000444 ) ) ;
#32279=CARTESIAN_POINT ( 'NONE',  ( -76.09606208423944906, -4.068416357244072579, -8.586815735137202310 ) ) ;
#32280=FACE_OUTER_BOUND ( 'NONE', #37130, .T. ) ;
#32283=CARTESIAN_POINT ( 'NONE',  ( 85.92174427069515730, 0.4035765525155806666, 6.008818417626160979 ) ) ;
#32284=DIRECTION ( 'NONE',  ( 0.000000000000000000, 0.000000000000000000, 1.000000000000000000 ) ) ;
#32288=( BOUNDED_CURVE ( )  B_SPLINE_CURVE ( 3, ( #24894, #22223, #28590, #12937 ),
 .UNSPECIFIED., .F., .T. ) 
 B_SPLINE_CURVE_WITH_KNOTS ( ( 4, 4 ),
 ( 3.394272908731871485, 3.785093762383077820 ),
 .UNSPECIFIED. ) 
 CURVE ( )  GEOMETRIC_REPRESENTATION_ITEM ( )  RATIONAL_B_SPLINE_CURVE ( ( 1.000000000000000000, 0.9873120399594201846, 0.9873120399594201846, 1.000000000000000000 ) ) 
 REPRESENTATION_ITEM ( '' )  );
#32295=CARTESIAN_POINT ( 'NONE',  ( 36.97963125324073275, -2.956583467688224776, 5.977963831466492906 ) ) ;
#32297=CARTESIAN_POINT ( 'NONE',  ( 87.11756278340992310, 0.5031432294147388795, -4.836983121871330837 ) ) ;
#32307=CARTESIAN_POINT ( 'NONE',  ( -80.82372619930970359, -6.607616770128094785, 1.502042499036972734 ) ) ;
#32311=CARTESIAN_POINT ( 'NONE',  ( 23.15964026960165967, 1.239783467617344037, 5.376747259291860814 ) ) ;
#32318=CARTESIAN_POINT ( 'NONE',  ( 85.15051256642057353, 2.712627394972505268, -0.4824498372492339593 ) ) ;
#32323=CARTESIAN_POINT ( 'NONE',  ( 22.20600778403895248, 3.972696832848836124, -4.026605987857512226 ) ) ;
#32324=ORIENTED_EDGE ( 'NONE', *, *, #24184, .F. ) ;
#32327=CARTESIAN_POINT ( 'NONE',  ( 21.85643539959775694, 5.081979399238238493, 12.23420521612613143 ) ) ;
#32329=CARTESIAN_POINT ( 'NONE',  ( 18.10407751945326638, 13.71956107779235268, -3.198739209383718585 ) ) ;
#32333=CARTESIAN_POINT ( 'NONE',  ( 86.63338141420044280, 0.5786414684654883622, -5.958757720264261870 ) ) ;
#32335=ORIENTED_EDGE ( 'NONE', *, *, #7909, .F. ) ;
#32337=CARTESIAN_POINT ( 'NONE',  ( 33.11221513172080932, -3.162643624533764353, 5.374360011888029476 ) ) ;
#32338=CARTESIAN_POINT ( 'NONE',  ( 30.31286271484965766, -3.794529559310727329, 4.460666598210623057 ) ) ;
#32340=CARTESIAN_POINT ( 'NONE',  ( 31.37671975378950151, -3.077845645974021771, -5.103493985049731840 ) ) ;
#32341=CARTESIAN_POINT ( 'NONE',  ( 29.10125458543393862, 0.3582796436202419499, -4.748352613195486960 ) ) ;
#32343=CARTESIAN_POINT ( 'NONE',  ( 84.19306202100948155, 2.904934786060358487, -1.717472329190754543 ) ) ;
#32347=CARTESIAN_POINT ( 'NONE',  ( 33.43971231075012440, -3.588053834546123255, 5.336497937005737491 ) ) ;
#32348=ORIENTED_EDGE ( 'NONE', *, *, #3214, .T. ) ;
#32350=CARTESIAN_POINT ( 'NONE',  ( 33.45677177907953848, -3.832870168856042703, 5.089957537689628886 ) ) ;
#32353=CARTESIAN_POINT ( 'NONE',  ( 87.44940651735645076, -1.930920027091641122, 3.725338843608501094 ) ) ;
#32354=VERTEX_POINT ( 'NONE', #23401 ) ;
#32372=CARTESIAN_POINT ( 'NONE',  ( 25.83191277475825132, 1.872540234882475785, -4.238092754309072951 ) ) ;
#32376=CARTESIAN_POINT ( 'NONE',  ( 28.41236345070440805, -1.224654026667450157, -6.045523132457580218 ) ) ;
#32387=CARTESIAN_POINT ( 'NONE',  ( 32.98356798830028680, -0.3891095675782572649, -5.239434360015620129 ) ) ;
#32389=DIRECTION ( 'NONE',  ( 0.000000000000000000, 1.000000000000000000, -0.000000000000000000 ) ) ;
#32396=CARTESIAN_POINT ( 'NONE',  ( 29.26500471863120367, 0.8173314802168033522, 4.740106445390345868 ) ) ;
#32403=CARTESIAN_POINT ( 'NONE',  ( 22.57817341642408238, 3.872950795758598463, 3.791059833831656345 ) ) ;
#32413=CARTESIAN_POINT ( 'NONE',  ( 24.74432928415070521, 0.5874317898091796497, 4.777574746359165125 ) ) ;
#32419=CARTESIAN_POINT ( 'NONE',  ( 24.68629359590044459, -1.668547755296895696, 6.687296101055469677 ) ) ;
#32423=CARTESIAN_POINT ( 'NONE',  ( -80.18991991861095414, -5.669444215152338096, 3.791920745091341249 ) ) ;
#32425=CARTESIAN_POINT ( 'NONE',  ( -70.92837670882107659, 13.87661300689599386, 0.000000000000000000 ) ) ;
#32426=DIRECTION ( 'NONE',  ( -0.000000000000000000, -0.000000000000000000, 1.000000000000000000 ) ) ;
#32428=CARTESIAN_POINT ( 'NONE',  ( 30.88365314066634326, 0.6996741485792697945, -4.491056140736914060 ) ) ;
#32435=CIRCLE ( 'NONE', #5468, 10.00000000000000888 ) ;
#32443=CARTESIAN_POINT ( 'NONE',  ( 84.96089493372460311, 1.928984934743871449, -4.835719925821683418 ) ) ;
#32446=CARTESIAN_POINT ( 'NONE',  ( -73.39348799458949202, 5.379232413676362512, -10.89378155313290897 ) ) ;
#32448=DIRECTION ( 'NONE',  ( -0.000000000000000000, -0.000000000000000000, -1.000000000000000000 ) ) ;
#32463=CARTESIAN_POINT ( 'NONE',  ( 33.87028684928710476, -5.289643708110279618, -1.965944456772101390 ) ) ;
#32470=CARTESIAN_POINT ( 'NONE',  ( -74.88476387340585916, -2.943434482340918645, -9.227807331241843158 ) ) ;
#32485=CARTESIAN_POINT ( 'NONE',  ( 35.86950732074304682, -2.085441397799345786, 5.804702143351438970 ) ) ;
#32488=CARTESIAN_POINT ( 'NONE',  ( 87.34032947353671261, 0.2529211099193515166, 5.122688537971352929 ) ) ;
#32491=CARTESIAN_POINT ( 'NONE',  ( -70.73005440458344140, -48.61702805680356931, 10.00000000000000533 ) ) ;
#32507=CARTESIAN_POINT ( 'NONE',  ( 22.77511887918089784, 1.984009684073128943, 5.106421591786454606 ) ) ;
#32508=ORIENTED_EDGE ( 'NONE', *, *, #16507, .F. ) ;
#32509=EDGE_CURVE ( 'NONE', #12694, #8980, #31150, .T. ) ;
#32512=CARTESIAN_POINT ( 'NONE',  ( 14.77315594796849574, 13.19392823276453441, -2.500000000000005773 ) ) ;
#32518=CARTESIAN_POINT ( 'NONE',  ( 22.55565315994001097, 4.076294750019800794, -3.649699173882503977 ) ) ;
#32522=CARTESIAN_POINT ( 'NONE',  ( 21.85643539959775339, -5.954433958055524556, -11.26730592371362505 ) ) ;
#32523=CARTESIAN_POINT ( 'NONE',  ( 21.80882946371355047, 5.293150380064015614, -3.367598806138242917 ) ) ;
#32526=CARTESIAN_POINT ( 'NONE',  ( 88.25293897076788596, -0.9571425830051931705, -4.167473131139645126 ) ) ;
#32529=CARTESIAN_POINT ( 'NONE',  ( -80.25993260945720920, -5.625204836179395151, 5.971172885161660560 ) ) ;
#32531=CARTESIAN_POINT ( 'NONE',  ( 15.04281356191366292, -4.011470685753230292, 2.554192886794166117 ) ) ;
#32536=CARTESIAN_POINT ( 'NONE',  ( 31.71772644211463188, -0.5622319885707789400, -5.156716326041481224 ) ) ;
#32538=CARTESIAN_POINT ( 'NONE',  ( 84.47597663471815110, 2.555392163460764809, -3.359472611266297815 ) ) ;
#32545=CARTESIAN_POINT ( 'NONE',  ( 37.00854049623069386, -3.246023182758657200, 5.947063170885879657 ) ) ;
#32549=CARTESIAN_POINT ( 'NONE',  ( 87.92225447513270353, -2.506640933623296430, 0.2833183356762295491 ) ) ;
#32554=ORIENTED_EDGE ( 'NONE', *, *, #39961, .F. ) ;
#32558=CARTESIAN_POINT ( 'NONE',  ( 22.14223375496702317, 4.765437392088810675, 3.533749582433190817 ) ) ;
#32580=CARTESIAN_POINT ( 'NONE',  ( 32.04447592720433136, -5.114560573210904515, 0.4782324236124577688 ) ) ;
#32582=CARTESIAN_POINT ( 'NONE',  ( -70.12927831234416942, -21.39817538196428615, 9.968450010350149881 ) ) ;
#32586=CARTESIAN_POINT ( 'NONE',  ( 29.26503589862772969, 0.8173198370404799462, -4.740111391064184332 ) ) ;
#32591=B_SPLINE_CURVE_WITH_KNOTS ( 'NONE', 3,
 ( #22422, #31892, #37626, #34589, #9641, #31076, #6767, #28798, #6364, #9023, #15826, #24827, #601, #2884 ),
 .UNSPECIFIED., .F., .F.,
 ( 4, 2, 2, 2, 2, 2, 4 ),
 ( 0.000000000000000000, 2.311601343512421228E-05, 4.623202687024842455E-05, 9.246405374049915303E-05, 0.0001849281074810030223, 0.0003698562149620148267, 0.0007397124299240395197 ),
 .UNSPECIFIED. ) ;
#32596=CARTESIAN_POINT ( 'NONE',  ( 29.34598460277089060, 0.9961803144104202090, 4.626948874399350764 ) ) ;
#32603=CARTESIAN_POINT ( 'NONE',  ( 30.74057244063293481, -3.574220798478507710, 4.805827853833087637 ) ) ;
#32604=CARTESIAN_POINT ( 'NONE',  ( 85.45652069754405034, 1.208412679805325407, -5.653737850026661071 ) ) ;
#32610=CARTESIAN_POINT ( 'NONE',  ( 24.74156297819196482, 3.012697116509819306, 3.382074263075999010 ) ) ;
#32616=ORIENTED_EDGE ( 'NONE', *, *, #28742, .F. ) ;
#32618=CARTESIAN_POINT ( 'NONE',  ( 21.78676948381099976, 0.2189784557031426993, 8.380332209910813290 ) ) ;
#32629=CARTESIAN_POINT ( 'NONE',  ( 24.43802896994273510, -0.4903351684736660387, 6.966919456710074954 ) ) ;
#32631=CARTESIAN_POINT ( 'NONE',  ( -74.78555365388220366, -2.834168353914430671, 10.55874562434718378 ) ) ;
#32632=CARTESIAN_POINT ( 'NONE',  ( 26.06260999411897217, 0.7785562455270252924, -4.421375452052825672 ) ) ;
#32635=CARTESIAN_POINT ( 'NONE',  ( 4.200390093233091093, -29.56993018339339940, -15.49999999999999822 ) ) ;
#32636=CARTESIAN_POINT ( 'NONE',  ( 33.11348551397914974, -0.1515143186654732133, -4.942515107159420218 ) ) ;
#32640=PLANE ( 'NONE',  #24549 ) ;
#32648=CARTESIAN_POINT ( 'NONE',  ( 86.89103086197154369, -0.8412156502217053022, -5.497997349500185926 ) ) ;
#32651=CARTESIAN_POINT ( 'NONE',  ( -77.50089735354119114, 9.756467026281873345, -9.131598822715689678 ) ) ;
#32657=ADVANCED_FACE ( 'NONE', ( #7275 ), #1932, .F. ) ;
#32662=CARTESIAN_POINT ( 'NONE',  ( 33.77937656451339166, -4.816664999545909431, 3.541921615443311744 ) ) ;
#32665=CARTESIAN_POINT ( 'NONE',  ( 24.13226474559606416, 2.704999742398795259, 3.972821573215394864 ) ) ;
#32668=CARTESIAN_POINT ( 'NONE',  ( 33.88647134759106194, -5.391981279974441321, -1.346411692250225833 ) ) ;
#32672=CARTESIAN_POINT ( 'NONE',  ( -73.77129911634021653, -3.508482060268308889, -9.588404479166415584 ) ) ;
#32685=CARTESIAN_POINT ( 'NONE',  ( 19.21360371875379514, 6.947362734548907071, -3.205145561710191160 ) ) ;
#32689=CARTESIAN_POINT ( 'NONE',  ( 37.04408834714948995, -2.892981267788033772, 5.988023919871666934 ) ) ;
#32692=CARTESIAN_POINT ( 'NONE',  ( 84.90669483503786807, 2.936226605105188625, 1.856525974524364297 ) ) ;
#32699=CARTESIAN_POINT ( 'NONE',  ( 21.76158951578306144, 5.855693934973000836, 3.369080518218454667 ) ) ;
#32711=CARTESIAN_POINT ( 'NONE',  ( 24.64619019099651354, 0.7543582096408616433, 4.794156199316148559 ) ) ;
#32715=CARTESIAN_POINT ( 'NONE',  ( 39.57450465021913999, -13.08403409140692553, -6.000000000000000000 ) ) ;
#32719=CARTESIAN_POINT ( 'NONE',  ( 24.57161973902774221, 2.977233313421253413, -3.583713660848351523 ) ) ;
#32721=CARTESIAN_POINT ( 'NONE',  ( -71.92837670882107659, -0.7829914368874778541, 5.916079783099617906 ) ) ;
#32723=CARTESIAN_POINT ( 'NONE',  ( 22.53953452546943126, -1.608357795960198677, 9.096105908381383998 ) ) ;
#32724=CARTESIAN_POINT ( 'NONE',  ( 21.85643539959980330, 4.658110446274656091, 2.545489860561468118E-12 ) ) ;
#32725=CARTESIAN_POINT ( 'NONE',  ( 15.43177744199658896, 12.90197810732775885, 2.500000000000005773 ) ) ;
#32728=CARTESIAN_POINT ( 'NONE',  ( 84.80723110164849743, 2.854080505324299466, 2.680610459220619912 ) ) ;
#32731=CARTESIAN_POINT ( 'NONE',  ( -80.03623703158197600, -5.604753948939747765, 6.344040936181177592 ) ) ;
#32734=CARTESIAN_POINT ( 'NONE',  ( 21.79474914018651788, 6.321282727555548320, -2.730181469529505023 ) ) ;
#32735=CARTESIAN_POINT ( 'NONE',  ( 28.89366916224668813, -3.006935889917436988, -4.715953887435873959 ) ) ;
#32736=CARTESIAN_POINT ( 'NONE',  ( 36.78886185490619454, -3.040240986573045756, -5.948189653081061401 ) ) ;
#32738=CARTESIAN_POINT ( 'NONE',  ( 84.49114003401015793, 2.536390008004397068, -3.421698485768037923 ) ) ;
#32745=EDGE_CURVE ( 'NONE', #20794, #17373, #27044, .T. ) ;
#32750=CARTESIAN_POINT ( 'NONE',  ( 36.68534330363475959, -1.915002933638632054, 5.803249200901428040 ) ) ;
#32753=CARTESIAN_POINT ( 'NONE',  ( 86.00054146471580907, 0.2529338399765344580, 5.999804812770356932 ) ) ;
#32759=DIRECTION ( 'NONE',  ( -0.000000000000000000, -0.000000000000000000, -1.000000000000000000 ) ) ;
#32762=EDGE_LOOP ( 'NONE', ( #16296, #5952, #39093, #35217 ) ) ;
#32763=CARTESIAN_POINT ( 'NONE',  ( 23.88456871391472092, 3.166956515880607892, 3.639194615745996675 ) ) ;
#32772=CARTESIAN_POINT ( 'NONE',  ( 23.83171675590329386, 2.746212528099347683, -4.025696239093874418 ) ) ;
#32775=CARTESIAN_POINT ( 'NONE',  ( 16.11725891507163766, 15.27317977277692052, -2.500000000000000000 ) ) ;
#32776=FACE_OUTER_BOUND ( 'NONE', #15415, .T. ) ;
#32780=CARTESIAN_POINT ( 'NONE',  ( 86.46420362610733434, 1.237027245193318192, -5.068583899740296772 ) ) ;
#32781=CARTESIAN_POINT ( 'NONE',  ( 31.96174557538834193, -4.583587016071825282, 3.235063174744643000 ) ) ;
#32784=CARTESIAN_POINT ( 'NONE',  ( -81.53531961795309257, -5.628198604101866565, -2.656554173279100262 ) ) ;
#32788=CARTESIAN_POINT ( 'NONE',  ( 37.00281670377963650, -2.989080459751201069, -5.981582481765331138 ) ) ;
#32793=CARTESIAN_POINT ( 'NONE',  ( 11.29080664838499182, -35.94265729135299381, 2.500000000000000000 ) ) ;
#32796=CARTESIAN_POINT ( 'NONE',  ( 34.78032543754396499, -3.716931077528784044, 5.478572017771286440 ) ) ;
#32807=FACE_OUTER_BOUND ( 'NONE', #26752, .T. ) ;
#32810=CARTESIAN_POINT ( 'NONE',  ( 22.38279560817339586, 4.933722530806304185, 3.054152587046873979 ) ) ;
#32817=CARTESIAN_POINT ( 'NONE',  ( 26.05852442447088890, 0.7874726545580505999, 4.421626571207251999 ) ) ;
#32824=CARTESIAN_POINT ( 'NONE',  ( 24.14839210154553584, 1.598524049810922998, 6.350534879451781300 ) ) ;
#32827=CARTESIAN_POINT ( 'NONE',  ( -79.18352549070058899, -5.465004164923950469, 7.520925182975014778 ) ) ;
#32828=CARTESIAN_POINT ( 'NONE',  ( 27.40045544475674077, 1.045213952888590203, -4.482696246924063210 ) ) ;
#32833=EDGE_CURVE ( 'NONE', #141, #40670, #39983, .T. ) ;
#32834=CARTESIAN_POINT ( 'NONE',  ( 35.83198913069367819, -3.726957495236238760, -5.625159356461098881 ) ) ;
#32838=CARTESIAN_POINT ( 'NONE',  ( -71.12575595825015284, -48.60721477804613500, 5.997525359197725336 ) ) ;
#32845=EDGE_LOOP ( 'NONE', ( #30835, #5543, #31961, #9259 ) ) ;
#32851=CARTESIAN_POINT ( 'NONE',  ( -79.56308247960363644, 10.39758802068803689, -7.037846573057998434 ) ) ;
#32860=CARTESIAN_POINT ( 'NONE',  ( 33.84452642184018600, -5.136433483475361328, 2.685500998610346191 ) ) ;
#32865=CARTESIAN_POINT ( 'NONE',  ( 17.03316807477964190, 9.497738621113558821, -2.806674216866353433 ) ) ;
#32867=CARTESIAN_POINT ( 'NONE',  ( 21.85643539959777115, -1.425092139247138734, 16.06258187428232986 ) ) ;
#32870=CARTESIAN_POINT ( 'NONE',  ( 14.68539687963933282, -4.701488008871138824, 2.500000000000806466 ) ) ;
#32871=CARTESIAN_POINT ( 'NONE',  ( -75.97102281476716712, -3.971666016424915124, -8.662871507693417072 ) ) ;
#32889=CARTESIAN_POINT ( 'NONE',  ( 36.91179562721963947, -2.638184243151847852, 5.967376441415058075 ) ) ;
#32890=CARTESIAN_POINT ( 'NONE',  ( 14.61802081865033642, 12.33286846116284252, -2.500000000000000000 ) ) ;
#32891=CARTESIAN_POINT ( 'NONE',  ( 87.10205511408864254, 0.5205621796347451591, 5.292648712017772539 ) ) ;
#32898=CARTESIAN_POINT ( 'NONE',  ( -78.06330667992513384, 11.25813893609656802, -7.018729043671574352 ) ) ;
#32899=CARTESIAN_POINT ( 'NONE',  ( 24.31240841717447410, -6.336097543977142976, -2.705716385158337012 ) ) ;
#32905=CARTESIAN_POINT ( 'NONE',  ( 21.75407835734251805, 0.6912123640297617166, 8.027689290590526383 ) ) ;
#32909=CARTESIAN_POINT ( 'NONE',  ( 14.69558838330753758, 3.996311804371543985, -6.000000000000000000 ) ) ;
#32913=CARTESIAN_POINT ( 'NONE',  ( 23.17722939410916183, 3.712341236063878114, -3.488222722305598822 ) ) ;
#32915=CARTESIAN_POINT ( 'NONE',  ( 1.700390093233090871, -29.56993018339339940, 27.90461065042423527 ) ) ;
#32916=CARTESIAN_POINT ( 'NONE',  ( 22.31759743831440090, 6.226164879696757026, 1.431367841762869686 ) ) ;
#32918=CARTESIAN_POINT ( 'NONE',  ( 16.61473264793675853, 9.888384249099596346, 2.499999999999963585 ) ) ;
#32922=CARTESIAN_POINT ( 'NONE',  ( 86.35968278939613185, 0.3242946576005459325, -6.017936684944984016 ) ) ;
#32929=CARTESIAN_POINT ( 'NONE',  ( 18.21053797601233981, -2.853449834380734185, -3.048592893318725405 ) ) ;
#32931=CARTESIAN_POINT ( 'NONE',  ( 36.63295709802978450, -3.078046445090460992, -5.923856945199692525 ) ) ;
#32933=CARTESIAN_POINT ( 'NONE',  ( 84.54498636705716308, 2.468675992724178592, -3.632217660620454147 ) ) ;
#32939=CARTESIAN_POINT ( 'NONE',  ( 31.83101670608917644, -2.965446787480832569, -5.174398011670120034 ) ) ;
#32942=CARTESIAN_POINT ( 'NONE',  ( 37.00966539048157955, -2.249461300321922597, 5.913205627773911566 ) ) ;
#32945=CARTESIAN_POINT ( 'NONE',  ( 33.46455515056310759, -3.089188617792877789, 5.429351193206847448 ) ) ;
#32946=CARTESIAN_POINT ( 'NONE',  ( 87.82805078818662992, -2.393880730231491061, -1.766410623985958050 ) ) ;
#32948=ORIENTED_EDGE ( 'NONE', *, *, #32745, .T. ) ;
#32949=AXIS2_PLACEMENT_3D ( 'NONE', #38130, #31770, #28057 ) ;
#32952=DIRECTION ( 'NONE',  ( 1.000000000000000000, -8.959828616340678715E-16, 0.000000000000000000 ) ) ;
#32956=CARTESIAN_POINT ( 'NONE',  ( 23.41651709676641246, 3.612060057188777318, 3.413386634271887932 ) ) ;
#32959=VERTEX_POINT ( 'NONE', #6830 ) ;
#32961=CARTESIAN_POINT ( 'NONE',  ( 16.18297655557976711, -3.318851087015777690, -2.732142896901965656 ) ) ;
#32962=CARTESIAN_POINT ( 'NONE',  ( -72.84815947045233031, 2.429809908903243443, 12.50000000000000000 ) ) ;
#32964=ORIENTED_EDGE ( 'NONE', *, *, #36302, .T. ) ;
#32965=CARTESIAN_POINT ( 'NONE',  ( 23.54860076899586119, 2.870803210893150048, -4.024937523241188586 ) ) ;
#32974=CARTESIAN_POINT ( 'NONE',  ( 88.37152744968734908, -0.9053694005015545665, 0.1944390934057901588 ) ) ;
#32975=CARTESIAN_POINT ( 'NONE',  ( 28.89923929355584065, 0.07307017450661948410, 5.719397691353443669 ) ) ;
#32978=CARTESIAN_POINT ( 'NONE',  ( -77.35749566552371448, -4.820597592931324726, -9.230088820010045936 ) ) ;
#32983=CARTESIAN_POINT ( 'NONE',  ( 32.84225399592710914, -0.7495783096613907182, -5.332226047615563402 ) ) ;
#32990=CARTESIAN_POINT ( 'NONE',  ( 34.51602972922534462, -1.013642683923393184, 5.504862190214542927 ) ) ;
#32991=CARTESIAN_POINT ( 'NONE',  ( -62.92837670882106238, -42.37473357531882812, -6.000000000000000000 ) ) ;
#32999=CARTESIAN_POINT ( 'NONE',  ( 84.97506497612948806, 1.907738733390036856, -4.849904034997914337 ) ) ;
#33004=CARTESIAN_POINT ( 'NONE',  ( 22.61565167955079758, 4.617847287593741079, 3.051803804880747872 ) ) ;
#33010=CARTESIAN_POINT ( 'NONE',  ( 22.28556628514242988, 0.2471207394018046788, 7.129339672946321649 ) ) ;
#33011=CARTESIAN_POINT ( 'NONE',  ( 14.74217871668694890, -5.108457001575695600, -2.500000000000635936 ) ) ;
#33020=CARTESIAN_POINT ( 'NONE',  ( 37.83867290611771494, -6.084034091406928191, -6.000000000000000000 ) ) ;
#33021=CARTESIAN_POINT ( 'NONE',  ( 27.87470673840761037, 2.608020033772324275, -0.5247038454205935620 ) ) ;
#33024=CARTESIAN_POINT ( 'NONE',  ( -80.83093704390071821, -5.699917940215170731, 1.450021397597311301 ) ) ;
#33025=CARTESIAN_POINT ( 'NONE',  ( 23.59548752951696571, 0.4310456963235400618, -5.519663247815086216 ) ) ;
#33028=CARTESIAN_POINT ( 'NONE',  ( 37.21106504267930148, -2.744214598291488727, -6.000909659284667796 ) ) ;
#33032=CARTESIAN_POINT ( 'NONE',  ( -72.38866088156714795, -47.51164815211338066, 5.820093912444312956 ) ) ;
#33033=DIRECTION ( 'NONE',  ( 1.682730792515357087E-16, -1.000000000000000000, 0.000000000000000000 ) ) ;
#33036=CARTESIAN_POINT ( 'NONE',  ( 23.51788449541176007, 1.295866407298160716, -5.129232269930078303 ) ) ;
#33043=CARTESIAN_POINT ( 'NONE',  ( 84.21289197705223728, 3.045783863710543660, -0.4930364517660317802 ) ) ;
#33050=FACE_OUTER_BOUND ( 'NONE', #12577, .T. ) ;
#33052=CARTESIAN_POINT ( 'NONE',  ( 30.67349724481533002, -3.593355625737403525, 4.777428303402127874 ) ) ;
#33057=CARTESIAN_POINT ( 'NONE',  ( 33.81811101054934454, -4.997128391572976724, 3.084473742510627670 ) ) ;
#33061=EDGE_CURVE ( 'NONE', #5866, #28854, #29952, .T. ) ;
#33064=CARTESIAN_POINT ( 'NONE',  ( 16.15319511113404261, 10.47632875577966338, -2.684738856704420584 ) ) ;
#33066=CARTESIAN_POINT ( 'NONE',  ( 21.85643539959774273, 10.29907807357824723, -3.463423532579224418 ) ) ;
#33068=CARTESIAN_POINT ( 'NONE',  ( -76.77456831373793023, 10.78129903716225790, 8.115337217677211612 ) ) ;
#33070=CARTESIAN_POINT ( 'NONE',  ( 14.75304912753043496, -4.607437571476275195, 2.508639535167287882 ) ) ;
#33071=CARTESIAN_POINT ( 'NONE',  ( -73.03883085241794504, 7.296995364254068583, -9.776882264804946487 ) ) ;
#33073=CARTESIAN_POINT ( 'NONE',  ( 37.18716061172991516, -2.963873844666090829, -6.000015731507488681 ) ) ;
#33078=CARTESIAN_POINT ( 'NONE',  ( -70.79792407645882690, 0.2170085631122713188, 9.999999999999980460 ) ) ;
#33083=CARTESIAN_POINT ( 'NONE',  ( 22.92221885755501631, 2.655821486554086786, 3.783964647315853469 ) ) ;
#33087=CARTESIAN_POINT ( 'NONE',  ( 88.25986434197210428, -0.7799440980648532085, -3.332403339731401015 ) ) ;
#33089=CARTESIAN_POINT ( 'NONE',  ( 33.61655304153408252, -1.223667153998024171, -5.453074140175755424 ) ) ;
#33090=LINE ( 'NONE', #39040, #30041 ) ;
#33099=ORIENTED_EDGE ( 'NONE', *, *, #628, .T. ) ;
#33103=CARTESIAN_POINT ( 'NONE',  ( 22.83213583935611624, 0.9805358558969262672, 5.835874598331055374 ) ) ;
#33107=ADVANCED_FACE ( 'NONE', ( #26379 ), #7228, .F. ) ;
#33112=DIRECTION ( 'NONE',  ( 1.000000000000000000, 1.776143608908745286E-15, 0.000000000000000000 ) ) ;
#33116=CARTESIAN_POINT ( 'NONE',  ( 22.27850866888861958, 4.871699234913689835, -3.307860320298297019 ) ) ;
#33120=CARTESIAN_POINT ( 'NONE',  ( 22.79820677575384380, -6.119817767430131283, -4.702819652331462486 ) ) ;
#33121=CARTESIAN_POINT ( 'NONE',  ( 21.88097534391988219, 3.372061099782372562, 3.393279653752791614 ) ) ;
#33125=CARTESIAN_POINT ( 'NONE',  ( 84.70654116317179216, 2.970325471579660981, -2.062712134826208299 ) ) ;
#33131=CARTESIAN_POINT ( 'NONE',  ( 17.02371012435539299, -3.136981811050143953, -2.862043499008697811 ) ) ;
#33132=CARTESIAN_POINT ( 'NONE',  ( 34.33178807571479751, -1.489136665238962154, -5.564703865284172934 ) ) ;
#33134=CARTESIAN_POINT ( 'NONE',  ( 22.39197674124670456, 0.3416523442181764736, -6.896521180731577161 ) ) ;
#33140=CARTESIAN_POINT ( 'NONE',  ( 31.83665345065898222, -2.965757740674789922, -5.175277761985421776 ) ) ;
#33143=CARTESIAN_POINT ( 'NONE',  ( 35.36852012591459982, -3.795115921518204871, 5.508735250874407186 ) ) ;
#33145=CARTESIAN_POINT ( 'NONE',  ( 14.74516149780720475, 13.12656125137930196, -2.500000000000006217 ) ) ;
#33153=VERTEX_POINT ( 'NONE', #18097 ) ;
#33157=ORIENTED_EDGE ( 'NONE', *, *, #6520, .F. ) ;
#33158=CARTESIAN_POINT ( 'NONE',  ( 23.41639419491407637, 3.441844816758488967, 3.597223659465575984 ) ) ;
#33164=DIRECTION ( 'NONE',  ( -0.000000000000000000, -0.000000000000000000, -1.000000000000000000 ) ) ;
#33168=CARTESIAN_POINT ( 'NONE',  ( 23.64026257316363555, 2.651593249435279631, -4.149758956619620243 ) ) ;
#33169=ORIENTED_EDGE ( 'NONE', *, *, #22150, .T. ) ;
#33171=CARTESIAN_POINT ( 'NONE',  ( 23.06594672544511582, -8.086844732617873177, 2.500000000000001332 ) ) ;
#33176=CARTESIAN_POINT ( 'NONE',  ( 87.18327248044521127, 0.4293349789342923994, 4.780712506200352152 ) ) ;
#33177=CARTESIAN_POINT ( 'NONE',  ( 32.03962978398497796, -5.076534887360421244, -0.9488177176524058565 ) ) ;
#33181=CARTESIAN_POINT ( 'NONE',  ( -76.43695570392601724, -4.296655540762186476, -9.829794133232820030 ) ) ;
#33184=CARTESIAN_POINT ( 'NONE',  ( 25.38653250821387175, 1.982128556287479304, -4.168580392152317238 ) ) ;
#33187=( BOUNDED_CURVE ( )  B_SPLINE_CURVE ( 3, ( #11502, #29651, #30061, #30469 ),
 .UNSPECIFIED., .F., .T. ) 
 B_SPLINE_CURVE_WITH_KNOTS ( ( 4, 4 ),
 ( 2.498091544796509300, 3.785093762383078708 ),
 .UNSPECIFIED. ) 
 CURVE ( )  GEOMETRIC_REPRESENTATION_ITEM ( )  RATIONAL_B_SPLINE_CURVE ( ( 1.000000000000000000, 0.8666666666666664742, 0.8666666666666664742, 1.000000000000000000 ) ) 
 REPRESENTATION_ITEM ( '' )  );
#33193=CARTESIAN_POINT ( 'NONE',  ( 37.07822424304627162, -3.092072612053704539, 5.980643640684182749 ) ) ;
#33201=CARTESIAN_POINT ( 'NONE',  ( 85.31284572182654813, 1.429488415003690838, -5.464460692432248301 ) ) ;
#33208=CARTESIAN_POINT ( 'NONE',  ( 21.99446821316316303, 5.584237617783551322, 3.108634153913448994 ) ) ;
#33210=AXIS2_PLACEMENT_3D ( 'NONE', #35645, #20174, #23662 ) ;
#33212=CARTESIAN_POINT ( 'NONE',  ( 16.75050750990541104, 0.9041099969468745501, -4.803821987783263303 ) ) ;
#33216=CARTESIAN_POINT ( 'NONE',  ( 26.76860462860027923, 0.8092645171851360342, 4.384286172079291610 ) ) ;
#33222=CARTESIAN_POINT ( 'NONE',  ( 87.04213330793392345, 0.5878691963682424193, 0.000000000000000000 ) ) ;
#33223=CARTESIAN_POINT ( 'NONE',  ( 39.57450465021913999, -13.08403409140692553, -6.000000000000000000 ) ) ;
#33224=CARTESIAN_POINT ( 'NONE',  ( 29.14988983353436680, -2.161137664473038900, -5.740130334263455758 ) ) ;
#33225=CARTESIAN_POINT ( 'NONE',  ( 14.77044403067345257, -5.165496212256374342, -2.499999999999999556 ) ) ;
#33226=FACE_OUTER_BOUND ( 'NONE', #14381, .T. ) ;
#33229=CARTESIAN_POINT ( 'NONE',  ( 24.74515534416565288, 0.5823800272612684736, -4.777517428576818048 ) ) ;
#33236=CARTESIAN_POINT ( 'NONE',  ( 35.21907562575142947, -1.051044697053814314, -5.414479983419766995 ) ) ;
#33237=CARTESIAN_POINT ( 'NONE',  ( 30.88512837779606102, -3.430581993324693268, -4.934071252754470116 ) ) ;
#33240=FACE_OUTER_BOUND ( 'NONE', #27433, .T. ) ;
#33243=VECTOR ( 'NONE', #343, 1000.000000000000000 ) ;
#33247=CARTESIAN_POINT ( 'NONE',  ( -69.61816732119611117, -47.87313727245317097, 5.855707401755813279 ) ) ;
#33253=CARTESIAN_POINT ( 'NONE',  ( 86.84125380892929513, -1.134812445414097981, 5.244953511127716794 ) ) ;
#33260=CARTESIAN_POINT ( 'NONE',  ( 24.59436848130510356, -3.190661413691112447, 3.914729585663517142 ) ) ;
#33261=AXIS2_PLACEMENT_3D ( 'NONE', #996, #23209, #19718 ) ;
#33266=CARTESIAN_POINT ( 'NONE',  ( 15.27436600411698997, 8.240067691444819431, -3.484044305282195442 ) ) ;
#33273=CARTESIAN_POINT ( 'NONE',  ( 16.65948297789018895, 14.84918060193631995, 2.499999999999999556 ) ) ;
#33275=CARTESIAN_POINT ( 'NONE',  ( 21.85643539959775339, 7.579478879252558698, 11.98046644763472024 ) ) ;
#33279=CARTESIAN_POINT ( 'NONE',  ( 14.76777200802055212, -5.161570699583752919, 2.499999999979765963 ) ) ;
#33280=CARTESIAN_POINT ( 'NONE',  ( -79.69001610741072739, 10.46859553514188867, -4.835689715862597993 ) ) ;
#33281=DIRECTION ( 'NONE',  ( -1.000000000000000000, 0.000000000000000000, 0.000000000000000000 ) ) ;
#33296=CARTESIAN_POINT ( 'NONE',  ( 37.01034345348816856, -2.703823390587133169, 5.982757213092503079 ) ) ;
#33301=CARTESIAN_POINT ( 'NONE',  ( 85.21894181876761820, 2.635764410888131959, 2.550537924818469637 ) ) ;
#33303=CARTESIAN_POINT ( 'NONE',  ( 31.21770016481918475, -0.3792164351781658338, -5.078675132288333671 ) ) ;
#33310=ORIENTED_EDGE ( 'NONE', *, *, #40244, .F. ) ;
#33315=CARTESIAN_POINT ( 'NONE',  ( 21.94773631808104497, 0.8018986738919260393, 7.249714582973164845 ) ) ;
#33326=VECTOR ( 'NONE', #19505, 1000.000000000000000 ) ;
#33327=CARTESIAN_POINT ( 'NONE',  ( 22.50262521106708746, 4.464923929019867010, -3.378628388999005860 ) ) ;
#33333=CARTESIAN_POINT ( 'NONE',  ( 22.33594428049882197, 5.124660873843202680, 5.347558210918236909 ) ) ;
#33336=LINE ( 'NONE', #14764, #37973 ) ;
#33337=VECTOR ( 'NONE', #28866, 1000.000000000000000 ) ;
#33346=CARTESIAN_POINT ( 'NONE',  ( 28.88852978429638796, -3.262707939826073655, -4.666690105132320632 ) ) ;
#33347=CARTESIAN_POINT ( 'NONE',  ( 35.86815174039828946, -2.088852906378757091, -5.804490572253821590 ) ) ;
#33349=CARTESIAN_POINT ( 'NONE',  ( 21.74205696664383680, 0.4458481429987432576, -8.549212226879914667 ) ) ;
#33352=CARTESIAN_POINT ( 'NONE',  ( 35.33522112941847837, -3.167697025310678871, 5.721313861434861536 ) ) ;
#33359=CARTESIAN_POINT ( 'NONE',  ( 35.73193773234398662, -1.301360303042222721, 5.535510931126363054 ) ) ;
#33362=CARTESIAN_POINT ( 'NONE',  ( 14.77500326541903952, -5.175625724643098557, -2.499997102511863911 ) ) ;
#33367=DIRECTION ( 'NONE',  ( 1.000000000000000000, 0.000000000000000000, -0.000000000000000000 ) ) ;
#33374=CARTESIAN_POINT ( 'NONE',  ( 14.73967931769175621, -5.056389090928278485, 2.500286496908393552 ) ) ;
#33377=DIRECTION ( 'NONE',  ( 0.000000000000000000, 0.000000000000000000, 1.000000000000000000 ) ) ;
#33379=CARTESIAN_POINT ( 'NONE',  ( 23.19659671777491283, 3.528833225524024897, 3.648563265218450091 ) ) ;
#33385=CARTESIAN_POINT ( 'NONE',  ( 17.95405594424124018, -2.878999424384995898, -3.008562669219466024 ) ) ;
#33388=CARTESIAN_POINT ( 'NONE',  ( 24.07252604127487672, 2.729050162928195356, -3.962914714437188124 ) ) ;
#33390=PLANE ( 'NONE',  #33521 ) ;
#33394=CARTESIAN_POINT ( 'NONE',  ( 85.24855023725586989, 2.602506829941634514, 1.762177041774413588 ) ) ;
#33395=CARTESIAN_POINT ( 'NONE',  ( 33.19459970134796123, -3.309813850278316760, -5.543304389637502716 ) ) ;
#33399=CARTESIAN_POINT ( 'NONE',  ( -72.84815947045237294, 2.027470820963650056, -10.96147798754374669 ) ) ;
#33401=CARTESIAN_POINT ( 'NONE',  ( 19.71787932340214411, -3.013412653616829751, 3.231043527512243330 ) ) ;
#33403=CARTESIAN_POINT ( 'NONE',  ( 36.14926277598984683, -3.245532955201251291, -5.848364748053938023 ) ) ;
#33408=EDGE_CURVE ( 'NONE', #10861, #24982, #6384, .T. ) ;
#33411=ORIENTED_EDGE ( 'NONE', *, *, #27200, .F. ) ;
#33412=CARTESIAN_POINT ( 'NONE',  ( 20.88448788323691119, 4.552395270423596152, 2.802001917821514532 ) ) ;
#33418=ORIENTED_EDGE ( 'NONE', *, *, #9827, .F. ) ;
#33421=CARTESIAN_POINT ( 'NONE',  ( 84.97662400644560421, 1.905623477933771737, -4.853294916085792998 ) ) ;
#33422=CARTESIAN_POINT ( 'NONE',  ( -76.23695949607322575, 10.51077996663807035, 8.482526175063888729 ) ) ;
#33427=CARTESIAN_POINT ( 'NONE',  ( 24.05810555315960642, 3.342710263256114089, 3.230529690456637404 ) ) ;
#33433=CARTESIAN_POINT ( 'NONE',  ( 21.77774817454276146, 0.1996980602981901221, 8.433676550975363284 ) ) ;
#33445=CARTESIAN_POINT ( 'NONE',  ( 26.56136967304951213, 3.021295450130037530, 0.006841891102512360698 ) ) ;
#33450=CARTESIAN_POINT ( 'NONE',  ( 21.97292779079860026, 0.2231725819405185052, -7.728249543608548322 ) ) ;
#33452=FACE_OUTER_BOUND ( 'NONE', #18866, .T. ) ;
#33456=CARTESIAN_POINT ( 'NONE',  ( 35.36775907828450016, -3.789722492740957183, -5.512854138522889968 ) ) ;
#33459=LINE ( 'NONE', #34278, #305 ) ;
#33463=CARTESIAN_POINT ( 'NONE',  ( 14.75718030968480932, -4.580811787944012003, -2.509406477144433545 ) ) ;
#33470=CARTESIAN_POINT ( 'NONE',  ( 87.51701825761838904, -2.015745416966476800, -3.511549023785576651 ) ) ;
#33471=CIRCLE ( 'NONE', #16332, 3.000000000000002665 ) ;
#33480=CARTESIAN_POINT ( 'NONE',  ( 22.53035224700295913, 7.500703693485321288, -2.500000000000001776 ) ) ;
#33486=CARTESIAN_POINT ( 'NONE',  ( 19.16552509909860902, 12.52704827632410556, 2.500000000000000444 ) ) ;
#33489=CARTESIAN_POINT ( 'NONE',  ( 21.85643539959779957, -12.42149291456256499, -5.642648835571736576 ) ) ;
#33491=CARTESIAN_POINT ( 'NONE',  ( -78.35305259910721531, 10.09532361400513523, 8.407576680341714237 ) ) ;
#33493=CARTESIAN_POINT ( 'NONE',  ( 14.71719540082058764, -5.067275742575013453, 2.500000000000000444 ) ) ;
#33494=CARTESIAN_POINT ( 'NONE',  ( -74.22183281877552474, 6.953451750990062408, -9.495966342939334837 ) ) ;
#33502=CARTESIAN_POINT ( 'NONE',  ( -17.27251170661583402, 3.729367930467589076, 6.000000000000000000 ) ) ;
#33508=CARTESIAN_POINT ( 'NONE',  ( 35.78619758286966857, -3.165684574248104344, 5.791699643902712857 ) ) ;
#33512=CARTESIAN_POINT ( 'NONE',  ( 88.92600529607371129, -1.724176122391732680, 0.2146816905789898644 ) ) ;
#33518=EDGE_CURVE ( 'NONE', #23544, #28626, #3602, .T. ) ;
#33519=ORIENTED_EDGE ( 'NONE', *, *, #32111, .T. ) ;
#33521=AXIS2_PLACEMENT_3D ( 'NONE', #29867, #30699, #5365 ) ;
#33526=CARTESIAN_POINT ( 'NONE',  ( 21.73992701349164491, 0.3979915806805984779, 8.655561263121205329 ) ) ;
#33533=DIRECTION ( 'NONE',  ( -0.000000000000000000, -0.000000000000000000, 1.000000000000000000 ) ) ;
#33536=CARTESIAN_POINT ( 'NONE',  ( 21.75127074489211410, 5.956360602679930949, -3.331638318609325911 ) ) ;
#33539=AXIS2_PLACEMENT_3D ( 'NONE', #24882, #21383, #9415 ) ;
#33540=CARTESIAN_POINT ( 'NONE',  ( 22.31758782591801094, 6.227955964823622459, -0.6941013191108784675 ) ) ;
#33542=LINE ( 'NONE', #23636, #1158 ) ;
#33544=CARTESIAN_POINT ( 'NONE',  ( 88.77375424906220758, -2.037038645060464503, 1.247452244799444276 ) ) ;
#33550=CARTESIAN_POINT ( 'NONE',  ( 14.78586781214834822, -4.455391028847350832, -2.513676416125953939 ) ) ;
#33552=DIRECTION ( 'NONE',  ( 0.000000000000000000, 0.000000000000000000, 1.000000000000000000 ) ) ;
#33553=CARTESIAN_POINT ( 'NONE',  ( 26.61193938308475992, 1.046481346643641341, -4.377103786515438522 ) ) ;
#33556=CARTESIAN_POINT ( 'NONE',  ( 34.92821691692935104, -1.713421868941626958, 5.657791010641918916 ) ) ;
#33557=CARTESIAN_POINT ( 'NONE',  ( 87.36631219772915813, 0.2237360808920199895, 4.554730944530843040 ) ) ;
#33561=CARTESIAN_POINT ( 'NONE',  ( 34.63773063272169850, -0.7807602160518050116, 5.273885112211214476 ) ) ;
#33562=CARTESIAN_POINT ( 'NONE',  ( 14.75437388269761385, -4.625874150431743104, -2.499999999999999556 ) ) ;
#33563=CARTESIAN_POINT ( 'NONE',  ( 14.77315594796471387, 13.19392823276521298, -2.499999999999998668 ) ) ;
#33567=EDGE_LOOP ( 'NONE', ( #3454, #12391, #3647, #21835 ) ) ;
#33576=CARTESIAN_POINT ( 'NONE',  ( 24.34634393679970898, 2.915314615346324967, 3.758318930332451124 ) ) ;
#33585=ORIENTED_EDGE ( 'NONE', *, *, #40629, .F. ) ;
#33586=CARTESIAN_POINT ( 'NONE',  ( 22.24257640610459674, 3.226614291024176406, -4.542278202119804043 ) ) ;
#33587=ORIENTED_EDGE ( 'NONE', *, *, #26107, .F. ) ;
#33594=B_SPLINE_CURVE_WITH_KNOTS ( 'NONE', 3,
 ( #25338, #37872, #3532, #16056, #38680, #10675, #29822, #20544, #7397, #26147, #29626, #32529, #32731, #4909, #26937, #4330, #16850, #23256, #1440, #26541, #25135, #3538, #7005, #16651, #22863, #436, #646, #19763, #25545, #38483, #25746, #34834, #38286, #6809, #28632, #10085 ),
 .UNSPECIFIED., .F., .F.,
 ( 4, 2, 2, 2, 2, 2, 2, 2, 2, 2, 2, 2, 2, 2, 2, 2, 2, 4 ),
 ( 0.03938660120963451833, 0.04068090286293612329, 0.04197520451623773519, 0.04326950616953934015, 0.04456380782284094511, 0.04585810947614255700, 0.04715241112944416196, 0.04844671278274577386, 0.04974101443604737882, 0.05103531608934898378, 0.05232961774265058874, 0.05362391939595220064, 0.05491822104925381254, 0.05621252270255541750, 0.05750682435585702246, 0.05880112600915864129, 0.05944827683580943684, 0.06009542766246023932 ),
 .UNSPECIFIED. ) ;
#33595=CARTESIAN_POINT ( 'NONE',  ( 85.06303677129686491, 2.810884359907178442, 0.2996589496366894867 ) ) ;
#33601=CARTESIAN_POINT ( 'NONE',  ( 37.02724721148364040, -2.689435811069947224, -5.985395453346618488 ) ) ;
#33605=( BOUNDED_SURFACE ( )  B_SPLINE_SURFACE ( 3, 3, ( 
 ( #30334, #33020, #36504, #5416 ),
 ( #29914, #5009, #36702, #14263 ),
 ( #17954, #23932, #4614, #17540 ),
 ( #7889, #30539, #8485, #39580 ),
 ( #11365, #23734, #39373, #29716 ),
 ( #17749, #33223, #30128, #17144 ),
 ( #33641, #1943, #11164, #14659 ) ),
 .UNSPECIFIED., .T., .F., .T. ) 
 B_SPLINE_SURFACE_WITH_KNOTS ( ( 4, 3, 4 ),
 ( 4, 4 ),
 ( 0.000000000000000000, 0.5000000000000000000, 1.000000000000000000 ),
 ( 0.000000000000000000, 1.000000000000000000 ),
 .UNSPECIFIED. ) 
 GEOMETRIC_REPRESENTATION_ITEM ( )  RATIONAL_B_SPLINE_SURFACE ( (
 ( 1.000000000000000000, 0.9563893749471424899, 0.9563893749471424899, 1.000000000000000000),
 ( 0.3333333333333333703, 0.3187964583157141818, 0.3187964583157141818, 0.3333333333333333703),
 ( 0.3333333333333333703, 0.3187964583157141818, 0.3187964583157141818, 0.3333333333333333703),
 ( 1.000000000000000000, 0.9563893749471424899, 0.9563893749471424899, 1.000000000000000000),
 ( 0.3333333333333333703, 0.3187964583157141818, 0.3187964583157141818, 0.3333333333333333703),
 ( 0.3333333333333333703, 0.3187964583157141818, 0.3187964583157141818, 0.3333333333333333703),
 ( 1.000000000000000000, 0.9563893749471424899, 0.9563893749471424899, 1.000000000000000000) ) ) 
 REPRESENTATION_ITEM ( '' )  SURFACE ( )  );
#33610=CARTESIAN_POINT ( 'NONE',  ( 34.79207415533190328, -3.831289137303656389, 5.380522550652695024 ) ) ;
#33623=CARTESIAN_POINT ( 'NONE',  ( 24.66975522534114162, 2.992800531127576047, 3.487905392549471628 ) ) ;
#33624=AXIS2_PLACEMENT_3D ( 'NONE', #12193, #28248, #18368 ) ;
#33630=CARTESIAN_POINT ( 'NONE',  ( 26.76516748616653629, 0.8542131806872658162, 4.383548290790947100 ) ) ;
#33631=CARTESIAN_POINT ( 'NONE',  ( 14.70299449326277141, -4.943839671930780000, -2.500000000006339818 ) ) ;
#33636=CARTESIAN_POINT ( 'NONE',  ( 36.51841587071722017, -3.542906066142682775, -5.805451938871582840 ) ) ;
#33641=CARTESIAN_POINT ( 'NONE',  ( 14.69558838330753758, 3.996311804371543985, -6.000000000000000000 ) ) ;
#33642=CARTESIAN_POINT ( 'NONE',  ( 32.02118327030063227, -4.941963151977918578, 1.942379491845174444 ) ) ;
#33646=CARTESIAN_POINT ( 'NONE',  ( 27.38334305430047166, 1.066451547753710871, -4.479821203429939835 ) ) ;
#33651=CARTESIAN_POINT ( 'NONE',  ( 29.48746289019463518, 1.218344962496953565, -4.224834120391865788 ) ) ;
#33653=CARTESIAN_POINT ( 'NONE',  ( 27.42865362376633698, 1.027713267802376818, -4.487302781120154016 ) ) ;
#33657=CARTESIAN_POINT ( 'NONE',  ( -72.87830298647827476, 3.234560164695657214, 10.95879046326537676 ) ) ;
#33661=CARTESIAN_POINT ( 'NONE',  ( -70.53757485429949270, -48.56857388652895224, 5.988040939572852217 ) ) ;
#33665=ORIENTED_EDGE ( 'NONE', *, *, #3882, .F. ) ;
#33666=CARTESIAN_POINT ( 'NONE',  ( 85.28844081106248609, 1.468752784057639094, 5.439171570854275828 ) ) ;
#33672=CARTESIAN_POINT ( 'NONE',  ( -60.92837670882106238, -37.87473357531881391, 0.000000000000000000 ) ) ;
#33679=CARTESIAN_POINT ( 'NONE',  ( 15.85384049071795332, 7.981620597509389015, -3.484773916741112476 ) ) ;
#33686=CARTESIAN_POINT ( 'NONE',  ( 21.85643539959775694, 0.3794388012242833064, 14.22155525766799045 ) ) ;
#33688=CARTESIAN_POINT ( 'NONE',  ( -80.90861860399087391, 11.45717611192839591, 0.6283086135788882309 ) ) ;
#33689=CARTESIAN_POINT ( 'NONE',  ( 14.69558838330748785, -4.461849342347332659, 2.499999999999996891 ) ) ;
#33690=CARTESIAN_POINT ( 'NONE',  ( -74.89083676646993126, 9.557107727799328600, -9.187685426891615492 ) ) ;
#33692=CARTESIAN_POINT ( 'NONE',  ( 35.83269171260823782, -3.732037575501295112, -5.621802225981361367 ) ) ;
#33694=CARTESIAN_POINT ( 'NONE',  ( 14.77286119241257722, 13.14530852789250304, 2.499563476182618427 ) ) ;
#33696=CARTESIAN_POINT ( 'NONE',  ( 31.24733724172370586, -0.3895753884219697039, 5.083300714914697593 ) ) ;
#33700=CARTESIAN_POINT ( 'NONE',  ( 87.30211668890848387, 0.2958435233019774402, 4.630501607711047463 ) ) ;
#33701=CARTESIAN_POINT ( 'NONE',  ( 26.36036888033374126, 1.773289138066936665, -4.282619303848153258 ) ) ;
#33702=ORIENTED_EDGE ( 'NONE', *, *, #30995, .F. ) ;
#33704=CARTESIAN_POINT ( 'NONE',  ( 36.64688567981695400, -2.460106794591897295, 5.926030837251451189 ) ) ;
#33706=CARTESIAN_POINT ( 'NONE',  ( 86.43196921298398649, 0.8512835087624049946, 5.909244108978848331 ) ) ;
#33708=CARTESIAN_POINT ( 'NONE',  ( 21.78047190118184773, 5.616103730238553027, 3.473245441588607374 ) ) ;
#33710=CARTESIAN_POINT ( 'NONE',  ( 8.290806648384990041, -10.90558813203967148, -6.000000000000000000 ) ) ;
#33711=CARTESIAN_POINT ( 'NONE',  ( 32.90365724210374765, -3.811969404918499560, 4.977804649287965510 ) ) ;
#33716=EDGE_LOOP ( 'NONE', ( #18762, #26961, #40189, #3953, #1029, #16949 ) ) ;
#33720=CARTESIAN_POINT ( 'NONE',  ( 26.54063429493796278, 1.105409551691596270, 4.373481918376509014 ) ) ;
#33726=ADVANCED_FACE ( 'NONE', ( #26478 ), #39006, .T. ) ;
#33728=DIRECTION ( 'NONE',  ( 1.165409145176969993E-16, -1.000000000000000000, 0.000000000000000000 ) ) ;
#33731=CARTESIAN_POINT ( 'NONE',  ( 24.66025866237015762, 2.990908695463429634, -3.498935737220656872 ) ) ;
#33734=CARTESIAN_POINT ( 'NONE',  ( 23.91855504425362255, 4.211737807167565961, 0.007810489111244203406 ) ) ;
#33738=CARTESIAN_POINT ( 'NONE',  ( 84.25787434187677150, 2.991901652185509075, -1.300773176381055940 ) ) ;
#33746=CARTESIAN_POINT ( 'NONE',  ( 18.22228433872105313, -2.944577058405784875, -3.048495850186285772 ) ) ;
#33747=CARTESIAN_POINT ( 'NONE',  ( 30.51370498771255768, -0.1447642529027365621, -4.968799658713162870 ) ) ;
#33758=ORIENTED_EDGE ( 'NONE', *, *, #34522, .T. ) ;
#33760=CARTESIAN_POINT ( 'NONE',  ( 36.44569688397662333, -1.731580701890905072, 5.730255527505096147 ) ) ;
#33761=CARTESIAN_POINT ( 'NONE',  ( 26.05544091025929276, -2.756875503939111294, 4.272979725902397163 ) ) ;
#33764=CARTESIAN_POINT ( 'NONE',  ( 21.93632313734164185, -3.072674611199754491, -3.536223897022242824 ) ) ;
#33768=CARTESIAN_POINT ( 'NONE',  ( -80.92837670882107659, 2.429809908903242555, -12.50000000000000000 ) ) ;
#33774=CARTESIAN_POINT ( 'NONE',  ( 14.75265942311007983, -4.610020690361468887, 2.508566039384218627 ) ) ;
#33776=CARTESIAN_POINT ( 'NONE',  ( 23.08977137947836056, 2.997041596059222268, 4.148509914069672178 ) ) ;
#33777=CARTESIAN_POINT ( 'NONE',  ( 21.42989180576616803, 8.003656144025150354, -2.742373372379655283 ) ) ;
#33782=CARTESIAN_POINT ( 'NONE',  ( 22.07382372493323786, -2.652280543961057724, -3.651552068356747061 ) ) ;
#33785=CARTESIAN_POINT ( 'NONE',  ( 22.44967802737946272, 3.154736390076984698, -4.439590424646853606 ) ) ;
#33786=CARTESIAN_POINT ( 'NONE',  ( 21.85643539959774273, 10.50077279934518160, -1.805501455388072385 ) ) ;
#33791=CARTESIAN_POINT ( 'NONE',  ( 87.26180097699096905, 0.3411280444268214862, 4.951700522085849876 ) ) ;
#33797=CARTESIAN_POINT ( 'NONE',  ( 15.61919507633180615, -3.751113255642578359, 2.631306685128067091 ) ) ;
#33799=CARTESIAN_POINT ( 'NONE',  ( 35.45425782886216837, -1.912984739101698750, -5.739892417296534433 ) ) ;
#33809=CARTESIAN_POINT ( 'NONE',  ( 23.31574270449137387, 3.489135525515108416, 3.362528818731710167 ) ) ;
#33816=CARTESIAN_POINT ( 'NONE',  ( -73.80328626875311215, 8.420059221808692485, -9.582109240214750301 ) ) ;
#33819=B_SPLINE_SURFACE_WITH_KNOTS ( 'NONE', 5, 3, ( 
 ( #15202, #39911, #12520, #28165, #24677, #21392, #11685, #18282, #12099, #8607, #34379, #36619, #36825, #21599, #15402, #27962, #17867, #34179, #8405, #21185, #6154, #18483, #2257, #2881, #33966, #2474, #40505, #2679, #12315, #5333, #33557, #30451, #24890, #27352, #14997, #27557, #40114, #37022, #8806, #5740, #1004, #19315, #9422, #9844, #19522, #22822, #32297, #18910 ),
 ( #25094, #795, #3497, #6963, #16608, #35392, #396, #16221, #7162, #25496, #22419, #38241, #34586, #38438, #19724, #34989, #37623, #3700, #28587, #4095, #31478, #32102, #25698, #6763, #10243, #31889, #10042, #29192, #28795, #13326, #22011, #6361, #599, #13139, #22622, #35191, #16420, #3908, #3301, #28993, #25902, #15822, #28377, #187, #12724, #25300, #37835, #9638 ),
 ( #22220, #34790, #6566, #31679, #19113, #16020, #12934, #4679, #29989, #17407, #4871, #26310, #23798, #13936, #23609, #23020, #20715, #36173, #33301, #35780, #14329, #29393, #38643, #7359, #7759, #1804, #13538, #23216, #32891, #32488, #10441, #7955, #20503, #5081, #4491, #39442, #17613, #35978, #20306, #17012, #30192, #33087, #8144, #26900, #1599, #16815, #29783, #26507 ),
 ( #17213, #26112, #11232, #36373, #35588, #4288, #11031, #1212, #14130, #26707, #38844, #19917, #13747, #10639, #39241, #7558, #20113, #32692, #29588, #1404, #39037, #10838, #23414, #8352, #33919, #27515, #14730, #2633, #24424, #36980, #11435, #15358, #27102, #8761, #39652, #24840, #37387, #33512, #15153, #27913, #2210, #18643, #21344, #24000, #40067, #37181, #40459, #9181 ),
 ( #27303, #39867, #2011, #36572, #12268, #14949, #5283, #14530, #21753, #11638, #5696, #12049, #17821, #34336, #24628, #30403, #18236, #6107, #36776, #24216, #8558, #27710, #21140, #40264, #11846, #30826, #33706, #8968, #5903, #21555, #34132, #5487, #18029, #30621, #18440, #31029, #2835, #2428, #6916, #31633, #37994, #25650, #25050, #28330, #3857, #25452, #146, #31838 ),
 ( #9379, #7115, #13283, #38392, #25253, #749, #31228, #3049, #22378, #38194, #32051, #22174, #28744, #31433, #34537, #22576, #16176, #37784, #9796, #15776, #9995, #12677, #15569, #19476, #9591, #13089, #22778, #28947, #6522, #34942, #25855, #3457, #28535, #3650, #12480, #16373, #10194, #344, #28122, #6721, #34743, #35345, #37583, #35144, #553, #12888, #21966, #19272 ),
 ( #6311, #18860, #3255, #19069, #15971, #4449, #20464, #29346, #36135, #20072, #26463, #14084, #13489, #16765, #33043, #13897, #1168, #20265, #23169, #35934, #38597, #36331, #1757, #26857, #13698, #29940, #19679, #32252, #10789, #26662, #4833, #10594, #35738, #17365, #39400, #1363, #38991, #7511, #4051, #1553, #14289, #23569, #7715, #22976, #4638, #32648, #11189, #38797 ),
 ( #7915, #39196, #23760, #10400, #17169, #7312, #23366, #29738, #32443, #16566, #29148, #19871, #10990, #954, #26063, #4240, #26265, #16973, #29545, #21507, #5652, #14490, #40023, #33666, #20882, #8718, #30571, #2379, #17568, #34085, #33253, #14900, #5036, #30984, #2788, #27063, #21297, #5860, #8306, #33872, #18396, #33470, #24797, #27468, #30152, #5444, #2585, #15315 ) ),
 .UNSPECIFIED., .F., .T., .F.,
 ( 6, 2, 6 ),
 ( 4, 1, 1, 1, 1, 1, 1, 1, 1, 1, 1, 1, 1, 1, 1, 1, 1, 1, 1, 1, 1, 1, 1, 1, 1, 1, 1, 1, 1, 1, 1, 1, 1, 1, 1, 1, 1, 1, 1, 1, 1, 1, 1, 1, 1, 4 ),
 ( 0.000000000000000000, 0.5000000000000000000, 1.000000000000000000 ),
 ( 0.02319993227479018663, 0.02338707809474536645, 0.02357422391470053238, 0.02376136973465571220, 0.02401089749459594039, 0.02432280719452123083, 0.02469709883443158005, 0.02507139047434192580, 0.02557044599422238565, 0.02619426539407297347, 0.02694284867389366844, 0.02769143195371436342, 0.02844001523353506186, 0.02918859851335575684, 0.02993718179317645181, 0.03068576507299715025, 0.03143434835281785217, 0.03218293163263854367, 0.03293151491245924212, 0.03355533431230981606, 0.03405438983219027937, 0.03442868147210063207, 0.03480297311201098476, 0.03511488281193627520, 0.03536441057187650339, 0.03555155639183167626, 0.03573870221178684914, 0.03598822997172709121, 0.03630013967165238165, 0.03667443131156272740, 0.03704872295147307315, 0.03754777847135353647, 0.03817159787120411735, 0.03892018115102481579, 0.03966876443084551424, 0.04041734771066620574, 0.04141545875042713931, 0.04241356979018806594, 0.04341168082994899952, 0.04416026410976969102, 0.04490884738959038947, 0.04553266678944096341, 0.04603172230932142672, 0.04640601394923177248, 0.04678030558914212517, 0.04715459722905247786 ),
 .UNSPECIFIED. ) ;
#33824=CARTESIAN_POINT ( 'NONE',  ( 23.42497383391232191, 3.742411600671747607, 3.213303063791231207 ) ) ;
#33832=CARTESIAN_POINT ( 'NONE',  ( 23.05082101514768667, 0.3401240180440390226, 5.963255066552523687 ) ) ;
#33833=CARTESIAN_POINT ( 'NONE',  ( 14.74692632493244027, -5.123162004414108850, -2.499999999977825738 ) ) ;
#33839=CARTESIAN_POINT ( 'NONE',  ( 36.77396871613090923, -3.421702227977501565, -5.878726859251444559 ) ) ;
#33844=CARTESIAN_POINT ( 'NONE',  ( 28.07449379822080004, 1.807001228253011016, 3.913063849393144888 ) ) ;
#33848=B_SPLINE_CURVE_WITH_KNOTS ( 'NONE', 3,
 ( #37195, #34555, #31447, #22188, #3269, #8985, #28345, #21361 ),
 .UNSPECIFIED., .F., .F.,
 ( 4, 2, 2, 4 ),
 ( 0.000000000000000000, 0.0004377122104129928964, 0.0006565683156194867696, 0.0008754244208259806970 ),
 .UNSPECIFIED. ) ;
#33850=EDGE_CURVE ( 'NONE', #16288, #25100, #9837, .T. ) ;
#33854=CARTESIAN_POINT ( 'NONE',  ( 37.15950049230122687, -2.950588481368993321, -5.999614729618140352 ) ) ;
#33863=CARTESIAN_POINT ( 'NONE',  ( 24.87654660328950129, 1.883990792660638069, -4.293584299149880934 ) ) ;
#33865=ORIENTED_EDGE ( 'NONE', *, *, #36733, .T. ) ;
#33867=DIRECTION ( 'NONE',  ( 1.165409145176969993E-16, -1.000000000000000000, 0.000000000000000000 ) ) ;
#33872=CARTESIAN_POINT ( 'NONE',  ( 87.82658540711466344, -2.392274210255118216, -1.851534029869310816 ) ) ;
#33873=EDGE_CURVE ( 'NONE', #34747, #37237, #28476, .T. ) ;
#33879=SHAPE_DEFINITION_REPRESENTATION ( #17689, #131 ) ;
#33882=CARTESIAN_POINT ( 'NONE',  ( 23.14331707321704457, 4.052454345113581269, 3.066645182171226836 ) ) ;
#33890=AXIS2_PLACEMENT_3D ( 'NONE', #17880, #33367, #30253 ) ;
#33891=CARTESIAN_POINT ( 'NONE',  ( 22.01622206693788897, 4.835086392017111656, 3.641232820207879417 ) ) ;
#33895=CARTESIAN_POINT ( 'NONE',  ( 22.56491764776242803, -2.112007571549842755, -8.936849366082922685 ) ) ;
#33901=CARTESIAN_POINT ( 'NONE',  ( -78.34784942564689914, 10.09360306622668446, -8.412543785568951549 ) ) ;
#33902=CARTESIAN_POINT ( 'NONE',  ( 1.700390093233090871, -29.56993018339339940, -2.499999999999998668 ) ) ;
#33903=CARTESIAN_POINT ( 'NONE',  ( 36.88828627238819280, -3.352251944545559414, -5.910322522570560899 ) ) ;
#33905=CARTESIAN_POINT ( 'NONE',  ( 15.30733144061336581, 11.48784145168144732, 2.585939450232884962 ) ) ;
#33908=CARTESIAN_POINT ( 'NONE',  ( 17.85923178500418373, 13.84674244481094085, -2.499999999999999556 ) ) ;
#33909=LINE ( 'NONE', #22163, #25385 ) ;
#33910=CARTESIAN_POINT ( 'NONE',  ( 24.42208616128406362, 2.821435771912959023, -3.829602786363869971 ) ) ;
#33913=CARTESIAN_POINT ( 'NONE',  ( 31.78478551401448016, -0.3652337162497744649, 5.167182516041234130 ) ) ;
#33919=CARTESIAN_POINT ( 'NONE',  ( 86.17769677085827595, 1.483769024673816661, 5.380928644057212828 ) ) ;
#33921=LINE ( 'NONE', #27304, #40593 ) ;
#33925=ORIENTED_EDGE ( 'NONE', *, *, #28157, .F. ) ;
#33926=LINE ( 'NONE', #5700, #1163 ) ;
#33940=CARTESIAN_POINT ( 'NONE',  ( -17.69482985384421880, -29.56993018339339940, 6.000000000000000000 ) ) ;
#33941=CARTESIAN_POINT ( 'NONE',  ( -17.27251170661583402, 3.729367930467589076, 6.000000000000000000 ) ) ;
#33942=CARTESIAN_POINT ( 'NONE',  ( 14.77222811005485603, -4.461988841550141416, 2.511961482897715481 ) ) ;
#33944=CARTESIAN_POINT ( 'NONE',  ( 24.32052479808152157, 3.131090298592408949, -3.427421788660176105 ) ) ;
#33948=CARTESIAN_POINT ( 'NONE',  ( 23.94338804316802438, 3.829326634665836782, 2.990621344434266415 ) ) ;
#33953=CARTESIAN_POINT ( 'NONE',  ( 85.30740962031771346, 1.871039318281703334, 5.038373847784950676 ) ) ;
#33960=CARTESIAN_POINT ( 'NONE',  ( 31.37632533542383229, -3.544562347629171661, -4.958508136961243373 ) ) ;
#33961=CARTESIAN_POINT ( 'NONE',  ( 27.40457795791207829, 0.9565065509615210404, -4.483545191191414148 ) ) ;
#33962=CARTESIAN_POINT ( 'NONE',  ( 11.29080664838498649, 1.564594260697056104E-15, 2.500000000000000000 ) ) ;
#33964=EDGE_LOOP ( 'NONE', ( #2269, #16227, #950, #34080, #2476, #9038, #4526, #13574 ) ) ;
#33966=CARTESIAN_POINT ( 'NONE',  ( 86.40868413783579172, 1.299389369533768379, 4.865112849554557251 ) ) ;
#33968=ORIENTED_EDGE ( 'NONE', *, *, #4732, .T. ) ;
#33971=CARTESIAN_POINT ( 'NONE',  ( 35.83279683802916082, -3.732019870312798027, 5.621828468275774426 ) ) ;
#33973=CARTESIAN_POINT ( 'NONE',  ( 22.05244047626662862, -2.652259403379859215, 3.648214695246499772 ) ) ;
#33983=CARTESIAN_POINT ( 'NONE',  ( 14.77209256136291238, -5.161470997039804054, 2.500001702421898564 ) ) ;
#33985=CARTESIAN_POINT ( 'NONE',  ( 21.85013245281674799, 2.795871195627560368, 5.288339663639888499 ) ) ;
#33986=CARTESIAN_POINT ( 'NONE',  ( 31.35344415347196545, 0.5184038160239171633, 4.590894038415813228 ) ) ;
#33996=CARTESIAN_POINT ( 'NONE',  ( 23.68553352910465648, 3.075504613652856989, -3.816384475219152694 ) ) ;
#33999=CARTESIAN_POINT ( 'NONE',  ( 21.85643539959779957, 4.362886173974390935, 14.46802226367788791 ) ) ;
#34000=CARTESIAN_POINT ( 'NONE',  ( -62.92837670882109080, -52.49535338866469658, 6.000000000000000000 ) ) ;
#34002=CARTESIAN_POINT ( 'NONE',  ( -4.890026461918814071, -8.228598103685714525E-16, 6.000000000000000000 ) ) ;
#34005=CARTESIAN_POINT ( 'NONE',  ( 88.39837738899358044, -0.9355285267052176890, 2.786041992172542336 ) ) ;
#34010=CARTESIAN_POINT ( 'NONE',  ( 14.89216304183951678, -6.126272768353560494, 2.529875904917741725 ) ) ;
#34012=CARTESIAN_POINT ( 'NONE',  ( 31.72030731019543381, -0.5546557356656219850, -5.157119132924021798 ) ) ;
#34023=CARTESIAN_POINT ( 'NONE',  ( 36.82361487772457309, -2.161144939959093403, 5.895778257769980435 ) ) ;
#34030=CARTESIAN_POINT ( 'NONE',  ( -76.57843430598849466, -5.832456142219742290, -8.260218182170147472 ) ) ;
#34035=ORIENTED_EDGE ( 'NONE', *, *, #34324, .F. ) ;
#34036=CARTESIAN_POINT ( 'NONE',  ( 22.00772085900330666, 5.524290953573272489, 3.138816991787310773 ) ) ;
#34038=ADVANCED_FACE ( 'NONE', ( #17794 ), #17380, .F. ) ;
#34043=CARTESIAN_POINT ( 'NONE',  ( -72.35143257368834213, -46.63264610307073355, 5.828929736913487147 ) ) ;
#34046=VECTOR ( 'NONE', #18240, 1000.000000000000000 ) ;
#34052=DIRECTION ( 'NONE',  ( -1.000000000000000000, 0.000000000000000000, 0.000000000000000000 ) ) ;
#34057=CARTESIAN_POINT ( 'NONE',  ( 31.05604276399450114, -2.500009215535430762, 5.784057531382419626 ) ) ;
#34061=CARTESIAN_POINT ( 'NONE',  ( 22.31500143320247531, 0.2710179362157456029, -7.066509127937782075 ) ) ;
#34063=DIRECTION ( 'NONE',  ( 1.000000000000000000, 0.000000000000000000, 0.000000000000000000 ) ) ;
#34067=CARTESIAN_POINT ( 'NONE',  ( 34.57554517587881548, -0.8971683385966218172, -5.398457213048259540 ) ) ;
#34071=CARTESIAN_POINT ( 'NONE',  ( 8.290806648384990041, -25.50263309590217276, -2.499999999999998668 ) ) ;
#34073=CARTESIAN_POINT ( 'NONE',  ( -73.47413635169593249, 5.573843681890572554, 10.88137847971116123 ) ) ;
#34074=EDGE_CURVE ( 'NONE', #26564, #30447, #25982, .T. ) ;
#34077=CARTESIAN_POINT ( 'NONE',  ( 14.74026921260515088, -4.699362955988203083, -2.506077451199989703 ) ) ;
#34078=CARTESIAN_POINT ( 'NONE',  ( 23.26251525840845957, 2.275869519923719331, -4.593821674871367833 ) ) ;
#34080=ORIENTED_EDGE ( 'NONE', *, *, #19261, .T. ) ;
#34085=CARTESIAN_POINT ( 'NONE',  ( 86.62140889132389532, -0.8164050916001737157, 5.580443680875508683 ) ) ;
#34091=CARTESIAN_POINT ( 'NONE',  ( 21.70978835544913110, 6.347857807235328664, 3.186345948389122551 ) ) ;
#34094=ORIENTED_EDGE ( 'NONE', *, *, #16842, .F. ) ;
#34097=CARTESIAN_POINT ( 'NONE',  ( 17.47038219521028779, 11.99840016206135118, -2.499999999999995115 ) ) ;
#34103=ADVANCED_FACE ( 'NONE', ( #15329 ), #40238, .T. ) ;
#34105=CARTESIAN_POINT ( 'NONE',  ( 22.71767909661236118, -4.608197067329504293, -7.212190040765698917 ) ) ;
#34107=CARTESIAN_POINT ( 'NONE',  ( -72.90053700259019820, 3.429967363124852842, 10.95643088971294965 ) ) ;
#34108=CARTESIAN_POINT ( 'NONE',  ( 37.19556178435423277, -2.859567876585734414, 6.000000005145950333 ) ) ;
#34113=CARTESIAN_POINT ( 'NONE',  ( -80.35180597995123719, 11.50364652777614971, -3.371254867381904496 ) ) ;
#34115=CARTESIAN_POINT ( 'NONE',  ( 37.00845883712383966, -3.246107522403217427, -5.947038319129071660 ) ) ;
#34117=CARTESIAN_POINT ( 'NONE',  ( 14.71143272272386326, 12.53673232395533965, 2.502472892362715307 ) ) ;
#34119=CARTESIAN_POINT ( 'NONE',  ( 29.51619774652193229, -3.826605600177332089, 4.386877048897818376 ) ) ;
#34125=CARTESIAN_POINT ( 'NONE',  ( 24.55513722008589639, 2.975329870594148218, -3.595293232472362988 ) ) ;
#34129=CARTESIAN_POINT ( 'NONE',  ( 35.33527427362074746, -3.300844520036612995, 5.721322155873344251 ) ) ;
#34131=LINE ( 'NONE', #6720, #35887 ) ;
#34132=CARTESIAN_POINT ( 'NONE',  ( 87.57592060778061693, -0.6244806207018304134, 5.359096402341661403 ) ) ;
#34134=CARTESIAN_POINT ( 'NONE',  ( -71.92837670882107659, -23.80776546975053520, 9.949874371066204759 ) ) ;
#34137=CARTESIAN_POINT ( 'NONE',  ( 24.63732103174290700, 2.685245520235881589, 3.901802067749889691 ) ) ;
#34138=B_SPLINE_CURVE_WITH_KNOTS ( 'NONE', 3,
 ( #11785, #27457, #33657, #30145, #23948, #2369, #34073, #5848, #14888, #24366, #2778, #36929, #27856, #8708, #25188, #10131, #37528, #6662, #6862, #34888, #28475, #31988, #25394, #19214, #25797, #37933, #35086, #22718, #13231, #9742, #22319, #31778 ),
 .UNSPECIFIED., .F., .F.,
 ( 4, 2, 2, 2, 2, 2, 2, 2, 2, 2, 2, 2, 2, 2, 2, 4 ),
 ( 0.06009542766246023932, 0.06130746216911493740, 0.06251949667576962855, 0.06373153118242433357, 0.06494356568907902472, 0.06615560019573371586, 0.06676161744906104756, 0.06736763470238837925, 0.06857966920904304264, 0.06918568646237036046, 0.06979170371569767828, 0.07221577272900697730, 0.07463984174231627633, 0.07585187624897093972, 0.07706391075562560311, 0.07948797976893491601 ),
 .UNSPECIFIED. ) ;
#34139=CARTESIAN_POINT ( 'NONE',  ( -62.92837670882106238, -23.80776546975053520, -6.000000000000000000 ) ) ;
#34143=UNCERTAINTY_MEASURE_WITH_UNIT (LENGTH_MEASURE( 1.000000000000000082E-05 ), #37895, 'distance_accuracy_value', 'NONE');
#34145=ORIENTED_EDGE ( 'NONE', *, *, #13562, .T. ) ;
#34157=CARTESIAN_POINT ( 'NONE',  ( 21.88600830960537635, 5.632864204250798146, -3.275930472131208138 ) ) ;
#34162=CARTESIAN_POINT ( 'NONE',  ( 25.28494853283190125, -3.333630280469910723, 5.108382079771137008 ) ) ;
#34164=CARTESIAN_POINT ( 'NONE',  ( -77.39670385617056070, -6.181659773469543318, -7.628895083485716988 ) ) ;
#34167=CARTESIAN_POINT ( 'NONE',  ( 88.38642666631945133, -2.374919807968325358, 0.2172961577596721761 ) ) ;
#34177=CARTESIAN_POINT ( 'NONE',  ( 35.78607896117043197, -3.162280031239083744, 5.791681130117677156 ) ) ;
#34179=CARTESIAN_POINT ( 'NONE',  ( 85.24855023725586989, 2.602506829941634514, 1.762177041774413588 ) ) ;
#34194=CARTESIAN_POINT ( 'NONE',  ( 21.85329537605191419, 3.009163427712417960, 5.104443796496481944 ) ) ;
#34195=CARTESIAN_POINT ( 'NONE',  ( 14.73500979046644233, 12.83520685450635490, 2.502377855999189826 ) ) ;
#34197=AXIS2_PLACEMENT_3D ( 'NONE', #10282, #26150, #37523 ) ;
#34206=CARTESIAN_POINT ( 'NONE',  ( 23.48457729831129726, 3.066923110525566543, -3.897436638742564963 ) ) ;
#34208=CARTESIAN_POINT ( 'NONE',  ( 21.85643539959776760, -0.9922589305345951294, -16.01828770219436393 ) ) ;
#34214=CARTESIAN_POINT ( 'NONE',  ( 87.87162303905448368, -0.3438530395839958231, 3.959040383187740542 ) ) ;
#34216=CARTESIAN_POINT ( 'NONE',  ( -62.14171895907916365, -49.48408358960642062, -4.951123000344130887 ) ) ;
#34219=CARTESIAN_POINT ( 'NONE',  ( 15.11041258174173407, -4.075176119877783165, 2.561837290471254303 ) ) ;
#34220=CARTESIAN_POINT ( 'NONE',  ( 24.75830837035764276, 3.019210359990082804, 3.350572556515618583 ) ) ;
#34221=CARTESIAN_POINT ( 'NONE',  ( 36.63352589858980224, -3.080950350379837666, -5.923945720283577465 ) ) ;
#34228=ORIENTED_EDGE ( 'NONE', *, *, #117, .F. ) ;
#34229=CARTESIAN_POINT ( 'NONE',  ( 37.08862871230790148, -2.428037328474826229, 5.958176329106160019 ) ) ;
#34242=CARTESIAN_POINT ( 'NONE',  ( 22.00379729694733655, 5.541703127858326638, 3.130312335064352247 ) ) ;
#34255=ORIENTED_EDGE ( 'NONE', *, *, #28267, .F. ) ;
#34263=CARTESIAN_POINT ( 'NONE',  ( 29.24680661740138632, 2.095232292622827508, -1.948189103474716966 ) ) ;
#34267=CARTESIAN_POINT ( 'NONE',  ( 23.60029590725254778, 0.4360417540011212734, -5.514987849079120430 ) ) ;
#34269=VERTEX_POINT ( 'NONE', #23492 ) ;
#34275=CARTESIAN_POINT ( 'NONE',  ( 36.18514542968358683, -3.553240791427502820, -5.771079380064234599 ) ) ;
#34277=DIRECTION ( 'NONE',  ( -0.000000000000000000, -1.000000000000000000, -0.000000000000000000 ) ) ;
#34278=CARTESIAN_POINT ( 'NONE',  ( -17.27251170661583402, 0.7293679304675921848, 6.000000000000000000 ) ) ;
#34280=CARTESIAN_POINT ( 'NONE',  ( -77.92837670882107659, 2.429809908903242555, 12.50000000000000000 ) ) ;
#34284=CARTESIAN_POINT ( 'NONE',  ( 14.73982985784992117, -5.057483637003035604, -2.500280250512573854 ) ) ;
#34286=ORIENTED_EDGE ( 'NONE', *, *, #11831, .F. ) ;
#34287=DIRECTION ( 'NONE',  ( 1.000000000000000000, 0.000000000000000000, 0.000000000000000000 ) ) ;
#34290=VERTEX_POINT ( 'NONE', #1282 ) ;
#34300=CARTESIAN_POINT ( 'NONE',  ( 23.75888155827460579, 3.577044823368265458, 3.132426108058699477 ) ) ;
#34310=CARTESIAN_POINT ( 'NONE',  ( 21.85643539959776049, -10.96491163060450802, -3.419414754301954851 ) ) ;
#34312=ORIENTED_EDGE ( 'NONE', *, *, #16956, .F. ) ;
#34313=CARTESIAN_POINT ( 'NONE',  ( -75.92086343153737005, 8.774164695908069689, 10.09508035950012506 ) ) ;
#34317=CARTESIAN_POINT ( 'NONE',  ( 28.62670612262708758, -3.097740522901847093, -4.674287848576377691 ) ) ;
#34318=CARTESIAN_POINT ( 'NONE',  ( 33.94692901654968153, -0.4865178363018504704, -5.119572993145925288 ) ) ;
#34320=FACE_OUTER_BOUND ( 'NONE', #40544, .T. ) ;
#34324=EDGE_CURVE ( 'NONE', #16788, #7910, #17089, .T. ) ;
#34325=CARTESIAN_POINT ( 'NONE',  ( 17.55394540761496813, 14.11332787939523215, -2.499999999999998668 ) ) ;
#34326=CARTESIAN_POINT ( 'NONE',  ( 24.71293417245692225, 0.6467480212540300810, -4.786583799029410002 ) ) ;
#34328=CARTESIAN_POINT ( 'NONE',  ( 37.19703447091560378, -2.679050652368330621, -5.993601543857010938 ) ) ;
#34329=CARTESIAN_POINT ( 'NONE',  ( 24.39286117734144810, 2.948013837470140786, -3.707038986443544015 ) ) ;
#34332=CARTESIAN_POINT ( 'NONE',  ( 37.09997507242855619, -2.920746538320391217, 5.996328951322015932 ) ) ;
#34336=CARTESIAN_POINT ( 'NONE',  ( 84.61987491094994596, 3.070148169510762415, -1.277140785624046426 ) ) ;
#34337=EDGE_CURVE ( 'NONE', #35445, #36906, #15231, .T. ) ;
#34338=CARTESIAN_POINT ( 'NONE',  ( 25.01075926162736351, 3.329891198200423563, 1.935509954479121886 ) ) ;
#34341=CARTESIAN_POINT ( 'NONE',  ( 24.69446985135231643, 2.652829802148882532, 3.917487620480931465 ) ) ;
#34358=CARTESIAN_POINT ( 'NONE',  ( 14.72123706662754117, -4.461849342347327330, 2.504003097347841766 ) ) ;
#34359=CARTESIAN_POINT ( 'NONE',  ( 21.85047837349528876, 5.846451070568255304, -3.185295450005349416 ) ) ;
#34360=ORIENTED_EDGE ( 'NONE', *, *, #21905, .F. ) ;
#34363=CARTESIAN_POINT ( 'NONE',  ( 24.13449073166137637, 1.731319574254092997, -6.231442870084249464 ) ) ;
#34364=CARTESIAN_POINT ( 'NONE',  ( -79.05013602958881336, -6.599521673326993465, -5.889945335535864857 ) ) ;
#34367=CARTESIAN_POINT ( 'NONE',  ( 85.07031394220433640, 1.982162274098862476, -4.809620659748507165 ) ) ;
#34373=CYLINDRICAL_SURFACE ( 'NONE', #26522, 1.000000000000000444 ) ;
#34377=CARTESIAN_POINT ( 'NONE',  ( 36.19384301497849776, -2.232512094164133210, 5.855322572525271774 ) ) ;
#34379=CARTESIAN_POINT ( 'NONE',  ( 85.56690561042726983, 2.244914964738076613, -3.295588454431229497 ) ) ;
#34383=CARTESIAN_POINT ( 'NONE',  ( 16.46868226795076140, -3.215900133094863111, 2.776734183136223777 ) ) ;
#34398=CARTESIAN_POINT ( 'NONE',  ( 23.42816911322859852, 2.562534313632369276, 4.299399775110970268 ) ) ;
#34399=DIRECTION ( 'NONE',  ( 0.000000000000000000, -0.000000000000000000, -1.000000000000000000 ) ) ;
#34404=CARTESIAN_POINT ( 'NONE',  ( 86.46381120609095206, 1.237468029981063866, -4.897693362183704657 ) ) ;
#34408=CARTESIAN_POINT ( 'NONE',  ( 22.61679165579552020, 3.482051183000346661, -4.061253451716217988 ) ) ;
#34409=ORIENTED_EDGE ( 'NONE', *, *, #18569, .T. ) ;
#34410=CARTESIAN_POINT ( 'NONE',  ( 21.85643539959776049, -15.24219007203948983, -1.854490019360333086 ) ) ;
#34415=CARTESIAN_POINT ( 'NONE',  ( 85.81943862418182789, 1.961257897749014045, -4.406084401447566634 ) ) ;
#34420=CARTESIAN_POINT ( 'NONE',  ( 33.10591517636001413, -3.525528538284762980, 5.308841012747972599 ) ) ;
#34422=CARTESIAN_POINT ( 'NONE',  ( 35.45475390766367951, -1.911721085124097108, -5.739969842391221100 ) ) ;
#34427=CARTESIAN_POINT ( 'NONE',  ( 33.94443037723285528, -0.4909204995510449976, 5.125095304665048701 ) ) ;
#34430=CARTESIAN_POINT ( 'NONE',  ( 87.67362551673814153, -2.207058729090509264, -2.772829007886140396 ) ) ;
#34431=ORIENTED_EDGE ( 'NONE', *, *, #25680, .T. ) ;
#34433=CARTESIAN_POINT ( 'NONE',  ( -73.59999746138505827, -3.294935041615913107, -9.639447355971549669 ) ) ;
#34440=CARTESIAN_POINT ( 'NONE',  ( 22.62113927429973970, 4.590997775111404167, 3.081078265741201694 ) ) ;
#34447=CARTESIAN_POINT ( 'NONE',  ( 14.76059668380545808, 12.79626003940931334, -2.505178952959561833 ) ) ;
#34449=CARTESIAN_POINT ( 'NONE',  ( 37.19747299874393320, -2.841585884120807481, 5.999818732555961098 ) ) ;
#34450=CARTESIAN_POINT ( 'NONE',  ( 18.49040214524046277, 7.936735459317859842, -3.063322579770844545 ) ) ;
#34461=CARTESIAN_POINT ( 'NONE',  ( 28.29523375420085074, 1.184784106264966219, 4.843441543353563361 ) ) ;
#34466=CARTESIAN_POINT ( 'NONE',  ( 25.38078854466783696, 0.7236405097827043331, -4.601989520496759134 ) ) ;
#34470=CARTESIAN_POINT ( 'NONE',  ( 33.45716606812183613, -3.829385970599605393, -5.093809925484540813 ) ) ;
#34471=CARTESIAN_POINT ( 'NONE',  ( 36.86628255965130307, -3.288546807751189238, -5.928673330178329870 ) ) ;
#34473=CARTESIAN_POINT ( 'NONE',  ( 31.04874620950890218, -3.764186376626990072, 4.612088004693758236 ) ) ;
#34479=CARTESIAN_POINT ( 'NONE',  ( 22.03385624869050829, -11.53008493239669718, 2.499999999999999556 ) ) ;
#34487=CARTESIAN_POINT ( 'NONE',  ( 11.29080664838499182, -35.94265729135299381, -2.500000000000000000 ) ) ;
#34494=CARTESIAN_POINT ( 'NONE',  ( 23.76174458026235925, 3.579459537482711173, 3.123613177595400359 ) ) ;
#34496=AXIS2_PLACEMENT_3D ( 'NONE', #20511, #40269, #36580 ) ;
#34499=CARTESIAN_POINT ( 'NONE',  ( 25.84749379405300829, 0.9947621561361583709, 4.433988674360729298 ) ) ;
#34507=CARTESIAN_POINT ( 'NONE',  ( 22.31758782591801094, 6.227955964823622459, -0.6941013191108784675 ) ) ;
#34510=CARTESIAN_POINT ( 'NONE',  ( -72.92764087594211730, 1.045607383799636914, 10.95381248315954892 ) ) ;
#34511=CARTESIAN_POINT ( 'NONE',  ( 34.98542202245123178, -3.831422351504832235, 5.422976750267761048 ) ) ;
#34517=CARTESIAN_POINT ( 'NONE',  ( 33.45672436422175622, -3.834025908535790617, -5.088635116787304291 ) ) ;
#34519=CARTESIAN_POINT ( 'NONE',  ( 18.57920759633674379, 8.033290316770353101, 3.021679359481073579 ) ) ;
#34520=DIRECTION ( 'NONE',  ( 0.000000000000000000, -0.000000000000000000, -1.000000000000000000 ) ) ;
#34522=EDGE_CURVE ( 'NONE', #11084, #21833, #29878, .T. ) ;
#34524=CARTESIAN_POINT ( 'NONE',  ( -71.92837670882107659, -20.78299143688747819, 38.00000000000000711 ) ) ;
#34528=CARTESIAN_POINT ( 'NONE',  ( 22.41226710412750123, 0.3842729703838025923, -6.836439051281914203 ) ) ;
#34530=CARTESIAN_POINT ( 'NONE',  ( 24.38031847485193992, 2.859899372990460265, -3.804262765778354094 ) ) ;
#34534=CARTESIAN_POINT ( 'NONE',  ( 37.02901651221678492, -3.025130311963915464, 5.984744259697210467 ) ) ;
#34537=CARTESIAN_POINT ( 'NONE',  ( 84.32156544206206661, 3.079100735703119707, -0.4907544566128131391 ) ) ;
#34539=CARTESIAN_POINT ( 'NONE',  ( 34.93825735751887152, -3.179062036616587150, -5.659358064224856655 ) ) ;
#34541=CARTESIAN_POINT ( 'NONE',  ( 26.28029581147721316, 1.816827303229512358, 4.266281445978443720 ) ) ;
#34543=DIRECTION ( 'NONE',  ( 1.000000000000000000, 0.000000000000000000, 0.000000000000000000 ) ) ;
#34555=CARTESIAN_POINT ( 'NONE',  ( 14.61802081865033820, 12.48098255133615453, 2.500000000000000000 ) ) ;
#34557=VERTEX_POINT ( 'NONE', #7786 ) ;
#34559=ADVANCED_FACE ( 'NONE', ( #13565 ), #4318, .T. ) ;
#34561=CARTESIAN_POINT ( 'NONE',  ( 24.86588413226784766, -5.834012684512337898, 2.864494517088915337 ) ) ;
#34562=DIRECTION ( 'NONE',  ( -1.000000000000000000, 0.000000000000000000, 0.000000000000000000 ) ) ;
#34564=CARTESIAN_POINT ( 'NONE',  ( 23.73594193330650626, 3.550460969293395941, -3.216120006333157644 ) ) ;
#34568=CARTESIAN_POINT ( 'NONE',  ( 25.45397947482645762, -4.047761836529544688, -3.708248611797466232 ) ) ;
#34570=CARTESIAN_POINT ( 'NONE',  ( -78.55304626648006661, -6.529379806983721224, -6.520005268348637806 ) ) ;
#34573=CARTESIAN_POINT ( 'NONE',  ( 88.08925887309592895, -2.022426073114577338, 2.982665067064442788 ) ) ;
#34583=CARTESIAN_POINT ( 'NONE',  ( 36.78893668764049352, -3.040219878132970344, 5.948201332539075459 ) ) ;
#34586=CARTESIAN_POINT ( 'NONE',  ( 85.19528866922426857, 2.662332751101227579, -1.941753459690362726 ) ) ;
#34589=CARTESIAN_POINT ( 'NONE',  ( 14.75451844360372178, -5.147523147571517299, 2.499999999999998668 ) ) ;
#34591=CARTESIAN_POINT ( 'NONE',  ( 14.72179218383689481, 13.26053291077059626, -2.500109524128790728 ) ) ;
#34593=CARTESIAN_POINT ( 'NONE',  ( 25.13734313143301335, -5.618766742075456122, -2.946603579881577062 ) ) ;
#34594=ORIENTED_EDGE ( 'NONE', *, *, #11414, .F. ) ;
#34595=CARTESIAN_POINT ( 'NONE',  ( 8.290806648384990041, 0.000000000000000000, 2.500000000000000000 ) ) ;
#34600=CARTESIAN_POINT ( 'NONE',  ( 22.67068927409770041, 2.950683925037858035, 4.428361241734660503 ) ) ;
#34601=CARTESIAN_POINT ( 'NONE',  ( 14.77315594796471743, 13.19392823276620419, 2.499999999999996891 ) ) ;
#34609=CARTESIAN_POINT ( 'NONE',  ( 85.73004710101714920, 2.061666699345307663, -3.754548065942108881 ) ) ;
#34613=CARTESIAN_POINT ( 'NONE',  ( 22.59525629365376886, 3.701236930939566072, -3.909849338992366974 ) ) ;
#34617=CARTESIAN_POINT ( 'NONE',  ( 21.85643539959776049, -14.86125632165375343, -4.251346793879176467 ) ) ;
#34623=CARTESIAN_POINT ( 'NONE',  ( 85.38025200535193449, 2.454573153073208225, 3.240196491381199362 ) ) ;
#34625=EDGE_CURVE ( 'NONE', #7910, #12163, #6748, .T. ) ;
#34627=CARTESIAN_POINT ( 'NONE',  ( 15.08693209430224691, -4.053257314178727810, 2.560592534577949220 ) ) ;
#34628=EDGE_CURVE ( 'NONE', #11656, #21561, #11275, .T. ) ;
#34629=CARTESIAN_POINT ( 'NONE',  ( 27.40697018688743825, 0.9632752721768236270, -4.483918556379298259 ) ) ;
#34636=CARTESIAN_POINT ( 'NONE',  ( 36.68389848233819350, -1.917438981616092386, 5.804549737457618264 ) ) ;
#34642=CARTESIAN_POINT ( 'NONE',  ( 88.13248502410320384, -0.6368656024474566024, -2.456193918704937751 ) ) ;
#34643=CARTESIAN_POINT ( 'NONE',  ( -72.93001361936202898, -2.241696845072889133, -9.799423676346561862 ) ) ;
#34646=DIRECTION ( 'NONE',  ( -0.000000000000000000, -0.000000000000000000, -1.000000000000000000 ) ) ;
#34658=CARTESIAN_POINT ( 'NONE',  ( -72.41848181666769335, -46.91894873934776200, 5.812054902733909678 ) ) ;
#34660=CARTESIAN_POINT ( 'NONE',  ( 17.26911231124185520, 8.751764850756153180, -2.901660649865550390 ) ) ;
#34670=CARTESIAN_POINT ( 'NONE',  ( 28.96592479936138176, -0.01829609152130128036, -5.755841479376210934 ) ) ;
#34680=EDGE_CURVE ( 'NONE', #27368, #7, #9940, .T. ) ;
#34682=CARTESIAN_POINT ( 'NONE',  ( 35.19026967813762496, -1.105067851863670958, -5.467017298376940282 ) ) ;
#34683=FACE_OUTER_BOUND ( 'NONE', #39929, .T. ) ;
#34685=CARTESIAN_POINT ( 'NONE',  ( 26.27415342575414314, -2.868604062501628693, -4.307115103527353384 ) ) ;
#34690=DIRECTION ( 'NONE',  ( 1.000000000000000000, 0.000000000000000000, 0.000000000000000000 ) ) ;
#34692=CARTESIAN_POINT ( 'NONE',  ( -70.92837670882107659, -42.37473357531882812, 0.000000000000000000 ) ) ;
#34695=ORIENTED_EDGE ( 'NONE', *, *, #624, .T. ) ;
#34698=CARTESIAN_POINT ( 'NONE',  ( 23.50817669065435922, 2.991962955900060450, 3.946939482339846705 ) ) ;
#34703=CARTESIAN_POINT ( 'NONE',  ( 24.77118930371659999, 3.025291850199358201, 3.323350240946416179 ) ) ;
#34710=CARTESIAN_POINT ( 'NONE',  ( 22.34894292866030696, 0.2931249150505332302, 6.995814783045894103 ) ) ;
#34716=CARTESIAN_POINT ( 'NONE',  ( 22.33830324658017830, 5.012815666754769417, -5.469126444728273029 ) ) ;
#34717=CARTESIAN_POINT ( 'NONE',  ( 21.85643539959777115, -15.24623503193425123, 0.9260495571226281530 ) ) ;
#34719=CARTESIAN_POINT ( 'NONE',  ( -76.82502513205872674, 9.399367495309471465, 9.598227121387571614 ) ) ;
#34725=CARTESIAN_POINT ( 'NONE',  ( 29.47129117146416633, -2.981296461931936204, -4.806105771814197958 ) ) ;
#34726=CARTESIAN_POINT ( 'NONE',  ( 37.21234802891099491, -2.743797681025498481, -6.000906795383097680 ) ) ;
#34728=CARTESIAN_POINT ( 'NONE',  ( 20.71699657508508707, 6.166998326322726598, 3.398385492444088385 ) ) ;
#34735=CARTESIAN_POINT ( 'NONE',  ( 22.83184364098003627, 0.9670597066702968370, -5.845920663466038114 ) ) ;
#34736=DIRECTION ( 'NONE',  ( 7.826543628040252284E-17, -1.000000000000000000, 0.000000000000000000 ) ) ;
#34739=ORIENTED_EDGE ( 'NONE', *, *, #7348, .F. ) ;
#34741=CARTESIAN_POINT ( 'NONE',  ( 34.98297737265904317, -1.566505368433440015, 5.666337704145168352 ) ) ;
#34743=CARTESIAN_POINT ( 'NONE',  ( 88.12503612275229159, -2.065192647045405838, -2.806263388478303256 ) ) ;
#34744=CARTESIAN_POINT ( 'NONE',  ( 25.06963540266364632, 3.214953575097277749, 2.439413512043087984 ) ) ;
#34747=VERTEX_POINT ( 'NONE', #3597 ) ;
#34748=CARTESIAN_POINT ( 'NONE',  ( 24.44576246782188278, 2.805470990093293704, 3.838296511438501923 ) ) ;
#34749=EDGE_CURVE ( 'NONE', #13546, #561, #35801, .T. ) ;
#34751=CARTESIAN_POINT ( 'NONE',  ( -12.99139449055068596, 10.37661300689600097, 6.000000000000000000 ) ) ;
#34755=AXIS2_PLACEMENT_3D ( 'NONE', #9822, #15384, #27941 ) ;
#34758=ADVANCED_FACE ( 'NONE', ( #893 ), #26006, .F. ) ;
#34767=CARTESIAN_POINT ( 'NONE',  ( -71.72859902172312729, -21.39704238849792262, 9.968370014334123397 ) ) ;
#34772=CARTESIAN_POINT ( 'NONE',  ( -80.20775046477413639, -6.649906843095007680, -3.749433596971158078 ) ) ;
#34776=CARTESIAN_POINT ( 'NONE',  ( 87.32189673294487875, -1.771757446153727322, -4.160567758657673920 ) ) ;
#34778=CARTESIAN_POINT ( 'NONE',  ( 1.700390093233090871, -29.56993018339339940, 6.000000000000001776 ) ) ;
#34782=CARTESIAN_POINT ( 'NONE',  ( 22.07327628326154922, 4.461839481733763435, -0.3963575452862883597 ) ) ;
#34785=CARTESIAN_POINT ( 'NONE',  ( 15.30049896279744992, -3.947521880118775250, -2.581831727127946063 ) ) ;
#34788=CARTESIAN_POINT ( 'NONE',  ( 34.13633707975591136, -3.132998035770167888, 5.534199010363774818 ) ) ;
#34790=CARTESIAN_POINT ( 'NONE',  ( 87.10491796770416784, 0.5173464865745804886, -5.275911943831619766 ) ) ;
#34798=CARTESIAN_POINT ( 'NONE',  ( -80.93405938708093572, -6.594533268907218471, 0.2501301618973993945 ) ) ;
#34799=ORIENTED_EDGE ( 'NONE', *, *, #25735, .F. ) ;
#34805=CARTESIAN_POINT ( 'NONE',  ( 22.26710026944065746, 2.334480711795404506, 5.248520767630765249 ) ) ;
#34818=VERTEX_POINT ( 'NONE', #32890 ) ;
#34819=CARTESIAN_POINT ( 'NONE',  ( 24.35198760066796808, 2.925641703088587064, -3.745929113794717491 ) ) ;
#34823=CARTESIAN_POINT ( 'NONE',  ( 21.85643539959779247, -13.31640034840845388, 0.8419676367911695936 ) ) ;
#34827=CARTESIAN_POINT ( 'NONE',  ( 85.02879235234962607, 2.798117532367836446, 2.624272742801059710 ) ) ;
#34828=ORIENTED_EDGE ( 'NONE', *, *, #39880, .F. ) ;
#34830=CARTESIAN_POINT ( 'NONE',  ( 14.74375015214041973, -5.597190475337525228, 2.503889630996063875 ) ) ;
#34831=CARTESIAN_POINT ( 'NONE',  ( 33.46254251190648432, -3.085782718482933618, -5.429037072268634745 ) ) ;
#34834=CARTESIAN_POINT ( 'NONE',  ( -72.91754375945518518, 1.351626832663766820, 10.95472414578862441 ) ) ;
#34838=CARTESIAN_POINT ( 'NONE',  ( 28.66061354658119953, -3.315359872734950031, 4.679579922280550086 ) ) ;
#34840=CARTESIAN_POINT ( 'NONE',  ( 33.11155473229664636, -0.1547796613981889668, 4.947169480470523517 ) ) ;
#34847=CARTESIAN_POINT ( 'NONE',  ( 87.76685765732969458, -0.2261755903657670097, -3.756757151743586931 ) ) ;
#34849=DIRECTION ( 'NONE',  ( 0.000000000000000000, 0.000000000000000000, 1.000000000000000000 ) ) ;
#34850=CARTESIAN_POINT ( 'NONE',  ( -4.890026461918812295, -8.951974136083761024, 6.000000000000000000 ) ) ;
#34854=CARTESIAN_POINT ( 'NONE',  ( 24.58106864520391710, 2.978418058025279258, 3.576134102654449087 ) ) ;
#34864=CARTESIAN_POINT ( 'NONE',  ( 16.86596627815397653, 9.683932516527400836, -2.782816404980593905 ) ) ;
#34867=ORIENTED_EDGE ( 'NONE', *, *, #38798, .T. ) ;
#34873=CARTESIAN_POINT ( 'NONE',  ( 29.67594332454466866, -2.985454744488035494, -5.114964129314456542 ) ) ;
#34881=FACE_OUTER_BOUND ( 'NONE', #38260, .T. ) ;
#34883=CARTESIAN_POINT ( 'NONE',  ( 37.09992950587152194, -2.920862267133551793, -5.996321585650099095 ) ) ;
#34888=CARTESIAN_POINT ( 'NONE',  ( -77.33993978126859759, 9.671531369715314241, 9.242830849232364088 ) ) ;
#34890=CARTESIAN_POINT ( 'NONE',  ( 21.92337503799926424, -12.52192678573947582, 2.500000000000000444 ) ) ;
#34899=CARTESIAN_POINT ( 'NONE',  ( 30.85955166002529282, -3.509934588350169360, 4.878265527032272786 ) ) ;
#34900=CARTESIAN_POINT ( 'NONE',  ( 22.43458216738055100, 3.371505658154835494, 4.287311446981358465 ) ) ;
#34905=CARTESIAN_POINT ( 'NONE',  ( 23.14179388839477269, 4.049790476811788942, 3.073817882771325838 ) ) ;
#34914=CARTESIAN_POINT ( 'NONE',  ( 26.64323651376993496, 1.020623712725687415, 4.378694421187283581 ) ) ;
#34920=CARTESIAN_POINT ( 'NONE',  ( 24.76528640762570888, -1.939968142380837701, -6.533370004292007316 ) ) ;
#34923=CARTESIAN_POINT ( 'NONE',  ( -75.71907068449459643, 8.624194553058243784, 8.809091513226231740 ) ) ;
#34926=CARTESIAN_POINT ( 'NONE',  ( -81.80172258451945311, 10.46396458320884371, -1.097114612388527588 ) ) ;
#34927=CARTESIAN_POINT ( 'NONE',  ( 32.89342118928954761, -3.693192685043988011, -5.116248522870010973 ) ) ;
#34928=CARTESIAN_POINT ( 'NONE',  ( 34.79218682057849321, -3.833549442645881378, -5.378504871664683940 ) ) ;
#34936=CARTESIAN_POINT ( 'NONE',  ( 23.18106065147113526, 1.013842311355323433, -5.509883555410340250 ) ) ;
#34937=CARTESIAN_POINT ( 'NONE',  ( 32.24397170968010329, 0.1813167479581142549, -4.768898611949658140 ) ) ;
#34938=CARTESIAN_POINT ( 'NONE',  ( 18.51265066094652667, 11.53724448403076863, -2.500000000000001332 ) ) ;
#34942=CARTESIAN_POINT ( 'NONE',  ( 86.96369117609759769, -0.5876503451053297633, 5.665127693518188678 ) ) ;
#34943=CIRCLE ( 'NONE', #2728, 10.00000000000000888 ) ;
#34945=CARTESIAN_POINT ( 'NONE',  ( 25.54921697257007196, 2.203847488687706857, 4.114390114421843769 ) ) ;
#34957=DIRECTION ( 'NONE',  ( 1.000000000000000000, 0.000000000000000000, 0.000000000000000000 ) ) ;
#34958=EDGE_LOOP ( 'NONE', ( #36031, #25270, #24813, #13979 ) ) ;
#34961=B_SPLINE_CURVE_WITH_KNOTS ( 'NONE', 3,
 ( #9263, #2515, #8852, #15446, #5784, #18322 ),
 .UNSPECIFIED., .F., .F.,
 ( 4, 2, 4 ),
 ( 0.0009802349148204147003, 0.003915514348654383289, 0.006850793782488352746 ),
 .UNSPECIFIED. ) ;
#34965=CARTESIAN_POINT ( 'NONE',  ( 33.87323733507539458, -5.307943772420733453, -1.870510103425834458 ) ) ;
#34966=CARTESIAN_POINT ( 'NONE',  ( 21.84352692530194773, 5.886300334905539167, -3.168733228457595086 ) ) ;
#34973=CARTESIAN_POINT ( 'NONE',  ( -81.58461690839780545, -5.624039435740707304, -2.430449384178134942 ) ) ;
#34978=CARTESIAN_POINT ( 'NONE',  ( 21.71191031684054806, 6.329465815346970281, -3.192820326339156800 ) ) ;
#34981=DIRECTION ( 'NONE',  ( -1.000000000000000000, 0.000000000000000000, 0.000000000000000000 ) ) ;
#34984=DIRECTION ( 'NONE',  ( 0.000000000000000000, -1.000000000000000000, 0.000000000000000000 ) ) ;
#34987=CARTESIAN_POINT ( 'NONE',  ( 36.89687251559261227, -3.001234578891534444, 5.965047328928867465 ) ) ;
#34989=CARTESIAN_POINT ( 'NONE',  ( 85.06303677129686491, 2.810884359907178442, 0.2996589496366894867 ) ) ;
#34998=CARTESIAN_POINT ( 'NONE',  ( -80.93573588528884954, -6.594316608410932368, -0.1743350153730407748 ) ) ;
#35001=ORIENTED_EDGE ( 'NONE', *, *, #20917, .F. ) ;
#35005=CARTESIAN_POINT ( 'NONE',  ( 21.99376790462624953, 1.189524801706998369, 6.708885966919416077 ) ) ;
#35011=CARTESIAN_POINT ( 'NONE',  ( 86.04131037299104889, 1.712041018818101001, 4.434258418812279778 ) ) ;
#35015=CARTESIAN_POINT ( 'NONE',  ( 21.83619960343240152, 4.667953057257941296, -3.941150944126043054 ) ) ;
#35016=ORIENTED_EDGE ( 'NONE', *, *, #20110, .F. ) ;
#35019=CARTESIAN_POINT ( 'NONE',  ( 21.85643539959776049, -11.26069278398387929, -1.499473835228683383 ) ) ;
#35020=CARTESIAN_POINT ( 'NONE',  ( 21.85643539959341197, 4.025506921158589435, -3.384544483166171069 ) ) ;
#35024=CARTESIAN_POINT ( 'NONE',  ( 84.84279093542515682, 3.008464274580536113, -1.251974654204536908 ) ) ;
#35027=CARTESIAN_POINT ( 'NONE',  ( 31.37023632097418613, -3.077502701871681623, 5.102482088558111251 ) ) ;
#35028=CARTESIAN_POINT ( 'NONE',  ( 37.04378618670349255, -2.892922215093147287, -5.987976760426303890 ) ) ;
#35037=CARTESIAN_POINT ( 'NONE',  ( 32.89336775635678833, -3.694078216458867914, 5.115754129267041428 ) ) ;
#35040=CARTESIAN_POINT ( 'NONE',  ( 35.21901955015318464, -1.051018187038459395, 5.414466639731517539 ) ) ;
#35045=CARTESIAN_POINT ( 'NONE',  ( -75.55075356912415430, 10.07540306679061537, -8.875197024773052945 ) ) ;
#35046=CARTESIAN_POINT ( 'NONE',  ( -70.92837670882107659, -20.78299143688747819, 38.00000000000000711 ) ) ;
#35048=( NAMED_UNIT ( * ) SI_UNIT ( $, .STERADIAN. ) SOLID_ANGLE_UNIT ( ) );
#35053=CARTESIAN_POINT ( 'NONE',  ( 23.15788130583384330, 3.915193624451748899, 3.265821563917845616 ) ) ;
#35061=CARTESIAN_POINT ( 'NONE',  ( 16.61524737713339306, 9.466292241573675881, -2.799609213114734096 ) ) ;
#35072=CARTESIAN_POINT ( 'NONE',  ( 17.73032609328552311, 9.401816658683801009, 2.500000000001603606 ) ) ;
#35073=CARTESIAN_POINT ( 'NONE',  ( 31.79760674661912745, -3.928098387035230843, -4.516596916592202859 ) ) ;
#35079=CARTESIAN_POINT ( 'NONE',  ( -69.92837670882107659, -20.78299143688747819, 38.00000000000000711 ) ) ;
#35082=CARTESIAN_POINT ( 'NONE',  ( 37.14564460383387257, -2.766510155177709596, -6.000552212166151200 ) ) ;
#35086=CARTESIAN_POINT ( 'NONE',  ( -80.92826776361104635, 10.51124857772332888, 4.601267702880412536 ) ) ;
#35089=CARTESIAN_POINT ( 'NONE',  ( 22.04113503551895192, -11.47825136006098568, -2.500000000000000000 ) ) ;
#35090=CARTESIAN_POINT ( 'NONE',  ( 21.85643539959775694, -14.72209017798242847, 2.500000000000000000 ) ) ;
#35097=CARTESIAN_POINT ( 'NONE',  ( 23.54004410631070598, 2.893922283036513665, 4.010806277782499762 ) ) ;
#35101=CARTESIAN_POINT ( 'NONE',  ( 22.87842739364366906, 4.334684949232740614, 3.062211079084044663 ) ) ;
#35104=DIRECTION ( 'NONE',  ( -0.000000000000000000, -1.000000000000000000, -0.000000000000000000 ) ) ;
#35107=CARTESIAN_POINT ( 'NONE',  ( 26.04583467364012250, 0.8117774137170248316, 4.422459632103364235 ) ) ;
#35115=CARTESIAN_POINT ( 'NONE',  ( 25.50488203239457974, -4.522972804344248310, -2.044314315604920829 ) ) ;
#35118=CARTESIAN_POINT ( 'NONE',  ( -75.60324101774568817, -3.659505646876107132, 10.24606351670531801 ) ) ;
#35119=CARTESIAN_POINT ( 'NONE',  ( 22.28556454289693534, 0.2471178846263055173, -7.129343698686286146 ) ) ;
#35124=CARTESIAN_POINT ( 'NONE',  ( 29.62493821037406505, -3.849392467081528046, -4.318428163209237169 ) ) ;
#35125=CARTESIAN_POINT ( 'NONE',  ( 36.87150573566773204, -2.086597623118781719, -5.863914357448089198 ) ) ;
#35127=CARTESIAN_POINT ( 'NONE',  ( 17.52987946391127139, 9.005527010368655993, 2.875160436497226524 ) ) ;
#35135=AXIS2_PLACEMENT_3D ( 'NONE', #1671, #19789, #35653 ) ;
#35136=CARTESIAN_POINT ( 'NONE',  ( 22.16990573667704822, 0.5916043469538394550, -7.020939071362018780 ) ) ;
#35137=CARTESIAN_POINT ( 'NONE',  ( 29.64522198537066089, 1.158353845804762638, -4.258353192414280564 ) ) ;
#35144=CARTESIAN_POINT ( 'NONE',  ( 87.52176134051316581, -1.326109120332903846, -4.764847963194966063 ) ) ;
#35147=CARTESIAN_POINT ( 'NONE',  ( -81.29308920802959904, 10.50256859448236746, -3.581322989614748042 ) ) ;
#35162=CARTESIAN_POINT ( 'NONE',  ( 21.85643539959777826, -4.218647804531223677, -15.78683364351815221 ) ) ;
#35164=CARTESIAN_POINT ( 'NONE',  ( 21.84013737357207319, 5.905724203777740655, -3.160582246606867596 ) ) ;
#35167=ORIENTED_EDGE ( 'NONE', *, *, #8300, .F. ) ;
#35171=CARTESIAN_POINT ( 'NONE',  ( -73.67079394104450785, -1.142843423449616092, -9.674537367239850028 ) ) ;
#35175=CARTESIAN_POINT ( 'NONE',  ( 85.62750488955801131, 0.9367966501063212936, -5.850367371124844063 ) ) ;
#35176=CARTESIAN_POINT ( 'NONE',  ( -80.92837670882107659, 2.429809908903242555, 12.50000000000000000 ) ) ;
#35178=DIRECTION ( 'NONE',  ( -1.000000000000000000, -2.706168622523821592E-13, 0.000000000000000000 ) ) ;
#35179=CARTESIAN_POINT ( 'NONE',  ( 33.61379031873056533, -1.222676232381281203, 5.452642950465561356 ) ) ;
#35182=LINE ( 'NONE', #33502, #1361 ) ;
#35184=EDGE_CURVE ( 'NONE', #21186, #30067, #34131, .T. ) ;
#35187=CARTESIAN_POINT ( 'NONE',  ( 21.25451707795022571, 3.323545404380253920, 3.523679451088993275 ) ) ;
#35191=CARTESIAN_POINT ( 'NONE',  ( 88.38542499104009664, -0.9209797785659445957, 1.969977704346236536 ) ) ;
#35201=DIRECTION ( 'NONE',  ( -0.9999026450364576490, -0.01395351027862084224, 0.000000000000000000 ) ) ;
#35206=CARTESIAN_POINT ( 'NONE',  ( 22.50446240958931909, 2.315161088752189400, 5.067441199431872434 ) ) ;
#35216=CARTESIAN_POINT ( 'NONE',  ( 23.45119107970727512, 3.196877576141845534, -3.804540727237317732 ) ) ;
#35217=ORIENTED_EDGE ( 'NONE', *, *, #4448, .T. ) ;
#35218=ORIENTED_EDGE ( 'NONE', *, *, #37599, .T. ) ;
#35220=CARTESIAN_POINT ( 'NONE',  ( 21.85643539959773207, -9.550271554086487313, -10.69920392963802769 ) ) ;
#35222=CARTESIAN_POINT ( 'NONE',  ( 21.86297326093952620, 3.431109414793966028, -3.921173740587788004 ) ) ;
#35225=CARTESIAN_POINT ( 'NONE',  ( 86.06476644049696745, 1.615394338423677079, -5.255309406831162988 ) ) ;
#35228=CARTESIAN_POINT ( 'NONE',  ( 16.20343186231441024, -3.286044633442916751, 2.735335442231370706 ) ) ;
#35229=CARTESIAN_POINT ( 'NONE',  ( 35.94816592885891993, -2.120094059548885745, 5.816978721513569539 ) ) ;
#35232=CARTESIAN_POINT ( 'NONE',  ( 25.29827998133839628, 1.741210327013272607, -4.154806450938097306 ) ) ;
#35238=CARTESIAN_POINT ( 'NONE',  ( 32.91125982496738800, -3.131047002244825794, 5.342996076127907834 ) ) ;
#35241=CARTESIAN_POINT ( 'NONE',  ( 29.48676609661965387, 1.217395433518708492, 4.226912799969553269 ) ) ;
#35262=CARTESIAN_POINT ( 'NONE',  ( 15.42938493869426075, 10.99473164328989405, -2.614526699404854604 ) ) ;
#35263=EDGE_CURVE ( 'NONE', #13934, #36582, #15970, .T. ) ;
#35265=B_SPLINE_CURVE_WITH_KNOTS ( 'NONE', 3,
 ( #7573, #26719, #38656, #7966, #23622, #29601, #36186, #1416 ),
 .UNSPECIFIED., .F., .F.,
 ( 4, 2, 2, 4 ),
 ( 0.001627818838919652990, 0.002602893308734022942, 0.003577967778548392895, 0.005528116718177132800 ),
 .UNSPECIFIED. ) ;
#35272=CARTESIAN_POINT ( 'NONE',  ( 86.92636418897033934, 0.7179065655219835085, -4.964803926638174048 ) ) ;
#35273=CARTESIAN_POINT ( 'NONE',  ( 31.06145916124171436, -2.509195271462365540, -5.777646538787225339 ) ) ;
#35275=CARTESIAN_POINT ( 'NONE',  ( 21.85643539959777115, -13.25467889390307796, 0.8368004220631568568 ) ) ;
#35278=AXIS2_PLACEMENT_3D ( 'NONE', #4153, #32759, #26770 ) ;
#35281=CARTESIAN_POINT ( 'NONE',  ( 34.12188614642886364, -3.607431673937933958, -5.453371772074238955 ) ) ;
#35285=CARTESIAN_POINT ( 'NONE',  ( -70.92837670882107659, 10.37661300689600097, 0.000000000000000000 ) ) ;
#35288=CARTESIAN_POINT ( 'NONE',  ( 21.88090590480122444, -13.32625148503419865, 2.500000000000000444 ) ) ;
#35296=CARTESIAN_POINT ( 'NONE',  ( 22.21409233198261290, 3.844288165656574829, 4.110153234016473256 ) ) ;
#35301=CARTESIAN_POINT ( 'NONE',  ( 23.14157197170704805, 4.048751080929327451, 3.076040433570303989 ) ) ;
#35302=CARTESIAN_POINT ( 'NONE',  ( -81.90888476619602443, -6.597313057213483489, -0.6545554231109771415 ) ) ;
#35303=CARTESIAN_POINT ( 'NONE',  ( 19.12733620826224978, -3.077968911084931758, 3.134593501090364054 ) ) ;
#35309=CARTESIAN_POINT ( 'NONE',  ( 25.40142685431079528, 0.6874522221836151248, 4.599600658783209006 ) ) ;
#35315=AXIS2_PLACEMENT_3D ( 'NONE', #20097, #19706, #7341 ) ;
#35321=CARTESIAN_POINT ( 'NONE',  ( 24.54460225945253526, -1.054324096271329614, -6.891227800717186547 ) ) ;
#35325=CARTESIAN_POINT ( 'NONE',  ( -75.48799235854204426, -5.171441145269375816, 8.906435695295353838 ) ) ;
#35326=CARTESIAN_POINT ( 'NONE',  ( 25.40611314139961507, 0.6577627199992637230, -4.600311117202987354 ) ) ;
#35330=CARTESIAN_POINT ( 'NONE',  ( 34.14206359931419854, -3.846217481392709914, -5.236744094428941843 ) ) ;
#35333=CARTESIAN_POINT ( 'NONE',  ( 19.31057600782361305, 7.430049097904062094, 3.124219774106051783 ) ) ;
#35337=AXIS2_PLACEMENT_3D ( 'NONE', #33902, #30810, #31411 ) ;
#35339=CARTESIAN_POINT ( 'NONE',  ( 24.65336533415635856, 1.592875596455870513, -4.500810045853856245 ) ) ;
#35340=CARTESIAN_POINT ( 'NONE',  ( 36.36861739423189022, -1.688192717328701686, -5.711810702524172889 ) ) ;
#35341=CARTESIAN_POINT ( 'NONE',  ( -4.444218661349752963, -35.94265729135299381, 6.000000000000000000 ) ) ;
#35345=CARTESIAN_POINT ( 'NONE',  ( 87.94553049950697243, -1.849565313017166535, -3.579236442506480653 ) ) ;
#35347=CARTESIAN_POINT ( 'NONE',  ( 26.59686585277882998, 1.637759102572657888, 4.330020466781864918 ) ) ;
#35350=CARTESIAN_POINT ( 'NONE',  ( -70.92837670882107659, -23.80776546975053520, 10.00000000000000533 ) ) ;
#35352=( NAMED_UNIT ( * ) SI_UNIT ( $, .STERADIAN. ) SOLID_ANGLE_UNIT ( ) );
#35353=EDGE_CURVE ( 'NONE', #20794, #8875, #3802, .T. ) ;
#35360=AXIS2_PLACEMENT_3D ( 'NONE', #28361, #25080, #6345 ) ;
#35361=CARTESIAN_POINT ( 'NONE',  ( 24.75277909289565770, 2.391494161259001938, 4.069667844307693905 ) ) ;
#35366=CARTESIAN_POINT ( 'NONE',  ( 21.85643539959781023, -13.06032977194142930, 9.178732910485948082 ) ) ;
#35368=CARTESIAN_POINT ( 'NONE',  ( 22.19214921742566204, 5.242882102261849475, -3.093814343854897064 ) ) ;
#35371=VECTOR ( 'NONE', #23715, 1000.000000000000000 ) ;
#35374=DIRECTION ( 'NONE',  ( 1.000000000000000000, 0.000000000000000000, 0.000000000000000000 ) ) ;
#35375=CARTESIAN_POINT ( 'NONE',  ( -72.84127017857981912, 2.226350102246259954, -9.875462825488979135 ) ) ;
#35379=CARTESIAN_POINT ( 'NONE',  ( 84.69769694898896262, 2.275084749292730635, 4.163914512140848068 ) ) ;
#35387=AXIS2_PLACEMENT_3D ( 'NONE', #27082, #39627, #4849 ) ;
#35389=CARTESIAN_POINT ( 'NONE',  ( 36.19429332948913469, -2.231517989824187254, 5.855392854995553620 ) ) ;
#35392=CARTESIAN_POINT ( 'NONE',  ( 86.46420362610733434, 1.237027245193318192, -5.068583899740296772 ) ) ;
#35401=CARTESIAN_POINT ( 'NONE',  ( -78.87124948352045806, -6.567092532003710126, 6.089658418205694090 ) ) ;
#35405=CARTESIAN_POINT ( 'NONE',  ( 25.84952034417671740, 2.048349254327011426, 4.178021515479660941 ) ) ;
#35414=CARTESIAN_POINT ( 'NONE',  ( 85.75260874296688485, 2.036324392267200079, 3.804357317183401754 ) ) ;
#35418=CARTESIAN_POINT ( 'NONE',  ( 22.37633911595722935, 4.133713974500000887, -3.770963387559532087 ) ) ;
#35419=ORIENTED_EDGE ( 'NONE', *, *, #5584, .T. ) ;
#35420=DIRECTION ( 'NONE',  ( -0.000000000000000000, -0.000000000000000000, -1.000000000000000000 ) ) ;
#35422=CARTESIAN_POINT ( 'NONE',  ( 21.85643539959779957, -12.42149291456256499, -5.642648835571736576 ) ) ;
#35423=CARTESIAN_POINT ( 'NONE',  ( 21.86624219161038241, 3.264102293340214622, 3.922476187580718587 ) ) ;
#35426=CARTESIAN_POINT ( 'NONE',  ( 84.79389884800966115, 3.063713526918731223, 0.3112276665278714827 ) ) ;
#35431=CARTESIAN_POINT ( 'NONE',  ( 36.79795713293712112, -2.555754650487687130, -5.949609191187919421 ) ) ;
#35437=CARTESIAN_POINT ( 'NONE',  ( 29.60505900326302609, -3.794812366572309692, 4.412074707466141277 ) ) ;
#35441=CARTESIAN_POINT ( 'NONE',  ( 37.00831260221009700, -3.245544418880986548, 5.947168679556439130 ) ) ;
#35444=CARTESIAN_POINT ( 'NONE',  ( 87.90201547669775550, -2.482640368694746691, -0.9994344668162112866 ) ) ;
#35445=VERTEX_POINT ( 'NONE', #8750 ) ;
#35448=CARTESIAN_POINT ( 'NONE',  ( 0.000000000000000000, 0.000000000000000000, 0.000000000000000000 ) ) ;
#35453=CARTESIAN_POINT ( 'NONE',  ( 23.71906029381402092, 3.521941673742745582, 3.287647665226494098 ) ) ;
#35457=VERTEX_POINT ( 'NONE', #32277 ) ;
#35466=CARTESIAN_POINT ( 'NONE',  ( 23.14565985387361025, 3.365906385940814260, -3.818838018732628292 ) ) ;
#35470=CARTESIAN_POINT ( 'NONE',  ( 29.80812890880734756, -3.278499718192964263, -4.781105184254491824 ) ) ;
#35476=CARTESIAN_POINT ( 'NONE',  ( 35.79586196015494437, -3.408963864873948424, -5.784727818347247918 ) ) ;
#35481=DIRECTION ( 'NONE',  ( -1.000000000000000000, -1.165409145176969993E-16, 0.000000000000000000 ) ) ;
#35483=CARTESIAN_POINT ( 'NONE',  ( 22.81512952464498056, -8.568292043100733224, -2.500000000000000000 ) ) ;
#35486=CARTESIAN_POINT ( 'NONE',  ( 32.98352007369545902, -0.3890908133127232160, 5.239426168307027787 ) ) ;
#35494=CARTESIAN_POINT ( 'NONE',  ( 30.87471915742276707, -3.492139151130889463, 4.893529281628630656 ) ) ;
#35495=CARTESIAN_POINT ( 'NONE',  ( 22.82768571636377075, 3.344825573009538644, 4.025161535770593879 ) ) ;
#35506=CARTESIAN_POINT ( 'NONE',  ( 23.59809321522951819, 0.4335636044344673423, 5.517173434541214228 ) ) ;
#35511=VECTOR ( 'NONE', #21590, 1000.000000000000000 ) ;
#35516=CARTESIAN_POINT ( 'NONE',  ( 22.53953452546943126, -1.608357795960198677, 9.096105908381383998 ) ) ;
#35519=CARTESIAN_POINT ( 'NONE',  ( -78.35162830023389802, -5.279867256489808369, 6.711823625471323496 ) ) ;
#35526=CARTESIAN_POINT ( 'NONE',  ( 35.22022786365597824, -1.048883770861420039, -5.412378490821479815 ) ) ;
#35531=CARTESIAN_POINT ( 'NONE',  ( -62.92837670882106238, 13.37661300689599742, -6.000000000000000000 ) ) ;
#35532=CARTESIAN_POINT ( 'NONE',  ( 23.94445520861282972, 1.171759895968547349, -4.943323473430091042 ) ) ;
#35533=CARTESIAN_POINT ( 'NONE',  ( 34.86059237354090357, -0.8869592652725889481, -5.330962963188696335 ) ) ;
#35545=CARTESIAN_POINT ( 'NONE',  ( -81.60592086609160845, 10.48184527842860980, -2.319392075440308787 ) ) ;
#35550=ORIENTED_EDGE ( 'NONE', *, *, #29347, .F. ) ;
#35555=CARTESIAN_POINT ( 'NONE',  ( 33.88603132824229647, -5.388632132188243773, 1.367569066300536429 ) ) ;
#35562=CARTESIAN_POINT ( 'NONE',  ( 33.62997687085571386, -4.269399587632154436, -4.589598755017198606 ) ) ;
#35568=CARTESIAN_POINT ( 'NONE',  ( 14.75101795178193775, -5.142163552057975373, -2.499999999999998668 ) ) ;
#35570=CARTESIAN_POINT ( 'NONE',  ( -73.12379269740060295, 4.558640974120507394, -9.815543729773533954 ) ) ;
#35574=CARTESIAN_POINT ( 'NONE',  ( 87.26468549332315661, -1.699173523771937644, 4.325011594718342067 ) ) ;
#35578=EDGE_CURVE ( 'NONE', #5866, #33153, #26881, .T. ) ;
#35585=CARTESIAN_POINT ( 'NONE',  ( 36.89727170037077997, -3.002153245520217784, 5.965109631367820242 ) ) ;
#35586=ADVANCED_FACE ( 'NONE', ( #24143 ), #30130, .F. ) ;
#35588=CARTESIAN_POINT ( 'NONE',  ( 86.54367451126900335, 1.050056116286632646, -5.670096781828877219 ) ) ;
#35603=CARTESIAN_POINT ( 'NONE',  ( 23.60946143526467722, 2.060598013451824251, 4.567481006929359211 ) ) ;
#35611=CARTESIAN_POINT ( 'NONE',  ( 22.33768170137506814, 4.516987467366701203, -3.522961905446787334 ) ) ;
#35616=CARTESIAN_POINT ( 'NONE',  ( 21.85643539959777115, -1.469530054879572223, 14.38030055974112464 ) ) ;
#35617=CARTESIAN_POINT ( 'NONE',  ( 18.10407751947404265, 13.71956107776613543, 3.198739209386171733 ) ) ;
#35621=CARTESIAN_POINT ( 'NONE',  ( 85.86339947292255204, 1.596523033150343718, -5.427711696011725984 ) ) ;
#35625=CARTESIAN_POINT ( 'NONE',  ( 31.02717173337874002, -3.764723011120618690, 4.607707110895616687 ) ) ;
#35627=CARTESIAN_POINT ( 'NONE',  ( 36.91040168402551558, -2.640011690967155378, -5.967158882866976377 ) ) ;
#35629=CARTESIAN_POINT ( 'NONE',  ( 84.47382700867750316, 2.558083702081526134, -3.350542113956249679 ) ) ;
#35633=EDGE_CURVE ( 'NONE', #24927, #13035, #5214, .T. ) ;
#35637=CARTESIAN_POINT ( 'NONE',  ( 30.74906057277648586, -3.703379513678140444, 4.639682255467033833 ) ) ;
#35640=CARTESIAN_POINT ( 'NONE',  ( 35.73082939662619140, -1.303437433980812576, 5.537266709372846485 ) ) ;
#35643=CARTESIAN_POINT ( 'NONE',  ( 86.76920234060486337, -1.029458178097735654, 5.350787913367871518 ) ) ;
#35645=CARTESIAN_POINT ( 'NONE',  ( -70.92837670882107659, -56.35932253828835314, 0.000000000000000000 ) ) ;
#35650=CARTESIAN_POINT ( 'NONE',  ( 21.89662549548976500, 5.563294812639966835, 3.306681051183087305 ) ) ;
#35653=DIRECTION ( 'NONE',  ( 1.000000000000000000, 0.000000000000000000, 0.000000000000000000 ) ) ;
#35658=CARTESIAN_POINT ( 'NONE',  ( 22.27817917822705951, 5.092324266975621683, -3.633448080353249399 ) ) ;
#35668=CARTESIAN_POINT ( 'NONE',  ( 85.75774791330482572, 2.030551832223961295, -3.840166728450957301 ) ) ;
#35669=CARTESIAN_POINT ( 'NONE',  ( 32.01248540970218670, -4.887874588265229470, -2.123135123820048875 ) ) ;
#35671=DIRECTION ( 'NONE',  ( -0.000000000000000000, -0.000000000000000000, -1.000000000000000000 ) ) ;
#35676=CARTESIAN_POINT ( 'NONE',  ( 31.86214199327330121, -0.1501766581728601335, -5.152687107714187142 ) ) ;
#35681=DIRECTION ( 'NONE',  ( -0.000000000000000000, -0.000000000000000000, -1.000000000000000000 ) ) ;
#35686=CARTESIAN_POINT ( 'NONE',  ( 36.46016930148370250, -3.391369413551937217, 5.869954818313481759 ) ) ;
#35699=CARTESIAN_POINT ( 'NONE',  ( 22.87846517050438067, 4.335907691735916281, 3.060191673758243969 ) ) ;
#35704=CARTESIAN_POINT ( 'NONE',  ( 26.71945218434455427, 0.9447924085842542841, 4.381674605026809388 ) ) ;
#35707=ADVANCED_FACE ( 'NONE', ( #3385 ), #21686, .F. ) ;
#35713=CARTESIAN_POINT ( 'NONE',  ( 22.81791704898701667, -6.824503531841428661, 2.299112860430994054 ) ) ;
#35716=CARTESIAN_POINT ( 'NONE',  ( -72.63519498226254711, -1.653156654010232041, 9.855318911829444417 ) ) ;
#35717=CARTESIAN_POINT ( 'NONE',  ( 24.12370628256579508, 0.4970018228905133673, -5.094551904089473560 ) ) ;
#35720=CARTESIAN_POINT ( 'NONE',  ( 36.88786849831456749, -3.351047888682084697, -5.910680165042082379 ) ) ;
#35721=CARTESIAN_POINT ( 'NONE',  ( 30.79114401576465809, -3.336758667098143061, -4.962072607841499838 ) ) ;
#35730=ADVANCED_FACE ( 'NONE', ( #21480 ), #15699, .F. ) ;
#35738=CARTESIAN_POINT ( 'NONE',  ( 87.47045099524558509, -1.608924759093422807, 4.367130927193085377 ) ) ;
#35749=CARTESIAN_POINT ( 'NONE',  ( 37.07689334178120077, -2.357884832068502856, 5.940193581006886880 ) ) ;
#35754=CARTESIAN_POINT ( 'NONE',  ( 18.29952987130526765, 8.276640680725938282, -2.983475682558551334 ) ) ;
#35757=CARTESIAN_POINT ( 'NONE',  ( 33.45716606812183613, -3.829385970599605393, -5.093809925484540813 ) ) ;
#35758=CARTESIAN_POINT ( 'NONE',  ( 21.71434179704859346, 6.308304841617775161, -3.200288761970310869 ) ) ;
#35764=DIRECTION ( 'NONE',  ( 0.000000000000000000, 1.000000000000000000, 0.000000000000000000 ) ) ;
#35766=CARTESIAN_POINT ( 'NONE',  ( -76.37480731197182138, -4.247693215982008219, -9.858617499677098550 ) ) ;
#35778=CARTESIAN_POINT ( 'NONE',  ( 22.92125608552839466, 2.653312946985113552, 3.783814383456351127 ) ) ;
#35780=CARTESIAN_POINT ( 'NONE',  ( 85.38025200535193449, 2.454573153073208225, 3.240196491381199362 ) ) ;
#35783=B_SPLINE_CURVE_WITH_KNOTS ( 'NONE', 3,
 ( #7004, #10287, #26547, #7403, #22861, #13789, #29239, #1252, #16465, #10082, #36024, #20354, #19762, #23456, #22668, #29037, #4337, #7604, #13978, #1047, #38687, #7801, #10484, #35829, #841, #32343, #10882, #38482, #35629, #23064, #32538, #10681, #20156, #32738, #13373, #32933, #4721, #20418, #20023, #38753, #36281, #32999, #33421, #27012, #13849, #36481, #7466, #23323, #10547, #26815, #20615, #33201, #26419, #1506, #23125, #39557, #14040, #32604, #35892, #4402, #20825, #1314, #16923, #4593, #1711, #11341, #38948, #17723, #36093, #26221, #26615, #8056 ),
 .UNSPECIFIED., .F., .F.,
 ( 4, 2, 2, 2, 2, 2, 2, 2, 1, 1, 1, 1, 1, 2, 2, 2, 2, 2, 1, 1, 1, 1, 1, 2, 2, 2, 2, 1, 1, 1, 1, 1, 2, 2, 2, 1, 1, 1, 2, 2, 2, 1, 1, 1, 1, 2, 4 ),
 ( 0.5000000000000000000, 0.5601148001498211793, 0.6202296002996423585, 0.6502870003745532257, 0.6803444004494640929, 0.7104018005243749601, 0.7404592005992858272, 0.7406940240373710571, 0.7409288474754562870, 0.7413984943516267467, 0.7423377881039677773, 0.7442163756086496162, 0.7479735506180135163, 0.7554879006367413163, 0.7705166006741968054, 0.8005740007491080057, 0.8606888008989305172, 0.8609236243370157471, 0.8611584477751008659, 0.8616280946512711036, 0.8625673884036118011, 0.8644459759082925299, 0.8682031509176542095, 0.8757175009363780127, 0.8907462009738250641, 0.9208036010487191669, 0.9210384244868041748, 0.9212732479248892936, 0.9217428948010597534, 0.9226821885534011169, 0.9245607760580834000, 0.9283179510674484103, 0.9358323010861785418, 0.9508610011236386939, 0.9513306479998092646, 0.9518002948759799464, 0.9527395886283216431, 0.9546181761330045923, 0.9583753511423709348, 0.9658897011611035088, 0.9661245245991884056, 0.9663593480372733024, 0.9668289949134435401, 0.9677682886657839045, 0.9696468761704649664, 0.9734040511798274231, 0.9809184011985525586 ),
 .UNSPECIFIED. ) ;
#35787=CARTESIAN_POINT ( 'NONE',  ( -80.56383756236691340, 11.49139298559813582, -2.708314019505869474 ) ) ;
#35793=AXIS2_PLACEMENT_3D ( 'NONE', #28925, #19048, #31612 ) ;
#35798=CARTESIAN_POINT ( 'NONE',  ( 25.78559136093029380, 1.048118573953673582, 4.433432929157029356 ) ) ;
#35801=B_SPLINE_CURVE_WITH_KNOTS ( 'NONE', 3,
 ( #10537, #3796, #22916, #28479, #286, #28890, #13234, #6865, #1107, #6667, #19419, #698, #29091, #38335, #3998 ),
 .UNSPECIFIED., .F., .F.,
 ( 4, 1, 1, 1, 1, 1, 1, 1, 2, 2, 4 ),
 ( 0.000000000000000000, 0.2500000000002247647, 0.3750000000003386735, 0.4375000000003986811, 0.4687500000004286571, 0.4843750000004435896, 0.4921875000004510281, 0.4960937500004519163, 0.4980468750004553025, 0.5000000000004587442, 1.000000000000000000 ),
 .UNSPECIFIED. ) ;
#35805=CARTESIAN_POINT ( 'NONE',  ( 37.83867290611771494, -6.084034091406928191, 6.000000000000000000 ) ) ;
#35809=CARTESIAN_POINT ( 'NONE',  ( 23.92706582939273474, 3.251021385653534601, -3.516417206103825688 ) ) ;
#35813=CARTESIAN_POINT ( 'NONE',  ( 22.63946314531691328, -3.430231901737621492, -8.286483013797429464 ) ) ;
#35814=CARTESIAN_POINT ( 'NONE',  ( 18.03538663863764668, 13.77327480705089258, 8.406736845118375017E-13 ) ) ;
#35815=CARTESIAN_POINT ( 'NONE',  ( 17.36540171046607384, 9.558839590344177850, 2.500000000000280664 ) ) ;
#35818=CARTESIAN_POINT ( 'NONE',  ( 88.80100535589549793, -2.068446212231642711, -0.8863989573356614304 ) ) ;
#35822=CARTESIAN_POINT ( 'NONE',  ( 14.62163843994035517, -5.048694678019860937, 2.488458322851438975 ) ) ;
#35826=CARTESIAN_POINT ( 'NONE',  ( 23.83095679137812084, -2.714704696622131319, -3.925795179799298928 ) ) ;
#35827=CARTESIAN_POINT ( 'NONE',  ( 25.29653240654878132, 1.736439669007842523, -4.154533699626928644 ) ) ;
#35829=CARTESIAN_POINT ( 'NONE',  ( 84.13406293396636215, 2.976669663089178020, -1.005002158774620069 ) ) ;
#35834=CARTESIAN_POINT ( 'NONE',  ( 31.25759568107904585, -2.934864719164037794, -5.084901792477391602 ) ) ;
#35835=ORIENTED_EDGE ( 'NONE', *, *, #40468, .F. ) ;
#35836=ORIENTED_EDGE ( 'NONE', *, *, #17895, .F. ) ;
#35837=CARTESIAN_POINT ( 'NONE',  ( 32.06846522142977562, 0.2517277866219041482, 4.728932550735457596 ) ) ;
#35841=CARTESIAN_POINT ( 'NONE',  ( 86.23726074625430726, -0.1810272084941833837, 5.933124737898375578 ) ) ;
#35847=CARTESIAN_POINT ( 'NONE',  ( 23.67393339541625608, 3.433482753640386242, 3.460823878934576658 ) ) ;
#35855=CARTESIAN_POINT ( 'NONE',  ( 20.51835354428452618, 5.903611222923889734, -3.408783327478037695 ) ) ;
#35857=EDGE_LOOP ( 'NONE', ( #37731, #16657, #30666, #37275, #33411, #14604, #9472, #13296, #917, #14641, #37159, #15266, #18141, #20934, #36620, #5975, #4979, #26358, #13392, #3161, #9419, #26246, #19130, #323, #29118, #9195, #3462 ) ) ;
#35858=CARTESIAN_POINT ( 'NONE',  ( 22.89638698299516761, 2.867431784428169816, -4.347809372303917286 ) ) ;
#35863=CYLINDRICAL_SURFACE ( 'NONE', #36151, 31.65266504832700534 ) ;
#35865=LINE ( 'NONE', #7643, #10961 ) ;
#35867=CARTESIAN_POINT ( 'NONE',  ( 87.25792211136258913, 0.3454849704027515567, -4.698443967043519187 ) ) ;
#35868=CARTESIAN_POINT ( 'NONE',  ( 30.98800548345937855, -0.8519925708576415735, -5.886550247782252221 ) ) ;
#35870=CARTESIAN_POINT ( 'NONE',  ( -69.95445451253289093, -21.04503801384016271, 9.952588678376169895 ) ) ;
#35874=CARTESIAN_POINT ( 'NONE',  ( 23.01850269868070242, 2.906672717470778267, -3.798992069357586487 ) ) ;
#35884=CARTESIAN_POINT ( 'NONE',  ( 35.04481386660351205, -1.406658151536976042, 5.661173613261942350 ) ) ;
#35887=VECTOR ( 'NONE', #24627, 1000.000000000000000 ) ;
#35889=ORIENTED_EDGE ( 'NONE', *, *, #39341, .F. ) ;
#35892=CARTESIAN_POINT ( 'NONE',  ( 85.49121078020223763, 1.153260294498703376, -5.693899337874601230 ) ) ;
#35897=CARTESIAN_POINT ( 'NONE',  ( 22.38310836802325099, 4.932112375007561944, 3.055667184124356783 ) ) ;
#35903=CARTESIAN_POINT ( 'NONE',  ( 27.38238008918371946, 1.067659690267280581, 4.479658769764347959 ) ) ;
#35914=CARTESIAN_POINT ( 'NONE',  ( 24.06190720129734473, 2.407014782553678955, 5.659300396313236448 ) ) ;
#35916=EDGE_LOOP ( 'NONE', ( #34695, #15203, #24400, #16546, #31328, #29639 ) ) ;
#35917=CARTESIAN_POINT ( 'NONE',  ( -76.83427164388604069, -4.573425012487537522, 8.089458760140365357 ) ) ;
#35918=CARTESIAN_POINT ( 'NONE',  ( 25.40388266914231252, 0.6804681363941469385, -4.599446440314822304 ) ) ;
#35921=VERTEX_POINT ( 'NONE', #36068 ) ;
#35924=CARTESIAN_POINT ( 'NONE',  ( 33.11160242427654055, -0.1547984075289232930, -4.947179439121399902 ) ) ;
#35934=CARTESIAN_POINT ( 'NONE',  ( 84.61114100273776728, 2.563204847888557403, 3.486439758113726306 ) ) ;
#35943=ORIENTED_EDGE ( 'NONE', *, *, #34337, .F. ) ;
#35946=CARTESIAN_POINT ( 'NONE',  ( 33.76263401838073008, -4.744560827115999579, 3.708591629391344568 ) ) ;
#35954=CARTESIAN_POINT ( 'NONE',  ( 21.85643539959776760, 9.193408351192362105, 7.099988578988766008 ) ) ;
#35958=CARTESIAN_POINT ( 'NONE',  ( 14.69492309387330664, -4.882291126226618871, 2.500000000000903277 ) ) ;
#35959=CARTESIAN_POINT ( 'NONE',  ( -73.64256375807426025, -3.340549628714686303, -9.625460544246696060 ) ) ;
#35969=B_SPLINE_CURVE_WITH_KNOTS ( 'NONE', 3,
 ( #4344, #29449, #1261, #20165, #13797, #10692, #34383, #21604, #31077, #2264, #15407, #37027, #11690, #2685, #5541, #18287, #20983, #18699, #24895, #9226, #21190, #27357, #27760, #37431, #33973, #18488, #5949, #2887, #39916, #12319, #2479, #12103, #11492, #24270, #27966, #33761, #21398, #18082, #15002, #27562, #5745, #17872, #40314, #24681, #11897 ),
 .UNSPECIFIED., .F., .F.,
 ( 4, 1, 2, 2, 1, 1, 1, 1, 1, 1, 1, 2, 2, 1, 1, 1, 1, 1, 1, 1, 1, 2, 2, 1, 1, 1, 1, 1, 1, 1, 1, 2, 2, 1, 4 ),
 ( 0.01538690458847954794, 0.1384635415149992888, 0.1423096864189528632, 0.1442327588709294284, 0.1461558313229059380, 0.1538481211308128094, 0.1692327007466265243, 0.2000018599782546203, 0.2307710192098827440, 0.2461555988256970695, 0.2480786712776741343, 0.2490402075036624030, 0.2500017437296506717, 0.2538478886336021367, 0.2615401784415042341, 0.3846168153679325186, 0.4461551338311469661, 0.4769242930627539123, 0.4923088726785574409, 0.4961550175825084064, 0.4980780900344842221, 0.4990396262604720468, 0.5000011624864599824, 0.5076934522943629124, 0.6307700892208103483, 0.6923084076840340106, 0.7230775669156456198, 0.7384621465314512578, 0.7461544363393539658, 0.7480775087913299481, 0.7490390450173182169, 0.7495198131303120181, 0.7500005812433059305, 0.7538467261472543424, 1.000000000000000000 ),
 .UNSPECIFIED. ) ;
#35972=CARTESIAN_POINT ( 'NONE',  ( 15.58401231752230842, 10.76254152672632536, -2.638660041548260615 ) ) ;
#35978=CARTESIAN_POINT ( 'NONE',  ( 88.68641656676298624, -1.259067802340008146, 0.2042187262504959744 ) ) ;
#35994=CARTESIAN_POINT ( 'NONE',  ( 21.74229646505971658, 0.4512508753831538377, 8.537182636489522025 ) ) ;
#36001=CARTESIAN_POINT ( 'NONE',  ( 14.69558838330753758, 3.996311804371543985, 6.000000000000000000 ) ) ;
#36005=CARTESIAN_POINT ( 'NONE',  ( 22.94357577811185323, 4.016617617340873636, -3.383606566543657213 ) ) ;
#36008=CARTESIAN_POINT ( 'NONE',  ( 22.35506120569036170, 4.170988562608182626, 6.826273348963533216 ) ) ;
#36009=CARTESIAN_POINT ( 'NONE',  ( 15.27436587416087121, 8.240068014946416497, 3.484044188646821638 ) ) ;
#36013=CARTESIAN_POINT ( 'NONE',  ( 87.91375683397511409, -1.031045523906674033, -4.794500835981626352 ) ) ;
#36014=CARTESIAN_POINT ( 'NONE',  ( -17.27251170661583402, -8.656638842136340273, 6.000000000000000000 ) ) ;
#36019=AXIS2_PLACEMENT_3D ( 'NONE', #28875, #6849, #29077 ) ;
#36021=CARTESIAN_POINT ( 'NONE',  ( 33.96234278159153774, -3.201214304958433843, -5.507042992068187814 ) ) ;
#36022=CARTESIAN_POINT ( 'NONE',  ( 34.77309710796683362, -3.158688717209038543, -5.633580812866661347 ) ) ;
#36024=CARTESIAN_POINT ( 'NONE',  ( 84.18174941840253211, 2.918289511092787780, 1.655912298728576815 ) ) ;
#36026=CARTESIAN_POINT ( 'NONE',  ( 29.31288836536752029, -3.867418896606279688, -4.320839978493723699 ) ) ;
#36031=ORIENTED_EDGE ( 'NONE', *, *, #8685, .F. ) ;
#36033=CARTESIAN_POINT ( 'NONE',  ( 25.73396967306546657, 2.637378028382216577, 3.518935617133692961 ) ) ;
#36036=EDGE_CURVE ( 'NONE', #23904, #8980, #13259, .T. ) ;
#36038=CARTESIAN_POINT ( 'NONE',  ( 87.89153558153043377, -2.469980296156808475, 1.041252188155484149 ) ) ;
#36043=VECTOR ( 'NONE', #2608, 1000.000000000000000 ) ;
#36048=CARTESIAN_POINT ( 'NONE',  ( 22.95533607554538946, 3.919416367836303206, 3.470897119079664250 ) ) ;
#36054=CARTESIAN_POINT ( 'NONE',  ( 22.13111492170271077, -2.652485278638713861, -3.660493745205452232 ) ) ;
#36057=CARTESIAN_POINT ( 'NONE',  ( 24.01690006195003235, 2.804734595017727372, -3.921598103404013713 ) ) ;
#36061=CARTESIAN_POINT ( 'NONE',  ( 24.12827207576258104, 2.707173303308993528, -3.972198420524792439 ) ) ;
#36066=CARTESIAN_POINT ( 'NONE',  ( 85.88453125851971492, 1.888142761377891832, -4.329341218647970280 ) ) ;
#36067=CARTESIAN_POINT ( 'NONE',  ( 31.38399832331403161, -1.255798082282080008, 5.972680360385385079 ) ) ;
#36068=CARTESIAN_POINT ( 'NONE',  ( 4.200390093233091093, -29.56993018339339940, 6.000000000000000000 ) ) ;
#36070=CARTESIAN_POINT ( 'NONE',  ( -73.08996536204158190, 0.4269082215137926517, -10.93610844367175261 ) ) ;
#36074=CARTESIAN_POINT ( 'NONE',  ( 20.66010564244338354, 4.228422099284120605, -3.378132346044065315 ) ) ;
#36079=LINE ( 'NONE', #890, #24358 ) ;
#36084=CARTESIAN_POINT ( 'NONE',  ( 23.13399157829620734, 3.188628281914902107, 3.769246907791176771 ) ) ;
#36087=EDGE_CURVE ( 'NONE', #32959, #32120, #26042, .T. ) ;
#36092=CARTESIAN_POINT ( 'NONE',  ( 86.18567091879171471, -0.09149539399120916461, -5.958500351614375745 ) ) ;
#36093=CARTESIAN_POINT ( 'NONE',  ( 85.80843657999245977, 0.6132022408405360947, -5.953866110284497637 ) ) ;
#36097=VERTEX_POINT ( 'NONE', #23339 ) ;
#36098=CARTESIAN_POINT ( 'NONE',  ( 24.38107346567219480, 3.152084082324316139, 3.324539938462093058 ) ) ;
#36105=CARTESIAN_POINT ( 'NONE',  ( 23.58291269724494654, 0.3979865196799417526, 5.534407531907699074 ) ) ;
#36109=DIRECTION ( 'NONE',  ( -0.9999026450364576490, -0.01395351027862084224, 0.000000000000000000 ) ) ;
#36113=CARTESIAN_POINT ( 'NONE',  ( 27.46505532721044318, 0.1961140298417080874, 5.884446595982424810 ) ) ;
#36117=CARTESIAN_POINT ( 'NONE',  ( 26.75173391963811298, 0.8966615678213633034, -4.382807213102920763 ) ) ;
#36121=CARTESIAN_POINT ( 'NONE',  ( 36.87059600844250440, -2.088011045112093900, -5.864540870269784101 ) ) ;
#36129=ORIENTED_EDGE ( 'NONE', *, *, #14631, .F. ) ;
#36133=EDGE_CURVE ( 'NONE', #6636, #34747, #16734, .T. ) ;
#36134=VERTEX_POINT ( 'NONE', #29319 ) ;
#36135=CARTESIAN_POINT ( 'NONE',  ( 85.07031394220433640, 1.982162274098862476, -4.809620659748507165 ) ) ;
#36139=CARTESIAN_POINT ( 'NONE',  ( -70.92837670882107659, -37.87473357531881391, 6.000000000000002665 ) ) ;
#36144=VERTEX_POINT ( 'NONE', #38363 ) ;
#36146=CARTESIAN_POINT ( 'NONE',  ( 33.78549810770471851, -4.844043753022709176, 3.475806433684239583 ) ) ;
#36149=B_SPLINE_CURVE_WITH_KNOTS ( 'NONE', 3,
 ( #9968, #27031, #20436, #14459, #21266, #36907, #5209, #1939, #14057, #1729, #2344, #27226, #8686, #36698, #5413, #17335, #30534, #11361, #26831, #17744, #33636, #23929, #33839, #8272, #29912, #7887, #8481 ),
 .UNSPECIFIED., .F., .F.,
 ( 4, 2, 2, 1, 1, 1, 1, 2, 2, 2, 1, 1, 1, 1, 1, 2, 2, 4 ),
 ( 0.000000000000000000, 0.08933253011160632862, 0.09003044050310334001, 0.09072835089460033753, 0.09212417167759436032, 0.09491581324358161487, 0.1004990963755560823, 0.1116656626395058499, 0.1339987951674053990, 0.1341732727652801827, 0.1343477503631549386, 0.1346967055589049223, 0.1353946159504048896, 0.1367904367334048243, 0.1395820782994046938, 0.1451653614314038776, 0.1563319276954028281, 0.1786650602234007013 ),
 .UNSPECIFIED. ) ;
#36151=AXIS2_PLACEMENT_3D ( 'NONE', #7641, #4565, #17092 ) ;
#36153=CARTESIAN_POINT ( 'NONE',  ( 18.54920515881659782, 13.18659104987385433, 2.500000000000000000 ) ) ;
#36154=CARTESIAN_POINT ( 'NONE',  ( 21.85643539959774984, 7.798985686765059100, -6.733359799098007414 ) ) ;
#36155=ORIENTED_EDGE ( 'NONE', *, *, #20775, .F. ) ;
#36157=CARTESIAN_POINT ( 'NONE',  ( -61.24591834330252027, -23.80776546975053520, 2.500000000000000000 ) ) ;
#36158=CARTESIAN_POINT ( 'NONE',  ( -72.46315804115566550, 6.112692013474589459, -9.882615271681798319 ) ) ;
#36160=CARTESIAN_POINT ( 'NONE',  ( 37.10495453580936953, -3.127303634092527762, -5.976092241509372016 ) ) ;
#36164=CYLINDRICAL_SURFACE ( 'NONE', #3717, 1.000000000000000444 ) ;
#36166=AXIS2_PLACEMENT_3D ( 'NONE', #20086, #32266, #16579 ) ;
#36170=CARTESIAN_POINT ( 'NONE',  ( -69.42837670882107659, -47.11702805680359063, 5.809475019311128641 ) ) ;
#36173=CARTESIAN_POINT ( 'NONE',  ( 85.09863483756090830, 2.770898922293168809, 1.806811963633389695 ) ) ;
#36177=CARTESIAN_POINT ( 'NONE',  ( 33.33049225550245609, -1.121405412915873256, -5.408427436109264796 ) ) ;
#36181=CARTESIAN_POINT ( 'NONE',  ( -79.78869251280185892, 11.50862393811266138, -4.655148827077255191 ) ) ;
#36186=CARTESIAN_POINT ( 'NONE',  ( 24.93765456293620275, 3.473447388903421196, 1.305885461667957825 ) ) ;
#36188=CARTESIAN_POINT ( 'NONE',  ( 22.50932894906165060, 0.7908534467655897737, 6.383121493648327593 ) ) ;
#36197=CARTESIAN_POINT ( 'NONE',  ( 23.19158755795082882, 3.577708210753886675, -3.605410824286771732 ) ) ;
#36201=CARTESIAN_POINT ( 'NONE',  ( 22.45979449916501736, 0.3571986981647585768, -9.138524188866155029 ) ) ;
#36205=CARTESIAN_POINT ( 'NONE',  ( 86.75210013534866960, -0.2795847087395720298, -5.842668109216860195 ) ) ;
#36211=CARTESIAN_POINT ( 'NONE',  ( 18.24203027604363214, -3.069080384045527410, -3.024498425576051197 ) ) ;
#36212=CARTESIAN_POINT ( 'NONE',  ( 29.10051722050815215, 0.3561458739526577322, -4.748237529565580317 ) ) ;
#36214=CARTESIAN_POINT ( 'NONE',  ( 24.11505776774735921, 0.5870443042865580718, -5.089557059125589866 ) ) ;
#36224=CARTESIAN_POINT ( 'NONE',  ( 30.88296028701921259, 0.6986673433299844804, 4.492958028923911940 ) ) ;
#36228=CARTESIAN_POINT ( 'NONE',  ( 86.31054848189137374, -0.3087909235149370879, 5.883766619840620216 ) ) ;
#36231=VERTEX_POINT ( 'NONE', #13059 ) ;
#36232=VECTOR ( 'NONE', #24983, 1000.000000000000000 ) ;
#36239=CARTESIAN_POINT ( 'NONE',  ( 22.06452787639179647, 5.259082593475454814, 3.268497644756389597 ) ) ;
#36241=EDGE_CURVE ( 'NONE', #24175, #22597, #36149, .T. ) ;
#36245=CARTESIAN_POINT ( 'NONE',  ( 26.13518495524960983, -2.760235698259291492, -4.285425712740152271 ) ) ;
#36246=DIRECTION ( 'NONE',  ( -1.000000000000000000, 0.000000000000000000, 0.000000000000000000 ) ) ;
#36249=CARTESIAN_POINT ( 'NONE',  ( 24.49589214427983208, 2.769561699705143099, -3.859156718590324164 ) ) ;
#36256=CARTESIAN_POINT ( 'NONE',  ( 87.93559242015480493, -0.4157064846058496355, 3.292354338654781998 ) ) ;
#36257=CARTESIAN_POINT ( 'NONE',  ( 30.65010716405877034, -0.4808061152566996399, -5.754690052858093097 ) ) ;
#36261=EDGE_CURVE ( 'NONE', #30067, #1864, #8075, .T. ) ;
#36262=CARTESIAN_POINT ( 'NONE',  ( -81.80090188080514224, -5.603160304130404334, -0.6545554231109831367 ) ) ;
#36266=CARTESIAN_POINT ( 'NONE',  ( 33.68680382786263294, -1.062740808955847660, -5.464038474404074641 ) ) ;
#36269=CARTESIAN_POINT ( 'NONE',  ( 11.29080664838498649, 1.564594260697056104E-15, 6.000000000000000000 ) ) ;
#36273=CARTESIAN_POINT ( 'NONE',  ( 36.86636322194920723, -3.288495969527875040, 5.928692945992483310 ) ) ;
#36277=DIRECTION ( 'NONE',  ( 0.000000000000000000, 1.000000000000000000, 0.000000000000000000 ) ) ;
#36279=FACE_OUTER_BOUND ( 'NONE', #21827, .T. ) ;
#36281=CARTESIAN_POINT ( 'NONE',  ( 84.89441094598296900, 2.017138685944319221, -4.674259599216689764 ) ) ;
#36282=CARTESIAN_POINT ( 'NONE',  ( -80.15742618671445996, 11.51087320173220263, 3.873033802042450180 ) ) ;
#36285=ORIENTED_EDGE ( 'NONE', *, *, #18826, .F. ) ;
#36286=CARTESIAN_POINT ( 'NONE',  ( 22.38435940742265373, 4.925671751812593868, 3.061725572434287557 ) ) ;
#36289=VECTOR ( 'NONE', #3927, 1000.000000000000000 ) ;
#36293=CARTESIAN_POINT ( 'NONE',  ( 27.44318431746329878, 0.9300348501808439750, 4.489570647297722594 ) ) ;
#36294=CARTESIAN_POINT ( 'NONE',  ( 14.77487148941764694, -5.166432627237171893, -2.500000000170817138 ) ) ;
#36302=EDGE_CURVE ( 'NONE', #37237, #22023, #25167, .T. ) ;
#36304=( BOUNDED_SURFACE ( )  B_SPLINE_SURFACE ( 3, 3, ( 
 ( #30215, #23236, #17234, #20735 ),
 ( #26524, #14548, #8166, #29806 ),
 ( #7779, #17635, #17031, #23816 ),
 ( #36001, #35805, #20134, #8374 ),
 ( #29606, #7580, #17841, #20327 ),
 ( #5102, #32715, #27322, #2032 ),
 ( #32909, #36392, #20948, #27122 ) ),
 .UNSPECIFIED., .T., .F., .T. ) 
 B_SPLINE_SURFACE_WITH_KNOTS ( ( 4, 3, 4 ),
 ( 4, 4 ),
 ( 0.000000000000000000, 0.5000000000000000000, 1.000000000000000000 ),
 ( 0.000000000000000000, 1.000000000000000000 ),
 .UNSPECIFIED. ) 
 GEOMETRIC_REPRESENTATION_ITEM ( )  RATIONAL_B_SPLINE_SURFACE ( (
 ( 1.000000000000000000, 0.9563893749471424899, 0.9563893749471424899, 1.000000000000000000),
 ( 0.3333333333333333703, 0.3187964583157141818, 0.3187964583157141818, 0.3333333333333333703),
 ( 0.3333333333333333703, 0.3187964583157141818, 0.3187964583157141818, 0.3333333333333333703),
 ( 1.000000000000000000, 0.9563893749471424899, 0.9563893749471424899, 1.000000000000000000),
 ( 0.3333333333333333703, 0.3187964583157141818, 0.3187964583157141818, 0.3333333333333333703),
 ( 0.3333333333333333703, 0.3187964583157141818, 0.3187964583157141818, 0.3333333333333333703),
 ( 1.000000000000000000, 0.9563893749471424899, 0.9563893749471424899, 1.000000000000000000) ) ) 
 REPRESENTATION_ITEM ( '' )  SURFACE ( )  );
#36307=CARTESIAN_POINT ( 'NONE',  ( 27.31903677934867147, 0.4900422023718347675, -5.740875207198388175 ) ) ;
#36310=CARTESIAN_POINT ( 'NONE',  ( -80.68111603624291206, -5.697143737140332398, 2.247291075986532771 ) ) ;
#36311=CARTESIAN_POINT ( 'NONE',  ( 26.76128115921286721, 0.8698978912984448586, -4.383280502865230410 ) ) ;
#36312=ADVANCED_FACE ( 'NONE', ( #28456 ), #37506, .T. ) ;
#36314=PLANE ( 'NONE',  #11224 ) ;
#36317=CARTESIAN_POINT ( 'NONE',  ( 33.94448162299985938, -0.4909416048696789159, -5.125106431712468158 ) ) ;
#36331=CARTESIAN_POINT ( 'NONE',  ( 85.00114435706898064, 2.071954908684588759, 4.651167869591634307 ) ) ;
#36338=CARTESIAN_POINT ( 'NONE',  ( 33.89725028478159174, -5.465908938576614418, 0.4877600842561391481 ) ) ;
#36344=CARTESIAN_POINT ( 'NONE',  ( 17.62552264067466012, 11.92971595993793699, -2.499999999999990230 ) ) ;
#36352=CARTESIAN_POINT ( 'NONE',  ( 21.85643539959774273, 10.54442680926682208, -0.8960936389291185300 ) ) ;
#36354=CARTESIAN_POINT ( 'NONE',  ( -80.70058103876492339, 10.56056044066735389, 2.265492480125265828 ) ) ;
#36357=CARTESIAN_POINT ( 'NONE',  ( 14.72816174088550412, -4.874090160042384490, 2.502238201714006571 ) ) ;
#36359=CARTESIAN_POINT ( 'NONE',  ( -79.68352313332665915, 11.50554291592259304, -4.849210015756803216 ) ) ;
#36367=CARTESIAN_POINT ( 'NONE',  ( 87.84483433992669177, -0.3137627012552636763, 3.545048087552764571 ) ) ;
#36370=CARTESIAN_POINT ( 'NONE',  ( 37.04660275223199761, -2.800648277598226876, 5.988416353595834352 ) ) ;
#36373=CARTESIAN_POINT ( 'NONE',  ( 86.79297523138272652, 0.7501027249346864378, -5.742269118526623473 ) ) ;
#36386=CARTESIAN_POINT ( 'NONE',  ( 21.76373982720479461, 0.8608337276742248356, 7.726924402482800325 ) ) ;
#36392=CARTESIAN_POINT ( 'NONE',  ( 37.83867290611771494, -6.084034091406928191, -6.000000000000000000 ) ) ;
#36397=CARTESIAN_POINT ( 'NONE',  ( 23.89311878034035530, 3.219763706263101266, -3.577746201333754428 ) ) ;
#36401=CARTESIAN_POINT ( 'NONE',  ( 22.67874324181232737, -4.030091496876125667, 7.802482278901700319 ) ) ;
#36406=CARTESIAN_POINT ( 'NONE',  ( 85.64278173364962754, 1.868356560669967470, -5.099220668941490509 ) ) ;
#36411=CARTESIAN_POINT ( 'NONE',  ( 16.03358042430196306, -3.427093395206350479, -2.707976865299952518 ) ) ;
#36412=CARTESIAN_POINT ( 'NONE',  ( 27.40617277722898493, 0.9610190317717227648, -4.483794101316670222 ) ) ;
#36413=DIRECTION ( 'NONE',  ( -0.000000000000000000, -1.000000000000000000, -0.000000000000000000 ) ) ;
#36414=CARTESIAN_POINT ( 'NONE',  ( 27.16624160081412853, 1.269200517689503593, -4.441067823234377876 ) ) ;
#36417=CARTESIAN_POINT ( 'NONE',  ( 36.89667292320353198, -3.000775245577192329, 5.965016177709391521 ) ) ;
#36418=VECTOR ( 'NONE', #30872, 1000.000000000000000 ) ;
#36423=CARTESIAN_POINT ( 'NONE',  ( 37.00899628427189469, -3.246980710513998947, 5.946852153544761599 ) ) ;
#36425=CARTESIAN_POINT ( 'NONE',  ( 17.66378170928452818, -3.205320407151504902, -2.924525624963761672 ) ) ;
#36427=ORIENTED_EDGE ( 'NONE', *, *, #3853, .T. ) ;
#36428=PLANE ( 'NONE',  #33890 ) ;
#36429=VECTOR ( 'NONE', #38345, 1000.000000000000000 ) ;
#36435=CARTESIAN_POINT ( 'NONE',  ( 14.77222197358542033, -4.491748702149269690, 2.511961485181798626 ) ) ;
#36447=CARTESIAN_POINT ( 'NONE',  ( 24.83382150147336986, 2.575822499426965617, -3.953843410308002237 ) ) ;
#36449=DIRECTION ( 'NONE',  ( -0.000000000000000000, -0.000000000000000000, -1.000000000000000000 ) ) ;
#36455=CARTESIAN_POINT ( 'NONE',  ( 87.97568001472090771, -0.4607347734944167716, -3.153239710520575390 ) ) ;
#36456=CARTESIAN_POINT ( 'NONE',  ( 29.20850709934801159, 2.242166301403143880, -0.5075834600922535245 ) ) ;
#36458=CARTESIAN_POINT ( 'NONE',  ( -72.87804133339554369, 1.626223713339684629, -10.95881965187203377 ) ) ;
#36459=CARTESIAN_POINT ( 'NONE',  ( 33.12434724996504798, -3.753162291981519516, 5.124365322589720328 ) ) ;
#36461=CARTESIAN_POINT ( 'NONE',  ( 33.68123845448776166, -3.186000923572973154, -5.463169863251220448 ) ) ;
#36468=VERTEX_POINT ( 'NONE', #5824 ) ;
#36469=CARTESIAN_POINT ( 'NONE',  ( 23.34994303252841163, 3.524623506009445961, 3.233127816796116605 ) ) ;
#36474=CARTESIAN_POINT ( 'NONE',  ( -71.92837670882107659, -0.6507271787433660526, 9.949874371066202983 ) ) ;
#36481=CARTESIAN_POINT ( 'NONE',  ( 84.98973554254388318, 1.887807287779055709, -4.881612716162457843 ) ) ;
#36482=CARTESIAN_POINT ( 'NONE',  ( -77.50518483875032416, 11.08526101523151475, 7.544008514241666852 ) ) ;
#36488=CARTESIAN_POINT ( 'NONE',  ( 24.75344691226916893, 3.017249892964377622, 3.359965021756160741 ) ) ;
#36491=EDGE_CURVE ( 'NONE', #14346, #23464, #10113, .T. ) ;
#36494=EDGE_LOOP ( 'NONE', ( #30262, #33099, #24622, #5013 ) ) ;
#36496=CARTESIAN_POINT ( 'NONE',  ( 22.60277826478245800, 0.2789680342660347256, 6.515017021779732964 ) ) ;
#36501=ADVANCED_FACE ( 'NONE', ( #22503 ), #28867, .T. ) ;
#36503=DIRECTION ( 'NONE',  ( 1.000000000000000000, 0.000000000000000000, 0.000000000000000000 ) ) ;
#36504=CARTESIAN_POINT ( 'NONE',  ( 63.05383694556373797, -7.271989087314214117, -6.000000000000000000 ) ) ;
#36505=CARTESIAN_POINT ( 'NONE',  ( 27.77988552260176291, -0.3358138158918914651, -6.029166980063449088 ) ) ;
#36508=EDGE_LOOP ( 'NONE', ( #34867, #39357 ) ) ;
#36510=CARTESIAN_POINT ( 'NONE',  ( 21.78348496727135952, 0.2136468579297728376, -8.398162227918549050 ) ) ;
#36516=CARTESIAN_POINT ( 'NONE',  ( -70.92837670882107659, -48.61702805680358352, 10.00000000000000888 ) ) ;
#36517=CARTESIAN_POINT ( 'NONE',  ( 37.17584199213645491, -2.565478455631990951, -5.981118737177594014 ) ) ;
#36537=FACE_BOUND ( 'NONE', #12800, .T. ) ;
#36542=VECTOR ( 'NONE', #31130, 1000.000000000000000 ) ;
#36547=CARTESIAN_POINT ( 'NONE',  ( 22.14454166288778580, 4.578504518513106802, 3.662589312894346083 ) ) ;
#36549=CARTESIAN_POINT ( 'NONE',  ( 20.40287464734031531, 10.75613383782063970, 2.500000000000000000 ) ) ;
#36550=CARTESIAN_POINT ( 'NONE',  ( 21.85643539959780313, 0.4758835581198413989, -14.20546615820951963 ) ) ;
#36552=CARTESIAN_POINT ( 'NONE',  ( -77.86968774964118722, 9.956382404624021021, 7.211963008493430749 ) ) ;
#36554=CARTESIAN_POINT ( 'NONE',  ( -80.20198641814972973, 10.53012318711579454, -3.762333814409368760 ) ) ;
#36558=CARTESIAN_POINT ( 'NONE',  ( 14.76778848929227372, 12.79472506199442172, 2.506269218290250400 ) ) ;
#36568=CARTESIAN_POINT ( 'NONE',  ( 36.89767088514894056, -3.003071912148901568, 5.965171933806773019 ) ) ;
#36572=CARTESIAN_POINT ( 'NONE',  ( 86.63338141420044280, 0.5786414684654883622, -5.958757720264261870 ) ) ;
#36576=CARTESIAN_POINT ( 'NONE',  ( 31.50304906168603125, -0.4789496544865932681, -5.123210728833553773 ) ) ;
#36580=DIRECTION ( 'NONE',  ( 1.000000000000000000, 0.000000000000000000, 0.000000000000000000 ) ) ;
#36582=VERTEX_POINT ( 'NONE', #28667 ) ;
#36584=PRODUCT_DEFINITION_CONTEXT ( 'detailed design', #6089, 'design' ) ;
#36586=ORIENTED_EDGE ( 'NONE', *, *, #32509, .T. ) ;
#36591=CARTESIAN_POINT ( 'NONE',  ( 22.41436559212412760, 0.3887359917284659017, 6.830184646630694800 ) ) ;
#36598=CARTESIAN_POINT ( 'NONE',  ( -62.92837670882107659, -49.49506129533733656, 6.000000000000000000 ) ) ;
#36600=CARTESIAN_POINT ( 'NONE',  ( 22.42542530853210181, 4.782089792738570821, -3.164282654266882933 ) ) ;
#36604=CARTESIAN_POINT ( 'NONE',  ( 22.31703049540045924, 6.264542857755036387, 0.009563241200241559548 ) ) ;
#36608=CARTESIAN_POINT ( 'NONE',  ( 84.43092178082896737, 2.949567725576020649, 1.921192885956162444 ) ) ;
#36611=CARTESIAN_POINT ( 'NONE',  ( 23.03318261145397017, 4.443153149067368801, -2.273821518518992502 ) ) ;
#36612=CARTESIAN_POINT ( 'NONE',  ( 16.07587011183210635, -3.522579363632067917, -2.698830145762970645 ) ) ;
#36613=CARTESIAN_POINT ( 'NONE',  ( 36.19300506522036187, -2.234529143593806388, -5.855191790199620883 ) ) ;
#36615=CARTESIAN_POINT ( 'NONE',  ( 27.07499125159621300, 1.335026952719597926, -4.423825550918643934 ) ) ;
#36618=CARTESIAN_POINT ( 'NONE',  ( 33.68750564893161936, -3.098785954741594573, 5.464148010559176427 ) ) ;
#36619=CARTESIAN_POINT ( 'NONE',  ( 85.39749695915146788, 2.435202802470831873, -2.633776547657810774 ) ) ;
#36620=ORIENTED_EDGE ( 'NONE', *, *, #17362, .T. ) ;
#36623=CARTESIAN_POINT ( 'NONE',  ( 32.07039327229519898, 0.2549240838516523278, 4.723724623685981783 ) ) ;
#36624=CARTESIAN_POINT ( 'NONE',  ( -69.42837670882107659, -47.31299788476771084, 9.886859966642605357 ) ) ;
#36625=CARTESIAN_POINT ( 'NONE',  ( 21.09191007886703062, -3.054293775446101478, -3.415671279545484218 ) ) ;
#36628=ADVANCED_FACE ( 'NONE', ( #20387 ), #5364, .F. ) ;
#36640=DIRECTION ( 'NONE',  ( -0.000000000000000000, 1.000000000000000000, -0.000000000000000000 ) ) ;
#36642=CARTESIAN_POINT ( 'NONE',  ( 21.83430649484399311, 4.714758532028221261, 3.915150708602226359 ) ) ;
#36647=CARTESIAN_POINT ( 'NONE',  ( 22.13428935428179400, -2.652497287587405772, -3.660989192183361052 ) ) ;
#36650=CARTESIAN_POINT ( 'NONE',  ( 24.31786857884458541, 2.722531517372515975, -3.914669340711137036 ) ) ;
#36652=CARTESIAN_POINT ( 'NONE',  ( -4.444218661349752963, -35.94265729135299381, 6.000000000000000000 ) ) ;
#36657=CARTESIAN_POINT ( 'NONE',  ( 87.36631219772915813, 0.2237360808920199895, 4.554730944530843040 ) ) ;
#36658=CARTESIAN_POINT ( 'NONE',  ( 29.43591252028664584, 1.494051637964393553, 3.776330930280134002 ) ) ;
#36661=CARTESIAN_POINT ( 'NONE',  ( 16.28057921272570496, -3.484615921975166231, 2.724815388562823681 ) ) ;
#36663=CARTESIAN_POINT ( 'NONE',  ( 36.90757751090616523, -3.026075607118911215, -5.966718102348832709 ) ) ;
#36669=CARTESIAN_POINT ( 'NONE',  ( 36.39216306811729851, -1.827485476554924437, 5.788500282070289771 ) ) ;
#36670=AXIS2_PLACEMENT_3D ( 'NONE', #25471, #6332, #34562 ) ;
#36678=EDGE_CURVE ( 'NONE', #36582, #36858, #26811, .T. ) ;
#36680=CARTESIAN_POINT ( 'NONE',  ( -74.39026271145056057, 9.085113976877558173, 9.386028689943199055 ) ) ;
#36688=CARTESIAN_POINT ( 'NONE',  ( 21.99269358992065193, 5.592676286834311838, 3.104126389907300165 ) ) ;
#36691=CARTESIAN_POINT ( 'NONE',  ( 23.40522682912259000, 3.763699709236936641, -3.087242233077766684 ) ) ;
#36694=CARTESIAN_POINT ( 'NONE',  ( 24.74480270654332514, 0.5641214079007167426, 4.778945666302679030 ) ) ;
#36695=CARTESIAN_POINT ( 'NONE',  ( 14.74076604532273294, -4.695325025251882778, -2.506186015952889701 ) ) ;
#36698=CARTESIAN_POINT ( 'NONE',  ( 36.27994091153181699, -3.621545396486653967, -5.740730168913134257 ) ) ;
#36699=ORIENTED_EDGE ( 'NONE', *, *, #12365, .T. ) ;
#36702=CARTESIAN_POINT ( 'NONE',  ( 59.69572451838116933, -0.8894979772356270686, -6.000000000000000000 ) ) ;
#36704=CARTESIAN_POINT ( 'NONE',  ( 29.67594332454466866, -2.985454744488035494, -5.114964129314456542 ) ) ;
#36706=CARTESIAN_POINT ( 'NONE',  ( 14.77500326541903952, -5.175625724643098557, -2.499997102511863911 ) ) ;
#36714=CARTESIAN_POINT ( 'NONE',  ( 33.68467625662385956, -3.836896542393491316, -5.141322647849833061 ) ) ;
#36725=ORIENTED_EDGE ( 'NONE', *, *, #26787, .T. ) ;
#36731=AXIS2_PLACEMENT_3D ( 'NONE', #20653, #23942, #39808 ) ;
#36733=EDGE_CURVE ( 'NONE', #22987, #13150, #17974, .T. ) ;
#36743=CARTESIAN_POINT ( 'NONE',  ( 16.70600443586730677, 9.848044269046425825, -2.499999999999896083 ) ) ;
#36749=DIRECTION ( 'NONE',  ( 1.000000000000000000, 0.000000000000000000, -0.000000000000000000 ) ) ;
#36752=CARTESIAN_POINT ( 'NONE',  ( 21.85643539959777115, -1.469530054879572223, 14.38030055974112464 ) ) ;
#36754=CARTESIAN_POINT ( 'NONE',  ( -78.60822725968512259, 10.22187107137118289, 6.417182048864131794 ) ) ;
#36755=CARTESIAN_POINT ( 'NONE',  ( 14.70646227107939907, -5.038312110033563052, 2.499999999999891198 ) ) ;
#36756=CARTESIAN_POINT ( 'NONE',  ( -75.81783553891371241, 10.25601890356784907, -8.731154437199055707 ) ) ;
#36757=AXIS2_PLACEMENT_3D ( 'NONE', #14974, #33728, #8781 ) ;
#36759=CARTESIAN_POINT ( 'NONE',  ( 33.45683418328554382, -3.835186817697033845, -5.087345507474531736 ) ) ;
#36761=CARTESIAN_POINT ( 'NONE',  ( 14.76957396737453365, 12.55251976517217116, 2.511547239741789284 ) ) ;
#36765=ADVANCED_FACE ( 'NONE', ( #1890 ), #11516, .F. ) ;
#36769=CARTESIAN_POINT ( 'NONE',  ( 87.03857031557907931, 0.5918713184910167069, 4.894172095624758079 ) ) ;
#36771=ORIENTED_EDGE ( 'NONE', *, *, #33408, .T. ) ;
#36773=CARTESIAN_POINT ( 'NONE',  ( 36.92993436146343811, -2.615930867933358162, 5.970207429580749903 ) ) ;
#36776=CARTESIAN_POINT ( 'NONE',  ( 84.80723110164849743, 2.854080505324299466, 2.680610459220619912 ) ) ;
#36777=CARTESIAN_POINT ( 'NONE',  ( -71.90214061647091626, -21.04549931135898078, 5.920672442023850124 ) ) ;
#36781=CARTESIAN_POINT ( 'NONE',  ( 86.46043323462474461, 1.241262327860113590, 4.894917242394325463 ) ) ;
#36782=CARTESIAN_POINT ( 'NONE',  ( -70.31369189463936209, -21.58244653382578448, 5.969151678864092148 ) ) ;
#36790=CARTESIAN_POINT ( 'NONE',  ( 22.39383066815476298, 0.3445199978907897975, 6.891788138977129385 ) ) ;
#36792=ORIENTED_EDGE ( 'NONE', *, *, #5758, .T. ) ;
#36800=CARTESIAN_POINT ( 'NONE',  ( 24.02597498973994306, 3.319991383958946329, -3.315850951064452268 ) ) ;
#36803=ADVANCED_FACE ( 'NONE', ( #14010 ), #22183, .T. ) ;
#36805=CARTESIAN_POINT ( 'NONE',  ( 25.51884215448320958, -4.718317418738882552, 0.4603789867971156413 ) ) ;
#36806=ADVANCED_FACE ( 'NONE', ( #12915 ), #21019, .T. ) ;
#36810=CARTESIAN_POINT ( 'NONE',  ( 85.73014479007146349, 1.298542115207370173, 5.666065989068760800 ) ) ;
#36811=CARTESIAN_POINT ( 'NONE',  ( 16.14955235345561846, 10.48078119528741681, 2.684236915963923220 ) ) ;
#36814=EDGE_CURVE ( 'NONE', #22023, #24696, #20900, .T. ) ;
#36817=CARTESIAN_POINT ( 'NONE',  ( 28.89703635215781574, -3.425538172464888564, -4.559836211139066009 ) ) ;
#36819=CARTESIAN_POINT ( 'NONE',  ( -69.92837670882107659, -20.78299143688747819, 38.00000000000000711 ) ) ;
#36822=CARTESIAN_POINT ( 'NONE',  ( 25.29476808408737654, 1.731675346697265860, 4.154258334436543798 ) ) ;
#36825=CARTESIAN_POINT ( 'NONE',  ( 85.27007178914716690, 2.578332801382848594, -1.917248250713118773 ) ) ;
#36829=CARTESIAN_POINT ( 'NONE',  ( 29.48942925047375141, 1.221239797401782567, 4.218574441359598914 ) ) ;
#36830=CARTESIAN_POINT ( 'NONE',  ( 17.26834050228787731, -3.265917822029717144, -2.867547815643560760 ) ) ;
#36831=CARTESIAN_POINT ( 'NONE',  ( 14.77315594796473874, 13.19392823276514015, -2.499999999999998668 ) ) ;
#36834=CARTESIAN_POINT ( 'NONE',  ( -61.24591834330252027, 10.37661300689600097, 2.500000000000000000 ) ) ;
#36842=CARTESIAN_POINT ( 'NONE',  ( 21.85777359310080570, 3.445828482919746527, 4.744213995278264484 ) ) ;
#36849=CYLINDRICAL_SURFACE ( 'NONE', #18675, 6.000000000000002665 ) ;
#36850=CARTESIAN_POINT ( 'NONE',  ( 22.15490704303159930, -2.652577471374245377, -3.664207081153456169 ) ) ;
#36853=CARTESIAN_POINT ( 'NONE',  ( 22.03798447844329189, 3.618149687637631562, -4.432112028060099185 ) ) ;
#36854=ORIENTED_EDGE ( 'NONE', *, *, #5099, .T. ) ;
#36856=CARTESIAN_POINT ( 'NONE',  ( 21.85643539959779247, -15.31483402087699197, 0.9306824932977513232 ) ) ;
#36857=LINE ( 'NONE', #8433, #9161 ) ;
#36858=VERTEX_POINT ( 'NONE', #27791 ) ;
#36860=CARTESIAN_POINT ( 'NONE',  ( 86.31714526353648864, 1.402210177843808081, 5.108895447378689170 ) ) ;
#36861=CARTESIAN_POINT ( 'NONE',  ( -62.92837670882107659, -49.49506129533733656, -6.000000000000000000 ) ) ;
#36867=CARTESIAN_POINT ( 'NONE',  ( 21.53366635609027213, -3.014980951220062266, 3.494836103679133998 ) ) ;
#36870=CARTESIAN_POINT ( 'NONE',  ( 36.19480630455252168, -2.230552841105437611, -5.855472917160542856 ) ) ;
#36875=CARTESIAN_POINT ( 'NONE',  ( -70.53399048836877228, -45.65663887815897937, 5.989775712723940160 ) ) ;
#36878=CARTESIAN_POINT ( 'NONE',  ( 36.07741663790258002, -1.633014503204270218, 5.715722609253349518 ) ) ;
#36884=LINE ( 'NONE', #21454, #39046 ) ;
#36885=CARTESIAN_POINT ( 'NONE',  ( -72.37610296055093784, -1.106069955589489284, -9.901772949365062360 ) ) ;
#36890=DIRECTION ( 'NONE',  ( -0.000000000000000000, -1.000000000000000000, -0.000000000000000000 ) ) ;
#36892=ORIENTED_EDGE ( 'NONE', *, *, #628, .F. ) ;
#36893=CARTESIAN_POINT ( 'NONE',  ( 23.14097115081952438, 4.021047326275176026, 3.125729442354085119 ) ) ;
#36901=CARTESIAN_POINT ( 'NONE',  ( 24.12183659247549627, 0.4863356266236299463, 5.096531192340497896 ) ) ;
#36906=VERTEX_POINT ( 'NONE', #8848 ) ;
#36907=CARTESIAN_POINT ( 'NONE',  ( 35.35377756119452641, -3.785667184757509407, -5.510616941430652282 ) ) ;
#36909=PLANE ( 'NONE',  #24403 ) ;
#36911=B_SPLINE_CURVE_WITH_KNOTS ( 'NONE', 3,
 ( #4429, #13268, #20057, #4034, #10382, #38783, #38176, #25838, #16955, #38577 ),
 .UNSPECIFIED., .F., .F.,
 ( 4, 2, 2, 2, 4 ),
 ( 0.000000000000000000, 0.2500000000000000000, 0.5000000000000000000, 0.7500000000000000000, 1.000000000000000000 ),
 .UNSPECIFIED. ) ;
#36912=CARTESIAN_POINT ( 'NONE',  ( 30.36459403182758265, -1.672762201151555939, 6.017704416797944766 ) ) ;
#36913=CARTESIAN_POINT ( 'NONE',  ( 14.67669714044831153, -4.948475139782464893, -2.499999999999940492 ) ) ;
#36914=LINE ( 'NONE', #27039, #12790 ) ;
#36916=CARTESIAN_POINT ( 'NONE',  ( 26.00522225989622171, 0.8586799828388421707, -4.425729458961279228 ) ) ;
#36923=CARTESIAN_POINT ( 'NONE',  ( 36.82367268480642508, -2.161198714638147056, -5.895793440235796545 ) ) ;
#36929=CARTESIAN_POINT ( 'NONE',  ( -75.12005306888337941, 8.050441697125293672, 10.43857059077842564 ) ) ;
#36940=LINE ( 'NONE', #27671, #9590 ) ;
#36946=CARTESIAN_POINT ( 'NONE',  ( 22.61730376708971235, 4.636646153475214582, 3.020898913531409935 ) ) ;
#36948=EDGE_CURVE ( 'NONE', #24169, #12496, #5780, .T. ) ;
#36951=CARTESIAN_POINT ( 'NONE',  ( 16.54830220824161913, 9.917958018445570900, -2.500000000000029754 ) ) ;
#36957=CARTESIAN_POINT ( 'NONE',  ( 21.85643539959780313, 0.1435845899245215551, -12.62009698158557747 ) ) ;
#36959=CARTESIAN_POINT ( 'NONE',  ( -80.19290758530635799, 10.52933779828717853, 3.784726273488611348 ) ) ;
#36960=CARTESIAN_POINT ( 'NONE',  ( 36.75962662137767722, -3.428235495735559635, 5.873601727554911278 ) ) ;
#36962=CARTESIAN_POINT ( 'NONE',  ( -76.84822446654321482, 9.441555170962290688, -8.079216459568250741 ) ) ;
#36965=CARTESIAN_POINT ( 'NONE',  ( 36.20134656968558318, -3.653170093647291949, -5.716499845661110690 ) ) ;
#36967=CARTESIAN_POINT ( 'NONE',  ( 14.80429365997629176, 12.91757655414798300, 2.502880492504405030 ) ) ;
#36972=CARTESIAN_POINT ( 'NONE',  ( 17.06903337278474808, 14.51719371156824501, -2.500000000000000444 ) ) ;
#36974=CARTESIAN_POINT ( 'NONE',  ( 25.83720352597168102, 2.054051280725787354, -4.175065982317311963 ) ) ;
#36975=VERTEX_POINT ( 'NONE', #25884 ) ;
#36977=CARTESIAN_POINT ( 'NONE',  ( 36.49083949649433833, -2.266323086343007276, 5.901676056353022837 ) ) ;
#36980=CARTESIAN_POINT ( 'NONE',  ( 87.43313723349395161, -0.009410480739497543642, 5.495402557179364322 ) ) ;
#36981=CARTESIAN_POINT ( 'NONE',  ( 33.55312825858863590, -1.200935527647059020, -5.443175168862945057 ) ) ;
#37003=CARTESIAN_POINT ( 'NONE',  ( 22.89069174712559374, 4.265217579236236567, -3.147968593956119054 ) ) ;
#37010=CARTESIAN_POINT ( 'NONE',  ( 84.65562454054800412, 2.508334066475362167, -3.654169056841765517 ) ) ;
#37017=CARTESIAN_POINT ( 'NONE',  ( 14.81281001777914064, -4.468420226103234860, -2.515823251450710174 ) ) ;
#37022=CARTESIAN_POINT ( 'NONE',  ( 88.37152744968734908, -0.9053694005015545665, 0.1944390934057901588 ) ) ;
#37026=CARTESIAN_POINT ( 'NONE',  ( 37.21265578649057204, -2.743522425390099162, 6.000894410541715907 ) ) ;
#37027=CARTESIAN_POINT ( 'NONE',  ( 17.69217577633630967, -2.919086151025220843, 2.967689935422107794 ) ) ;
#37029=FACE_OUTER_BOUND ( 'NONE', #15209, .T. ) ;
#37040=CARTESIAN_POINT ( 'NONE',  ( 22.47157634915228996, 2.831433730378157154, 4.675524411331370089 ) ) ;
#37041=CARTESIAN_POINT ( 'NONE',  ( 14.74978830686079156, 12.47633826711515681, 2.508459208900589044 ) ) ;
#37043=ADVANCED_FACE ( 'NONE', ( #23396 ), #26491, .F. ) ;
#37048=CARTESIAN_POINT ( 'NONE',  ( 85.17069404690863621, 2.689958598217443875, -0.9157604595814767823 ) ) ;
#37051=CARTESIAN_POINT ( 'NONE',  ( 24.38698540644270807, 2.853369664508251358, -3.808177377505154837 ) ) ;
#37053=CARTESIAN_POINT ( 'NONE',  ( 21.85643539959778892, 9.726370091839324772, -5.619754257929120200 ) ) ;
#37058=CARTESIAN_POINT ( 'NONE',  ( 85.75411537215676105, 2.034632074852215311, 4.270953678727185121 ) ) ;
#37063=CARTESIAN_POINT ( 'NONE',  ( -70.92837670882107659, -65.19654454972992141, 6.000000000000002665 ) ) ;
#37064=CARTESIAN_POINT ( 'NONE',  ( 37.04632708303561373, -2.800829925423356404, -5.988373328750657087 ) ) ;
#37066=CARTESIAN_POINT ( 'NONE',  ( 25.01091298175105848, 3.329590532566609529, -1.936828115965013142 ) ) ;
#37072=CARTESIAN_POINT ( 'NONE',  ( 35.16091957826717618, -1.161011098338289749, 5.517918506450993910 ) ) ;
#37075=EDGE_CURVE ( 'NONE', #18960, #14346, #30020, .T. ) ;
#37076=CARTESIAN_POINT ( 'NONE',  ( -71.80181757295153488, -0.2787158081064600723, 9.961909801952202770 ) ) ;
#37082=CARTESIAN_POINT ( 'NONE',  ( 20.58590956074638711, 5.855084980973656705, 3.419327077695344386 ) ) ;
#37089=CARTESIAN_POINT ( 'NONE',  ( 22.02370413983413044, 5.453436713694586935, 3.173045162501021643 ) ) ;
#37090=EDGE_CURVE ( 'NONE', #20369, #13284, #4475, .T. ) ;
#37099=CARTESIAN_POINT ( 'NONE',  ( 14.72162123416106638, -5.034119505677589146, -2.499999999996632916 ) ) ;
#37108=DIRECTION ( 'NONE',  ( 1.000000000000000000, 0.000000000000000000, -0.000000000000000000 ) ) ;
#37110=CARTESIAN_POINT ( 'NONE',  ( 31.06145916124171436, -2.509195271462365540, -5.777646538787225339 ) ) ;
#37114=DIRECTION ( 'NONE',  ( 1.165409145176969993E-16, -1.000000000000000000, 0.000000000000000000 ) ) ;
#37119=CARTESIAN_POINT ( 'NONE',  ( 37.06799344668426954, -2.451880675787394992, -5.964061398877268161 ) ) ;
#37120=CARTESIAN_POINT ( 'NONE',  ( 30.88954940396924087, -3.454941690857903591, -4.920487672143777580 ) ) ;
#37128=CARTESIAN_POINT ( 'NONE',  ( 21.33769325710290943, 8.396068077058080448, 2.669439336573398158 ) ) ;
#37129=CARTESIAN_POINT ( 'NONE',  ( 23.09544648813622914, 1.703250674360487382, -5.094339560058331884 ) ) ;
#37130=EDGE_LOOP ( 'NONE', ( #38671, #15283, #5961, #35943 ) ) ;
#37135=CARTESIAN_POINT ( 'NONE',  ( -0.7996099067669091287, -29.56993018339339940, -6.000000000000000000 ) ) ;
#37144=CARTESIAN_POINT ( 'NONE',  ( 23.14717476177426647, 4.059201937619430822, 3.048413602859032512 ) ) ;
#37153=CIRCLE ( 'NONE', #16122, 12.38600677260393113 ) ;
#37158=CARTESIAN_POINT ( 'NONE',  ( 21.85643539959778892, -9.157157878381195104, -8.039778668638760450 ) ) ;
#37159=ORIENTED_EDGE ( 'NONE', *, *, #36491, .T. ) ;
#37160=CARTESIAN_POINT ( 'NONE',  ( -77.38833691583745633, 11.04400030039685277, 7.643251527845681181 ) ) ;
#37166=CARTESIAN_POINT ( 'NONE',  ( 23.38716521561124750, 3.561324528878642592, -3.087505459527394081 ) ) ;
#37168=CARTESIAN_POINT ( 'NONE',  ( 14.78431785254804431, 13.03024247939681679, 2.500601908585387001 ) ) ;
#37172=CARTESIAN_POINT ( 'NONE',  ( 17.27696687802587050, 14.34575037107839890, -2.499999999999999556 ) ) ;
#37173=CARTESIAN_POINT ( 'NONE',  ( 31.94853774039595251, -3.766211141015790353, -4.792495538025669077 ) ) ;
#37174=CARTESIAN_POINT ( 'NONE',  ( 24.56779495282315651, 2.976875296945072691, -3.585541128247576648 ) ) ;
#37177=CARTESIAN_POINT ( 'NONE',  ( 36.15903063279257879, -3.359981914139457793, 5.843280261744577153 ) ) ;
#37181=CARTESIAN_POINT ( 'NONE',  ( 87.54376689718995408, -0.1385995495200708916, -5.388168202639758597 ) ) ;
#37182=CARTESIAN_POINT ( 'NONE',  ( 29.20850709934801159, 2.242166301403143880, -0.5075834600922535245 ) ) ;
#37185=CARTESIAN_POINT ( 'NONE',  ( 24.50840889722684324, 2.969483997251146867, 3.629079860099836186 ) ) ;
#37190=ADVANCED_FACE ( 'NONE', ( #584 ), #26093, .F. ) ;
#37195=CARTESIAN_POINT ( 'NONE',  ( 14.61802081865033820, 12.33286846116140190, 2.500000000000000000 ) ) ;
#37202=DIRECTION ( 'NONE',  ( 1.000000000000000000, 0.000000000000000000, 0.000000000000000000 ) ) ;
#37204=CARTESIAN_POINT ( 'NONE',  ( 21.73142018617180682, 6.152679399380986069, -3.256810401554945056 ) ) ;
#37208=AXIS2_PLACEMENT_3D ( 'NONE', #14394, #1663, #32952 ) ;
#37212=CARTESIAN_POINT ( 'NONE',  ( 86.96369117609759769, -0.5876503451053297633, 5.665127693518188678 ) ) ;
#37213=CARTESIAN_POINT ( 'NONE',  ( 20.34593195197777149, 6.625392312321536359, 3.270953163479469961 ) ) ;
#37220=CARTESIAN_POINT ( 'NONE',  ( -70.92837670882107659, -56.35932253828836025, 10.00000000000000888 ) ) ;
#37221=CARTESIAN_POINT ( 'NONE',  ( 14.91073189335287807, -5.916690698649474278, -2.519298049349560475 ) ) ;
#37225=CARTESIAN_POINT ( 'NONE',  ( 36.64525587059520717, -2.463007710373897652, 5.925776466105311613 ) ) ;
#37232=CARTESIAN_POINT ( 'NONE',  ( 14.69558838330741857, 12.33286846116280699, -2.500000000000005773 ) ) ;
#37237=VERTEX_POINT ( 'NONE', #7939 ) ;
#37244=CARTESIAN_POINT ( 'NONE',  ( 24.06991255396462392, 2.373183232073612370, 4.210890719218481237 ) ) ;
#37245=CARTESIAN_POINT ( 'NONE',  ( 31.44497614105462446, 0.4838685039436804169, 4.609055630922440194 ) ) ;
#37247=AXIS2_PLACEMENT_3D ( 'NONE', #36652, #36449, #7838 ) ;
#37256=CARTESIAN_POINT ( 'NONE',  ( 23.28996408820413322, 3.028860784884633173, -4.014842745608873997 ) ) ;
#37259=CARTESIAN_POINT ( 'NONE',  ( 21.85643539959773207, -2.491245572580281564, -14.29094192267194607 ) ) ;
#37263=CARTESIAN_POINT ( 'NONE',  ( 87.56526962053540331, 0.0002576605070852033049, 4.866394609412610706 ) ) ;
#37267=CARTESIAN_POINT ( 'NONE',  ( 33.11504244789421136, -3.652289920775848131, 5.213393308200740428 ) ) ;
#37269=CARTESIAN_POINT ( 'NONE',  ( 30.51714320403715419, -0.1346950231246703544, -4.969336275524192104 ) ) ;
#37272=ADVANCED_FACE ( 'NONE', ( #8335 ), #22524, .T. ) ;
#37275=ORIENTED_EDGE ( 'NONE', *, *, #17140, .F. ) ;
#37277=VECTOR ( 'NONE', #40212, 1000.000000000000000 ) ;
#37279=CARTESIAN_POINT ( 'NONE',  ( 21.78047233922835346, 5.616103166486084319, -3.473245622192032034 ) ) ;
#37282=CARTESIAN_POINT ( 'NONE',  ( 21.67022320682240988, 4.173608297239179699, 3.080183978364538611 ) ) ;
#37287=CARTESIAN_POINT ( 'NONE',  ( 88.29941837874866906, -0.8243730695201928471, 1.365802595430977151 ) ) ;
#37288=CARTESIAN_POINT ( 'NONE',  ( -78.41777952335573332, -6.504124592832953411, -6.677813406577614685 ) ) ;
#37294=CARTESIAN_POINT ( 'NONE',  ( 24.70642277111918617, 3.001709267698361661, 3.438663434477700065 ) ) ;
#37300=CARTESIAN_POINT ( 'NONE',  ( -12.99139449055068241, 13.37661300689600097, -6.000000000000000000 ) ) ;
#37312=CARTESIAN_POINT ( 'NONE',  ( 31.90185279284946773, -4.312872639525808793, -3.838359570106229413 ) ) ;
#37313=CARTESIAN_POINT ( 'NONE',  ( 0.000000000000000000, 10.37661300689600097, 6.000000000000000000 ) ) ;
#37316=CARTESIAN_POINT ( 'NONE',  ( 21.78989781213234167, 0.2240611524379590713, -8.363397281163468477 ) ) ;
#37318=FACE_OUTER_BOUND ( 'NONE', #2454, .T. ) ;
#37323=CARTESIAN_POINT ( 'NONE',  ( 36.69958409632433671, -3.382823349610835972, -5.888586716072319760 ) ) ;
#37332=VECTOR ( 'NONE', #35671, 1000.000000000000000 ) ;
#37333=CARTESIAN_POINT ( 'NONE',  ( 14.77094618574839302, -5.164039144567283302, -2.500001188512491090 ) ) ;
#37337=AXIS2_PLACEMENT_3D ( 'NONE', #15788, #28340, #1560 ) ;
#37346=CARTESIAN_POINT ( 'NONE',  ( 22.88200939092931208, 4.346293566238504269, 3.037513980216376641 ) ) ;
#37358=CARTESIAN_POINT ( 'NONE',  ( 22.36058758039612471, 3.933412737179332375, -7.046732538784932665 ) ) ;
#37359=ORIENTED_EDGE ( 'NONE', *, *, #37729, .F. ) ;
#37360=CARTESIAN_POINT ( 'NONE',  ( -72.84075015605040448, 2.241838945666980720, 9.875564344321709598 ) ) ;
#37361=CARTESIAN_POINT ( 'NONE',  ( 36.39055874488383324, -3.588954754978076256, 5.770159689808049386 ) ) ;
#37364=ORIENTED_EDGE ( 'NONE', *, *, #36133, .T. ) ;
#37366=CARTESIAN_POINT ( 'NONE',  ( 29.51386328998167485, -3.424974278474657297, -4.784120810196317741 ) ) ;
#37367=CARTESIAN_POINT ( 'NONE',  ( 37.17696383940524640, -2.564559183315724855, -5.980961330593222769 ) ) ;
#37375=CARTESIAN_POINT ( 'NONE',  ( 16.74143876458001401, 14.78209838809407017, -2.499999999999999556 ) ) ;
#37376=CARTESIAN_POINT ( 'NONE',  ( 21.83244621861719637, 0.3031599029397021305, -8.132627632833301590 ) ) ;
#37377=CARTESIAN_POINT ( 'NONE',  ( 36.68199778546589584, -1.920130161400638302, -5.804599519094802318 ) ) ;
#37380=CARTESIAN_POINT ( 'NONE',  ( 26.72282919489819264, 1.562893068380316830, -4.355115922428256070 ) ) ;
#37384=CARTESIAN_POINT ( 'NONE',  ( 36.66477430105471313, -3.237310495223860496, 5.925263590695005966 ) ) ;
#37387=CARTESIAN_POINT ( 'NONE',  ( 88.87549651282381546, -1.666836616135117799, 1.222388837546040330 ) ) ;
#37389=CARTESIAN_POINT ( 'NONE',  ( 22.37955706836635983, 4.044372726829571718, 2.563398534706760046 ) ) ;
#37391=CARTESIAN_POINT ( 'NONE',  ( 24.49274287821404172, 2.967433299905803512, 3.639746199902306412 ) ) ;
#37399=CARTESIAN_POINT ( 'NONE',  ( 21.58863023475808873, 7.202558683720228672, -2.923977588977705544 ) ) ;
#37406=CARTESIAN_POINT ( 'NONE',  ( 21.74132580300875617, 6.055672829483719433, -3.293574973715298615 ) ) ;
#37409=CARTESIAN_POINT ( 'NONE',  ( 24.83717141299267794, -2.182840666565796006, 6.391756413845674167 ) ) ;
#37410=CARTESIAN_POINT ( 'NONE',  ( -80.78522550881831421, -5.650799850798457591, -4.938740386049992104 ) ) ;
#37413=CARTESIAN_POINT ( 'NONE',  ( 87.52176134051316581, -1.326109120332903846, -4.764847963194966063 ) ) ;
#37425=CARTESIAN_POINT ( 'NONE',  ( 36.64566332290064565, -2.462282481428397674, 5.925840058891846063 ) ) ;
#37427=CIRCLE ( 'NONE', #21012, 31.65266504832700534 ) ;
#37431=CARTESIAN_POINT ( 'NONE',  ( 21.91440216420213360, -2.652013307545402654, 3.626670478179643275 ) ) ;
#37441=CARTESIAN_POINT ( 'NONE',  ( 22.04383411009131422, 3.353668517320957498, 4.622206337531012288 ) ) ;
#37442=CARTESIAN_POINT ( 'NONE',  ( 36.06837000820846839, -1.500464606615067753, 5.629282289834582009 ) ) ;
#37448=LINE ( 'NONE', #12, #25283 ) ;
#37449=CARTESIAN_POINT ( 'NONE',  ( 85.59581148158818564, 2.212446518294743480, -3.358098885934541755 ) ) ;
#37453=CARTESIAN_POINT ( 'NONE',  ( 24.40178566874492816, 2.839217219712215634, -3.817826656981023081 ) ) ;
#37456=CARTESIAN_POINT ( 'NONE',  ( 21.85643539959774628, 6.760345589247273246, -10.71366635798555578 ) ) ;
#37460=CARTESIAN_POINT ( 'NONE',  ( 28.84632484126239760, -3.982640415251879062, -4.149463024310225734 ) ) ;
#37462=CARTESIAN_POINT ( 'NONE',  ( 87.05115134601746263, 0.5777397079708905814, 5.111878656935144427 ) ) ;
#37465=CARTESIAN_POINT ( 'NONE',  ( 15.13412790246976058, -4.097024560658993231, 2.561171989064709997 ) ) ;
#37468=CARTESIAN_POINT ( 'NONE',  ( 34.77288883663810992, -3.165682983332114286, -5.633548307088366514 ) ) ;
#37476=CARTESIAN_POINT ( 'NONE',  ( 32.06782253780797021, 0.2506623542119881254, 4.730668526418615905 ) ) ;
#37490=CARTESIAN_POINT ( 'NONE',  ( 24.01385423370390626, 3.312006728691793800, 3.343613740752824803 ) ) ;
#37494=EDGE_LOOP ( 'NONE', ( #32554, #13334, #8571, #36699 ) ) ;
#37498=CARTESIAN_POINT ( 'NONE',  ( 14.76930820911141495, 12.55346518732212857, -2.511505761737421683 ) ) ;
#37506=CYLINDRICAL_SURFACE ( 'NONE', #3056, 12.80480339192541628 ) ;
#37511=CARTESIAN_POINT ( 'NONE',  ( 29.23504802441905071, -0.3867851007456850065, 5.903809272860179647 ) ) ;
#37515=CARTESIAN_POINT ( 'NONE',  ( 21.98512429705750648, 0.2333936388226412750, -7.692680552510582359 ) ) ;
#37516=CARTESIAN_POINT ( 'NONE',  ( -71.92837670882107659, -0.7829914368874778541, 38.00000000000000711 ) ) ;
#37519=CARTESIAN_POINT ( 'NONE',  ( 33.45155509882757627, -3.250653912085893715, -5.427322220725915969 ) ) ;
#37521=CARTESIAN_POINT ( 'NONE',  ( 36.19289006885171034, -3.601804653832907377, -5.745383553838919077 ) ) ;
#37523=DIRECTION ( 'NONE',  ( 1.000000000000000000, 0.000000000000000000, 0.000000000000000000 ) ) ;
#37528=CARTESIAN_POINT ( 'NONE',  ( -76.42881101814404587, 9.150640561982111620, 9.834217937602943493 ) ) ;
#37529=CARTESIAN_POINT ( 'NONE',  ( 86.75210013534866960, -0.2795847087395720298, -5.842668109216860195 ) ) ;
#37530=CARTESIAN_POINT ( 'NONE',  ( 21.25000211823397933, 8.711688037120479677, 2.624172062053642396 ) ) ;
#37537=CARTESIAN_POINT ( 'NONE',  ( 33.45716606812183613, -3.829385970599605393, -5.093809925484540813 ) ) ;
#37543=CARTESIAN_POINT ( 'NONE',  ( 22.38247687632654959, 4.949581816714125004, 3.033779412410520848 ) ) ;
#37549=CARTESIAN_POINT ( 'NONE',  ( 25.98038313832403290, 0.8809173887663540592, 4.427613202293294137 ) ) ;
#37557=CARTESIAN_POINT ( 'NONE',  ( 22.53076953550388950, -1.409035359855524749, -9.122014670555362414 ) ) ;
#37558=CARTESIAN_POINT ( 'NONE',  ( 21.85643539959776760, -15.11462368761991293, 2.500000000000000000 ) ) ;
#37560=CARTESIAN_POINT ( 'NONE',  ( -74.02963593684843602, 8.693065175645321219, 9.511771665882234217 ) ) ;
#37561=CARTESIAN_POINT ( 'NONE',  ( 36.26322319698421381, -3.626588400798672396, 5.736275618128532372 ) ) ;
#37566=CARTESIAN_POINT ( 'NONE',  ( 34.14240489748642204, -3.849676338616116578, -5.233289980769661121 ) ) ;
#37573=CARTESIAN_POINT ( 'NONE',  ( 27.24896854768403998, 1.198804712641063253, -4.456107267776617142 ) ) ;
#37576=CARTESIAN_POINT ( 'NONE',  ( 24.75839165839662925, 3.019244830385916956, -3.350409272483306111 ) ) ;
#37579=CARTESIAN_POINT ( 'NONE',  ( 25.34282642491231030, 1.862868491491909362, 4.161759000817419007 ) ) ;
#37583=CARTESIAN_POINT ( 'NONE',  ( 87.73660070961769009, -1.594395026316068220, -4.241058185374163791 ) ) ;
#37584=CARTESIAN_POINT ( 'NONE',  ( 35.84098429011871900, -3.161360823169788059, -5.800250434590431325 ) ) ;
#37586=CARTESIAN_POINT ( 'NONE',  ( 25.66089067728524142, 2.145916329718004167, 4.138078528123439348 ) ) ;
#37599=EDGE_CURVE ( 'NONE', #17308, #32259, #8545, .T. ) ;
#37603=CARTESIAN_POINT ( 'NONE',  ( -17.27251170661583402, -8.656638842136340273, 2.500000000000000000 ) ) ;
#37604=DIRECTION ( 'NONE',  ( -1.385724075720358314E-16, 1.000000000000000000, 0.000000000000000000 ) ) ;
#37605=CARTESIAN_POINT ( 'NONE',  ( 21.72407540026657102, 6.220878712065926130, -3.231759089253579909 ) ) ;
#37608=CARTESIAN_POINT ( 'NONE',  ( 25.11223377877777807, -2.893972711065841086, 5.714375009671201155 ) ) ;
#37609=CARTESIAN_POINT ( 'NONE',  ( -76.34937612267491147, -4.253321125015449233, -8.424943696077420441 ) ) ;
#37612=CARTESIAN_POINT ( 'NONE',  ( 88.23373314635465192, -2.194529332924425091, 2.156499936145213070 ) ) ;
#37619=CARTESIAN_POINT ( 'NONE',  ( 85.73057283473386292, 0.7451135881651274051, 5.912605931588609920 ) ) ;
#37621=CARTESIAN_POINT ( 'NONE',  ( 36.78910914328132264, -3.040808538379049519, 5.948228248412681829 ) ) ;
#37623=CARTESIAN_POINT ( 'NONE',  ( 85.09836244081553502, 2.771204891246429547, 1.045684100250478643 ) ) ;
#37626=CARTESIAN_POINT ( 'NONE',  ( 14.76394723472931325, -5.159572269938053068, 2.499999999999999556 ) ) ;
#37627=CARTESIAN_POINT ( 'NONE',  ( -70.17231294992166113, -45.80665935166715741, 9.973038756526108273 ) ) ;
#37628=VECTOR ( 'NONE', #17937, 1000.000000000000000 ) ;
#37638=CARTESIAN_POINT ( 'NONE',  ( 23.73424597286967952, 2.447426312426829398, 4.258169151716980849 ) ) ;
#37645=CARTESIAN_POINT ( 'NONE',  ( 86.19938718321334647, 1.534481642798401380, -4.634396957419961716 ) ) ;
#37651=CARTESIAN_POINT ( 'NONE',  ( 22.23015695420303928, 3.514796972574160794, -4.336854520634696009 ) ) ;
#37653=CARTESIAN_POINT ( 'NONE',  ( 21.85643539959778181, 2.657715471900086612, -15.25567151318962367 ) ) ;
#37655=VERTEX_POINT ( 'NONE', #37721 ) ;
#37658=CARTESIAN_POINT ( 'NONE',  ( 87.46579090913228072, 0.1119968706995537605, 4.710562776971725540 ) ) ;
#37663=CARTESIAN_POINT ( 'NONE',  ( 14.65281498853338782, -5.050736788034034142, 2.492857568421119829 ) ) ;
#37664=CARTESIAN_POINT ( 'NONE',  ( 36.97979765674093500, -2.956942819130029765, -5.977989802757186055 ) ) ;
#37669=VECTOR ( 'NONE', #23750, 1000.000000000000000 ) ;
#37672=CARTESIAN_POINT ( 'NONE',  ( 30.88164994506820449, 0.6966255426222526248, 4.496776574569896212 ) ) ;
#37673=LINE ( 'NONE', #9896, #5411 ) ;
#37678=CARTESIAN_POINT ( 'NONE',  ( 88.33288515625950765, -0.8619645424494146724, 0.9116167777034707154 ) ) ;
#37679=CARTESIAN_POINT ( 'NONE',  ( -80.67847586496442602, -6.621814235793498149, -2.260889596539092938 ) ) ;
#37680=FACE_BOUND ( 'NONE', #36508, .T. ) ;
#37681=( NAMED_UNIT ( * ) PLANE_ANGLE_UNIT ( ) SI_UNIT ( $, .RADIAN. ) );
#37686=CARTESIAN_POINT ( 'NONE',  ( 24.30163658516156033, 3.125396681048508096, 3.455688527987379910 ) ) ;
#37695=CARTESIAN_POINT ( 'NONE',  ( 19.31369698277901037, 7.427556948433061912, -3.124657957306991918 ) ) ;
#37705=CARTESIAN_POINT ( 'NONE',  ( 29.75157451403313758, 0.8046206704518127362, -4.785270562610461020 ) ) ;
#37707=CARTESIAN_POINT ( 'NONE',  ( 20.41865484760615956, -3.555473204735890125, 2.500000000123285826 ) ) ;
#37711=DIRECTION ( 'NONE',  ( 1.000000000000000000, 0.000000000000000000, 0.000000000000000000 ) ) ;
#37713=LINE ( 'NONE', #21694, #32152 ) ;
#37714=CARTESIAN_POINT ( 'NONE',  ( 21.70417750497355058, 4.205083950317406227, -2.944929369283658893 ) ) ;
#37721=CARTESIAN_POINT ( 'NONE',  ( 21.85643539959777115, -15.24623503193425123, 0.9260495571226281530 ) ) ;
#37722=CARTESIAN_POINT ( 'NONE',  ( 21.85643539959776760, -15.11462368761991293, 2.500000000000000000 ) ) ;
#37725=B_SPLINE_CURVE_WITH_KNOTS ( 'NONE', 3,
 ( #28008, #16063, #9683, #18743, #18955, #9266 ),
 .UNSPECIFIED., .F., .F.,
 ( 4, 2, 4 ),
 ( 0.000000000000000000, 0.0004188893554603549240, 0.0008377787109207098480 ),
 .UNSPECIFIED. ) ;
#37729=EDGE_CURVE ( 'NONE', #16251, #4540, #18182, .T. ) ;
#37731=ORIENTED_EDGE ( 'NONE', *, *, #26107, .T. ) ;
#37734=CARTESIAN_POINT ( 'NONE',  ( 24.43561622922326038, 2.813159176002239192, 3.833666132760469303 ) ) ;
#37739=CARTESIAN_POINT ( 'NONE',  ( 22.87946623223324139, 4.338853656372669398, 3.053785548036103581 ) ) ;
#37746=VERTEX_POINT ( 'NONE', #28686 ) ;
#37748=CARTESIAN_POINT ( 'NONE',  ( 23.61296149509351139, 0.4561011562658625618, 5.500673751672807477 ) ) ;
#37754=CARTESIAN_POINT ( 'NONE',  ( 21.85643539959777826, -9.955546997263933662, -6.545918539092090427 ) ) ;
#37757=ORIENTED_EDGE ( 'NONE', *, *, #4732, .F. ) ;
#37758=CARTESIAN_POINT ( 'NONE',  ( -74.45682198657978290, 9.142387462817648469, 9.358043394732074916 ) ) ;
#37759=CARTESIAN_POINT ( 'NONE',  ( 36.87624210086934085, -3.358183527908076282, 5.907681686615140038 ) ) ;
#37761=ADVANCED_FACE ( 'NONE', ( #38738 ), #19415, .T. ) ;
#37764=EDGE_CURVE ( 'NONE', #24052, #615, #30671, .T. ) ;
#37765=CARTESIAN_POINT ( 'NONE',  ( -80.90946895960888696, 10.56086125674553422, -1.015159195828805760 ) ) ;
#37767=CARTESIAN_POINT ( 'NONE',  ( 35.22138010156052701, -1.046722844669025765, -5.410276998223191747 ) ) ;
#37769=CARTESIAN_POINT ( 'NONE',  ( 19.86572073012567330, 6.626268771028025917, 3.306924192844295618 ) ) ;
#37771=CARTESIAN_POINT ( 'NONE',  ( 29.65186663566715808, -3.798820256635906834, 4.430807847150231460 ) ) ;
#37774=CARTESIAN_POINT ( 'NONE',  ( 23.61900895148505697, 0.7560519036968751383, -5.377082254995243282 ) ) ;
#37776=CARTESIAN_POINT ( 'NONE',  ( 26.63902384589101047, 1.612943561579256224, -4.338441080883199241 ) ) ;
#37781=CARTESIAN_POINT ( 'NONE',  ( 37.00288072789806648, -2.989026547920700327, 5.981592474277436899 ) ) ;
#37782=EDGE_CURVE ( 'NONE', #40651, #14452, #25798, .T. ) ;
#37784=CARTESIAN_POINT ( 'NONE',  ( 84.43092178082896737, 2.949567725576020649, 1.921192885956162444 ) ) ;
#37785=CARTESIAN_POINT ( 'NONE',  ( 24.75815691998409562, 3.019130790117518170, 3.350895687454368055 ) ) ;
#37789=CARTESIAN_POINT ( 'NONE',  ( 24.75839165839662925, 3.019244830385916956, -3.350409272483306111 ) ) ;
#37794=UNCERTAINTY_MEASURE_WITH_UNIT (LENGTH_MEASURE( 1.000000000000000082E-05 ), #6529, 'distance_accuracy_value', 'NONE');
#37806=CARTESIAN_POINT ( 'NONE',  ( -71.90227038838925466, -21.04509535909790330, 9.952591258774150518 ) ) ;
#37808=CARTESIAN_POINT ( 'NONE',  ( 22.62157167972026883, 4.589994619255199915, -3.081681181103287592 ) ) ;
#37814=CARTESIAN_POINT ( 'NONE',  ( -80.88644286667957317, -6.600206128780238046, -1.001251069996826448 ) ) ;
#37817=CARTESIAN_POINT ( 'NONE',  ( 84.75081314860828741, 2.206698042984908792, -4.319373971756642838 ) ) ;
#37818=CARTESIAN_POINT ( 'NONE',  ( 22.47899254214195608, 3.957058747972870716, -2.823133405592673562 ) ) ;
#37821=CARTESIAN_POINT ( 'NONE',  ( 22.07330900774856275, 4.463300359340192536, 0.7514602381188923985 ) ) ;
#37825=CIRCLE ( 'NONE', #30620, 24.28220113893567245 ) ;
#37827=ADVANCED_FACE ( 'NONE', ( #19216 ), #10133, .T. ) ;
#37828=CARTESIAN_POINT ( 'NONE',  ( 14.80983598776561472, -5.580000773509008027, -2.503340399836785579 ) ) ;
#37830=CARTESIAN_POINT ( 'NONE',  ( 85.61058318453605409, 0.9550117787157472726, 5.816704139769944604 ) ) ;
#37831=VERTEX_POINT ( 'NONE', #16514 ) ;
#37832=CARTESIAN_POINT ( 'NONE',  ( 21.25348936832362412, 3.320962282439187341, 3.523519052146550923 ) ) ;
#37835=CARTESIAN_POINT ( 'NONE',  ( 87.18644375116411993, 0.4257728571452945587, -5.011944538332810062 ) ) ;
#37843=CARTESIAN_POINT ( 'NONE',  ( -77.13767261641073958, -6.081113133698417883, 7.841263487880433480 ) ) ;
#37847=CARTESIAN_POINT ( 'NONE',  ( 36.00559039101765535, -3.152632923976596224, 5.825941197649304293 ) ) ;
#37848=CARTESIAN_POINT ( 'NONE',  ( 23.78674307609086824, 1.600237366897277802, 4.774347307045557542 ) ) ;
#37849=CARTESIAN_POINT ( 'NONE',  ( 37.10781593239299525, -2.412025766632669210, 5.952297030325896188 ) ) ;
#37857=DIRECTION ( 'NONE',  ( -7.232507224765808510E-18, 1.000000000000000000, 0.000000000000000000 ) ) ;
#37861=ORIENTED_EDGE ( 'NONE', *, *, #13402, .T. ) ;
#37862=CARTESIAN_POINT ( 'NONE',  ( 22.02527683978544104, 4.022755422383132107, -4.157466662046956252 ) ) ;
#37866=CARTESIAN_POINT ( 'NONE',  ( 21.85643539959780313, -9.021070270546461600, 11.21731785579436291 ) ) ;
#37870=CARTESIAN_POINT ( 'NONE',  ( 85.64504565501374600, 2.098084819171330828, -4.577105872335450520 ) ) ;
#37872=CARTESIAN_POINT ( 'NONE',  ( -81.82381003581529910, -5.600672066111338943, -0.2226990585086200125 ) ) ;
#37873=CARTESIAN_POINT ( 'NONE',  ( 14.89717971670494556, -5.930256159152071938, 2.520399783277118111 ) ) ;
#37874=CARTESIAN_POINT ( 'NONE',  ( 36.89700021831158949, -3.001725562179715201, -5.965067260026661877 ) ) ;
#37882=CARTESIAN_POINT ( 'NONE',  ( 32.91909972634648796, -3.046172459632647822, 5.344219682368552604 ) ) ;
#37885=CARTESIAN_POINT ( 'NONE',  ( 36.87008432447370154, -2.088660079878024156, 5.864835073014669220 ) ) ;
#37892=CARTESIAN_POINT ( 'NONE',  ( 88.26456443100552463, -0.7852234611469554038, -1.669442870725792449 ) ) ;
#37893=CARTESIAN_POINT ( 'NONE',  ( -75.23895599219262920, 9.844379164151915163, -9.029202135315509636 ) ) ;
#37895=( LENGTH_UNIT ( ) NAMED_UNIT ( * ) SI_UNIT ( .MILLI., .METRE. ) );
#37899=CARTESIAN_POINT ( 'NONE',  ( 22.43706763645577595, 4.742359000873816122, 3.190859319307013831 ) ) ;
#37903=ORIENTED_EDGE ( 'NONE', *, *, #12365, .F. ) ;
#37908=CARTESIAN_POINT ( 'NONE',  ( 16.06987909445021856, 10.26701343839525826, -2.714491302820267737 ) ) ;
#37917=CARTESIAN_POINT ( 'NONE',  ( 14.72270833303476500, 13.21629034477860998, 2.500000000000005773 ) ) ;
#37918=CARTESIAN_POINT ( 'NONE',  ( 30.01304521823198712, -3.946539318896107318, -3.661452490695084272 ) ) ;
#37919=VECTOR ( 'NONE', #22874, 1000.000000000000000 ) ;
#37928=CARTESIAN_POINT ( 'NONE',  ( 36.96297856671265691, -3.150510869464469899, -5.966408781979020581 ) ) ;
#37931=CARTESIAN_POINT ( 'NONE',  ( 15.21509089441225981, -3.846322154070160426, -2.581080931073590268 ) ) ;
#37933=CARTESIAN_POINT ( 'NONE',  ( -80.76903247909713457, 10.51040070415216299, 4.971711105935894714 ) ) ;
#37937=DIRECTION ( 'NONE',  ( -0.9999026450364576490, -0.01395351027862084224, 0.000000000000000000 ) ) ;
#37944=CARTESIAN_POINT ( 'NONE',  ( 30.77693785172156282, -3.327810147074260705, 4.963017966735677078 ) ) ;
#37945=CARTESIAN_POINT ( 'NONE',  ( 22.62052229059043640, 3.442390791615673518, 4.088590503876035953 ) ) ;
#37957=CARTESIAN_POINT ( 'NONE',  ( 25.95513938031040269, 0.9030353738542202802, 4.429115342626236185 ) ) ;
#37964=ORIENTED_EDGE ( 'NONE', *, *, #21922, .T. ) ;
#37965=CARTESIAN_POINT ( 'NONE',  ( 22.58802438714224081, -2.565763546402358486, 8.787087332313648247 ) ) ;
#37968=CARTESIAN_POINT ( 'NONE',  ( -74.09938582373443694, 6.767060077088832060, 10.75363259336874933 ) ) ;
#37969=CARTESIAN_POINT ( 'NONE',  ( 27.44078372763345541, 0.9562943962831292888, -4.489200806087393580 ) ) ;
#37970=VERTEX_POINT ( 'NONE', #22034 ) ;
#37973=VECTOR ( 'NONE', #11670, 1000.000000000000000 ) ;
#37976=CARTESIAN_POINT ( 'NONE',  ( 36.49360370896476979, -3.560832467653986200, -5.796016089073773969 ) ) ;
#37980=CARTESIAN_POINT ( 'NONE',  ( 15.93325076494975256, 10.76686990589485049, 2.654092171972521452 ) ) ;
#37987=CARTESIAN_POINT ( 'NONE',  ( 23.99747144395669807, 1.007762411719124618, -4.993298325900711987 ) ) ;
#37988=CARTESIAN_POINT ( 'NONE',  ( 30.57682521627442185, -3.782462783739084067, -4.515814102832556465 ) ) ;
#37989=DIRECTION ( 'NONE',  ( 0.000000000000000000, -0.000000000000000000, -1.000000000000000000 ) ) ;
#37994=CARTESIAN_POINT ( 'NONE',  ( 88.55280947256005675, -1.781472883390815110, -2.828200999223334566 ) ) ;
#37998=CARTESIAN_POINT ( 'NONE',  ( 24.56661666422449741, 2.976733537025225029, 3.586665788575320146 ) ) ;
#38000=CARTESIAN_POINT ( 'NONE',  ( 25.06774369592266538, 3.218163280828734596, -2.425390343617369826 ) ) ;
#38006=ORIENTED_EDGE ( 'NONE', *, *, #30995, .T. ) ;
#38018=CARTESIAN_POINT ( 'NONE',  ( 21.85643539959774273, 11.87467848218428834, -0.9583437110454642305 ) ) ;
#38019=CARTESIAN_POINT ( 'NONE',  ( 23.43039554023339122, 3.779663734359625771, -3.137929522636683455 ) ) ;
#38020=ORIENTED_EDGE ( 'NONE', *, *, #28084, .T. ) ;
#38025=CARTESIAN_POINT ( 'NONE',  ( -77.69396300944833911, -6.284379105152234857, -7.366555388289405926 ) ) ;
#38029=CARTESIAN_POINT ( 'NONE',  ( 86.43572624768424362, -0.5192074800720991590, -5.777013305174518720 ) ) ;
#38040=B_SPLINE_CURVE_WITH_KNOTS ( 'NONE', 3,
 ( #23362, #7707, #20258, #30975, #28068, #18587, #8916, #11996, #37128, #37530, #2578, #24993, #20873 ),
 .UNSPECIFIED., .F., .F.,
 ( 4, 2, 1, 2, 2, 2, 4 ),
 ( 0.3391172959757620120, 0.4217276339787944250, 0.4630328029803104650, 0.4836853874810680409, 0.5043379719818256168, 0.6695586479878841146, 1.000000000000000000 ),
 .UNSPECIFIED. ) ;
#38042=CARTESIAN_POINT ( 'NONE',  ( 35.45320544181257105, -1.915487943862905773, 5.739728166845379675 ) ) ;
#38047=CARTESIAN_POINT ( 'NONE',  ( 8.290806648384990041, -10.90558813203967148, 2.500000000000000000 ) ) ;
#38048=CARTESIAN_POINT ( 'NONE',  ( -70.01360951184285852, -48.30983266357521444, 9.958407075284599230 ) ) ;
#38054=CARTESIAN_POINT ( 'NONE',  ( -75.54470190824260101, -5.203473257850061984, 8.872432550771755189 ) ) ;
#38055=ORIENTED_EDGE ( 'NONE', *, *, #8902, .F. ) ;
#38059=CARTESIAN_POINT ( 'NONE',  ( 22.02680808259401957, 1.706773391190979039, 6.102062103760552247 ) ) ;
#38063=ADVANCED_FACE ( 'NONE', ( #18257 ), #40288, .T. ) ;
#38066=CARTESIAN_POINT ( 'NONE',  ( 85.35528217256008077, 2.482620454404805166, 2.380853641630215289 ) ) ;
#38070=CARTESIAN_POINT ( 'NONE',  ( 22.58150593364278791, 3.840177467176269843, -3.813772455918038595 ) ) ;
#38073=EDGE_CURVE ( 'NONE', #4341, #26564, #19363, .T. ) ;
#38075=CARTESIAN_POINT ( 'NONE',  ( 21.85643539959775694, 0.3794388012242833064, 14.22155525766799045 ) ) ;
#38077=CARTESIAN_POINT ( 'NONE',  ( 70.21968079846043054, -4.730580361459368888, 6.000000000000000888 ) ) ;
#38079=CARTESIAN_POINT ( 'NONE',  ( 85.19300053701067554, 2.612159253720373275, 3.340723803646971302 ) ) ;
#38082=CARTESIAN_POINT ( 'NONE',  ( 26.27630619708502735, -2.986427969042946717, 4.300631657982672884 ) ) ;
#38083=CARTESIAN_POINT ( 'NONE',  ( 34.13619771771038813, -3.132990105432221561, -5.534177259546053662 ) ) ;
#38085=LINE ( 'NONE', #21643, #11452 ) ;
#38086=CARTESIAN_POINT ( 'NONE',  ( 30.63618695437729400, -3.604233874750632616, -4.761443182589183643 ) ) ;
#38089=CARTESIAN_POINT ( 'NONE',  ( 28.82329466325964873, -3.930707862937422359, 4.251064711185412293 ) ) ;
#38091=EDGE_LOOP ( 'NONE', ( #9602, #29533, #30361, #40634 ) ) ;
#38092=CARTESIAN_POINT ( 'NONE',  ( 21.73837075214035508, 4.234937956566636963, 2.803927625586267514 ) ) ;
#38100=CARTESIAN_POINT ( 'NONE',  ( -17.69482985384421880, -42.37473357531882101, 6.000000000000000000 ) ) ;
#38105=ORIENTED_EDGE ( 'NONE', *, *, #39587, .T. ) ;
#38108=VECTOR ( 'NONE', #3976, 1000.000000000000000 ) ;
#38114=CARTESIAN_POINT ( 'NONE',  ( 19.77298615262494863, 6.502606513668326649, -3.292450719231072132 ) ) ;
#38124=CARTESIAN_POINT ( 'NONE',  ( 17.73639058713895267, 11.88077765114964279, 2.500000000000007550 ) ) ;
#38125=CARTESIAN_POINT ( 'NONE',  ( 30.13146195922598380, -4.635528103762326602, -0.9093114724505712010 ) ) ;
#38128=CIRCLE ( 'NONE', #28915, 24.28220113893567245 ) ;
#38130=CARTESIAN_POINT ( 'NONE',  ( -70.92837670882107659, -37.87473357531881391, 0.000000000000000000 ) ) ;
#38133=CARTESIAN_POINT ( 'NONE',  ( 23.13399818617703119, 3.188625524576914394, -3.769247952470702323 ) ) ;
#38134=CARTESIAN_POINT ( 'NONE',  ( 11.29080664838499182, -35.94265729135299381, -6.000000000000000000 ) ) ;
#38147=CARTESIAN_POINT ( 'NONE',  ( 24.24310498680376469, 2.794393895970717523, 3.876533112567932537 ) ) ;
#38156=VERTEX_POINT ( 'NONE', #15381 ) ;
#38158=CARTESIAN_POINT ( 'NONE',  ( 21.73550026715119543, 0.2732327172998176845, 8.957745052953152154 ) ) ;
#38169=CARTESIAN_POINT ( 'NONE',  ( 22.49677218534670331, -0.6234722885575160189, 9.207484322151008982 ) ) ;
#38172=CARTESIAN_POINT ( 'NONE',  ( -74.21348950129103628, -2.081539577114183803, 9.498975700750209583 ) ) ;
#38173=CARTESIAN_POINT ( 'NONE',  ( 21.96608578389022171, 0.2111773095693803282, -7.751388582462531929 ) ) ;
#38176=CARTESIAN_POINT ( 'NONE',  ( 23.38231645333376818, 4.144860998403037122, 2.192943146592336134 ) ) ;
#38177=CARTESIAN_POINT ( 'NONE',  ( 28.82242951612792581, -3.931231161810520014, -4.250723811025777010 ) ) ;
#38178=CARTESIAN_POINT ( 'NONE',  ( 33.94570531977476691, -0.4887297205857646931, -5.122339712429196723 ) ) ;
#38180=CARTESIAN_POINT ( 'NONE',  ( 15.78123433858440450, 10.66027319286623687, 2.669441307767606020 ) ) ;
#38182=CARTESIAN_POINT ( 'NONE',  ( -5.316495087772350914, -32.84709638682603838, 0.000000000000000000 ) ) ;
#38186=CARTESIAN_POINT ( 'NONE',  ( 25.37327375539348751, 1.417373392026759493, -4.399323053431193564 ) ) ;
#38187=CARTESIAN_POINT ( 'NONE',  ( 29.87221045764711747, 1.073546826849551161, -4.301872174529671078 ) ) ;
#38190=EDGE_LOOP ( 'NONE', ( #28754, #10248, #20570, #18 ) ) ;
#38194=CARTESIAN_POINT ( 'NONE',  ( 84.96877181165257298, 2.299433286287765554, -4.273906790846864645 ) ) ;
#38198=CARTESIAN_POINT ( 'NONE',  ( 27.14060876212918316, 1.318306631261646045, 4.438683710678335004 ) ) ;
#38202=EDGE_CURVE ( 'NONE', #22978, #24175, #10521, .T. ) ;
#38211=EDGE_CURVE ( 'NONE', #32354, #10467, #21543, .T. ) ;
#38212=B_SPLINE_CURVE_WITH_KNOTS ( 'NONE', 3,
 ( #33362, #33562, #30672, #15207, #30049, #1862, #2265, #36830, #5339, #27761, #36425, #20984, #27358, #15003, #17875, #8612, #23849, #24057, #30878, #26955, #21191, #36625, #12104, #8813, #33764, #5747, #5542, #39500, #14580, #40315, #40119, #17668, #8410 ),
 .UNSPECIFIED., .F., .F.,
 ( 4, 2, 2, 2, 2, 1, 1, 1, 1, 2, 2, 2, 2, 1, 1, 1, 1, 1, 2, 2, 4 ),
 ( 0.000000000000000000, 0.1250000000000277278, 0.1875000000000412725, 0.2187500000000483225, 0.2343750000000518474, 0.2421875000000538458, 0.2460937500000548173, 0.2480468750000554834, 0.2490234375000556222, 0.2495117187500556777, 0.2500000000000557332, 0.3750000000000170974, 0.4374999999999981126, 0.4687499999999886202, 0.4843749999999836242, 0.4921874999999813483, 0.4960937499999801825, 0.4980468749999799050, 0.4990234374999800160, 0.4999999999999801270, 1.000000000000000000 ),
 .UNSPECIFIED. ) ;
#38213=CARTESIAN_POINT ( 'NONE',  ( 27.34605239800119136, -4.443250099184577806, 3.670018459242561981 ) ) ;
#38215=CARTESIAN_POINT ( 'NONE',  ( 21.85643539959777115, 5.662525507098640887, -13.61651877770312957 ) ) ;
#38216=CARTESIAN_POINT ( 'NONE',  ( 23.14021789239912863, 4.034458455300417690, -3.103648843234191101 ) ) ;
#38217=VERTEX_POINT ( 'NONE', #16990 ) ;
#38223=CARTESIAN_POINT ( 'NONE',  ( -74.23111751286343463, -2.107699029187716455, -9.492660611869487397 ) ) ;
#38227=CARTESIAN_POINT ( 'NONE',  ( 88.13894822871212398, -2.422255244508634053, -0.8714879239747004291 ) ) ;
#38229=DIRECTION ( 'NONE',  ( 0.000000000000000000, 0.000000000000000000, 1.000000000000000000 ) ) ;
#38230=CARTESIAN_POINT ( 'NONE',  ( 22.07207100664286870, 4.383386263552846884, 1.524166271142376239 ) ) ;
#38231=CARTESIAN_POINT ( 'NONE',  ( 33.64165290529265206, -1.232672941509324716, 5.456991580957781807 ) ) ;
#38237=CARTESIAN_POINT ( 'NONE',  ( 35.45419760563620315, -1.912960601587893716, 5.739883018005628834 ) ) ;
#38238=ADVANCED_FACE ( 'NONE', ( #29562 ), #21775, .T. ) ;
#38241=CARTESIAN_POINT ( 'NONE',  ( 85.32384696181071604, 2.517929975123688990, -2.669340390032339361 ) ) ;
#38245=EDGE_CURVE ( 'NONE', #19379, #20545, #33921, .T. ) ;
#38246=DIRECTION ( 'NONE',  ( 0.000000000000000000, -0.000000000000000000, -1.000000000000000000 ) ) ;
#38248=EDGE_CURVE ( 'NONE', #10739, #37970, #21329, .T. ) ;
#38251=CARTESIAN_POINT ( 'NONE',  ( -78.33784134423007117, -6.465022251522651864, 6.728521485594535001 ) ) ;
#38256=ORIENTED_EDGE ( 'NONE', *, *, #8812, .F. ) ;
#38259=CARTESIAN_POINT ( 'NONE',  ( 23.79107460766518400, 2.334731070376283579, 4.312254787772835662 ) ) ;
#38260=EDGE_LOOP ( 'NONE', ( #25248, #20514, #16375, #15005 ) ) ;
#38263=CARTESIAN_POINT ( 'NONE',  ( 14.75988012746532441, 13.12337194104328653, -2.499999999999869882 ) ) ;
#38269=CARTESIAN_POINT ( 'NONE',  ( 24.12389204279378063, 2.961437545701208318, -3.763128746285317128 ) ) ;
#38273=CARTESIAN_POINT ( 'NONE',  ( 21.85643539959774273, -5.916281280498693285, 11.28130179073419015 ) ) ;
#38274=CARTESIAN_POINT ( 'NONE',  ( 21.85643539959905368, 4.448544635521362700, -2.117591927232864712 ) ) ;
#38277=CARTESIAN_POINT ( 'NONE',  ( 88.80901725076027731, -1.591322664339660298, -1.862171775454326550 ) ) ;
#38279=CARTESIAN_POINT ( 'NONE',  ( 14.77315594796431064, 13.19392823276595195, 2.499999999999996891 ) ) ;
#38280=CARTESIAN_POINT ( 'NONE',  ( 14.73577947313193270, -4.490654621266425117, 2.506272791592270899 ) ) ;
#38281=CARTESIAN_POINT ( 'NONE',  ( 36.08720898791031573, -2.181208829428816109, 5.838679753647628701 ) ) ;
#38283=CARTESIAN_POINT ( 'NONE',  ( 36.14153500552394149, -3.143492148517922580, -5.847158642575881693 ) ) ;
#38286=CARTESIAN_POINT ( 'NONE',  ( -72.89163490554884106, 1.565256442275936966, 10.95728629449147995 ) ) ;
#38289=CARTESIAN_POINT ( 'NONE',  ( 29.54621482125871879, -3.606128174059152869, 4.678900705189122711 ) ) ;
#38292=CARTESIAN_POINT ( 'NONE',  ( 37.10858378118385303, -2.405180162493830487, 5.952030529888895138 ) ) ;
#38296=CARTESIAN_POINT ( 'NONE',  ( 87.20834523746592026, -1.621581766752904441, -4.479905140931061958 ) ) ;
#38300=CARTESIAN_POINT ( 'NONE',  ( 11.29080664838499182, -35.94265729135299381, 6.000000000000000000 ) ) ;
#38312=CARTESIAN_POINT ( 'NONE',  ( 15.86194215377555494, 10.70901654444746676, -2.668816250362950449 ) ) ;
#38317=CARTESIAN_POINT ( 'NONE',  ( -17.27251170661583402, 3.729367930467589076, 6.000000000000000000 ) ) ;
#38319=CARTESIAN_POINT ( 'NONE',  ( 87.04213330793400871, 0.5878691963681530464, -4.891134986362597914 ) ) ;
#38320=CARTESIAN_POINT ( 'NONE',  ( 26.98641761431236930, 1.293889648236598022, -5.140668381306381818 ) ) ;
#38326=CARTESIAN_POINT ( 'NONE',  ( 37.11166072668748228, -2.778356675396603581, -5.998012396607308894 ) ) ;
#38327=CARTESIAN_POINT ( 'NONE',  ( -70.92837670882107659, -56.35932253828836025, -10.00000000000000888 ) ) ;
#38335=CARTESIAN_POINT ( 'NONE',  ( 32.50899170535470262, -3.013835995739015061, 5.280212407192823143 ) ) ;
#38338=DIRECTION ( 'NONE',  ( -0.000000000000000000, 1.000000000000000000, -0.000000000000000000 ) ) ;
#38345=DIRECTION ( 'NONE',  ( 0.000000000000000000, 1.000000000000000000, 0.000000000000000000 ) ) ;
#38346=CARTESIAN_POINT ( 'NONE',  ( 23.90227964751484535, 3.010637336354621496, 3.787656613205743650 ) ) ;
#38352=CARTESIAN_POINT ( 'NONE',  ( 24.75663416313030751, 3.018532308770745409, 3.353834330914950090 ) ) ;
#38359=CARTESIAN_POINT ( 'NONE',  ( 23.59559651940404024, 0.4311816695734068117, 5.519554995405929532 ) ) ;
#38363=CARTESIAN_POINT ( 'NONE',  ( -69.92837670882107659, -0.7829914368874778541, 9.949874371066204759 ) ) ;
#38366=CARTESIAN_POINT ( 'NONE',  ( 25.20438522764541744, -3.119311913904994515, 5.422531462276817038 ) ) ;
#38369=CARTESIAN_POINT ( 'NONE',  ( -74.57913178212034211, -4.413113548761699256, 9.314603197924022027 ) ) ;
#38370=CARTESIAN_POINT ( 'NONE',  ( 26.76647965857537415, 0.8302664925678825414, -4.383954519114094950 ) ) ;
#38371=CARTESIAN_POINT ( 'NONE',  ( -77.92837670882107659, 2.429809908903242555, -12.50000000000000000 ) ) ;
#38373=CARTESIAN_POINT ( 'NONE',  ( 33.45639490703039343, -3.830543181052060486, -5.092503944725620180 ) ) ;
#38376=CARTESIAN_POINT ( 'NONE',  ( 22.27827011423021375, 5.092264179490945786, 3.633461677088038577 ) ) ;
#38380=CIRCLE ( 'NONE', #9434, 12.38600677260393113 ) ;
#38381=CARTESIAN_POINT ( 'NONE',  ( 20.40287464304303100, 10.75613383955523616, -2.500000000000000000 ) ) ;
#38383=CARTESIAN_POINT ( 'NONE',  ( 24.44373853437086197, 1.125249206679775238, -4.746398584013702404 ) ) ;
#38384=CARTESIAN_POINT ( 'NONE',  ( 33.50539668211418842, -0.3143895519534527505, -5.031603207882493045 ) ) ;
#38385=LINE ( 'NONE', #25850, #3906 ) ;
#38392=CARTESIAN_POINT ( 'NONE',  ( 86.35968278939613185, 0.3242946576005459325, -6.017936684944984016 ) ) ;
#38399=DIRECTION ( 'NONE',  ( -1.000000000000000000, -5.551115123125787751E-14, 0.000000000000000000 ) ) ;
#38402=DIRECTION ( 'NONE',  ( -1.000000000000000000, 0.000000000000000000, 0.000000000000000000 ) ) ;
#38407=FACE_OUTER_BOUND ( 'NONE', #6305, .T. ) ;
#38412=CARTESIAN_POINT ( 'NONE',  ( 25.95070172733332825, 1.815565124465190250, 4.256632643280088502 ) ) ;
#38415=CARTESIAN_POINT ( 'NONE',  ( 33.78722970661161185, -4.852430101419790809, -3.455127649274125190 ) ) ;
#38416=CARTESIAN_POINT ( 'NONE',  ( 24.73483262695019391, 3.010241890163435574, -3.394196563057135130 ) ) ;
#38421=CARTESIAN_POINT ( 'NONE',  ( -73.53810101549979095, -0.8611987601447699259, -10.86982216486306640 ) ) ;
#38425=CARTESIAN_POINT ( 'NONE',  ( 84.36871573755720988, 2.689384369868815128, -2.914620128191189874 ) ) ;
#38426=DIRECTION ( 'NONE',  ( -0.000000000000000000, 0.000000000000000000, 1.000000000000000000 ) ) ;
#38428=CARTESIAN_POINT ( 'NONE',  ( 21.54803796295231777, 7.333299173607420229, 1.920888206966631984 ) ) ;
#38434=CARTESIAN_POINT ( 'NONE',  ( 36.64647822751152262, -2.460832023537397273, 5.925967244464915851 ) ) ;
#38435=AXIS2_PLACEMENT_3D ( 'NONE', #26449, #7497, #10977 ) ;
#38438=CARTESIAN_POINT ( 'NONE',  ( 85.11099552155531001, 2.757014815357352155, -1.204572545719858834 ) ) ;
#38444=ORIENTED_EDGE ( 'NONE', *, *, #7448, .T. ) ;
#38448=CARTESIAN_POINT ( 'NONE',  ( -73.55543068772023219, -3.221851483746068112, 9.649644320831473721 ) ) ;
#38451=( BOUNDED_SURFACE ( )  B_SPLINE_SURFACE ( 3, 2, ( 
 ( #33688, #1779, #29968 ),
 ( #5467, #15130, #20693 ),
 ( #30386, #36354, #17800 ),
 ( #40242, #18007, #39848 ),
 ( #30171, #36959, #20906 ),
 ( #40044, #8739, #5058 ),
 ( #11615, #1992, #30596 ),
 ( #24195, #27085, #17591 ),
 ( #11211, #11819, #11413 ),
 ( #27686, #36754, #21322 ),
 ( #12026, #23980, #24605 ),
 ( #2404, #36552, #20484 ),
 ( #37160, #8330, #33491 ),
 ( #14926, #26879, #27495 ),
 ( #33068, #4852, #14310 ),
 ( #39422, #8121, #28304 ),
 ( #22356, #21731, #3630 ),
 ( #31204, #5881, #34719 ),
 ( #321, #31006, #22147 ),
 ( #12244, #34923, #31815 ),
 ( #21531, #6699, #34313 ),
 ( #3232, #9567, #31611 ),
 ( #37758, #19047, #19248 ),
 ( #37560, #28719, #15751 ),
 ( #122, #9155, #40435 ),
 ( #6082, #25229, #16155 ),
 ( #25427, #12860, #37968 ),
 ( #531, #9355, #3434 ),
 ( #18617, #9773, #3024 ),
 ( #18418, #13066, #6498 ),
 ( #15544, #28098, #12654 ),
 ( #25627, #24818, #15947 ),
 ( #28511, #8946, #34107 ),
 ( #2811, #15333, #40652 ),
 ( #27888, #37360, #12454 ),
 ( #25023, #21936, #34510 ),
 ( #6286, #18835, #31407 ),
 ( #38573, #6895, #23345 ),
 ( #35716, #4426, #10769 ),
 ( #32026, #13677, #725 ),
 ( #16950, #38172, #32229 ),
 ( #22555, #22956, #32631 ),
 ( #4618, #3831, #38779 ),
 ( #38369, #9975, #35118 ),
 ( #16351, #13876, #20245 ),
 ( #35325, #1143, #7492 ),
 ( #16547, #4221, #28924 ),
 ( #10575, #35917, #23149 ),
 ( #20052, #19452, #13266 ),
 ( #19657, #38970, #4029 ),
 ( #7696, #25834, #1530 ),
 ( #26247, #35519, #32827 ),
 ( #26443, #10379, #29720 ),
 ( #17148, #14064, #10166 ),
 ( #22757, #7290, #7093 ),
 ( #29128, #29528, #1340 ),
 ( #931, #13465, #26039 ),
 ( #19853, #32423, #16742 ),
 ( #29326, #26838, #29919 ),
 ( #11571, #20647, #20857 ),
 ( #21071, #36310, #2561 ),
 ( #8282, #33024, #2354 ),
 ( #17752, #8695, #27041 ),
 ( #26641, #39175, #39585 ),
 ( #30133, #40001, #4814 ),
 ( #23937, #24146, #1948 ) ),
 .UNSPECIFIED., .F., .F., .F. ) 
 B_SPLINE_SURFACE_WITH_KNOTS ( ( 4, 2, 2, 2, 2, 2, 2, 2, 2, 2, 2, 2, 2, 2, 2, 2, 2, 2, 2, 2, 2, 2, 2, 2, 2, 2, 2, 2, 2, 2, 2, 2, 4 ),
 ( 3, 3 ),
 ( 0.000000000000000000, 0.002658035264796820320, 0.003987052897195230913, 0.005316070529593640639, 0.006645088161992051233, 0.007974105794390461827, 0.009303123426788871553, 0.009967632242988076416, 0.01063214105918728128, 0.01196115869158569101, 0.01262566750778489760, 0.01329017632398410247, 0.01461919395638251393, 0.01594821158878092365, 0.01727722922117933338, 0.01860624685357774311, 0.01993526448597615283, 0.02126428211837456256, 0.02392231738317138201, 0.02525133501556979521, 0.02658035264796820493, 0.02790937028036661466, 0.02923838791276502785, 0.03056740554516343758, 0.03189642317756184731, 0.03322544080996026050, 0.03455445844235866676, 0.03588347607475707302, 0.03721249370715548621, 0.03854151133955389941, 0.03987052897195230566, 0.04119954660435071192, 0.04252856423674912512 ),
 ( 0.000000000000000000, 1.000000000000000000 ),
 .UNSPECIFIED. ) 
 GEOMETRIC_REPRESENTATION_ITEM ( )  RATIONAL_B_SPLINE_SURFACE ( (
 ( 1.000000000000000000, 0.7441515679388579496, 1.000000000000000000),
 ( 1.000000000000000000, 0.7418889564077462140, 1.000000000000000000),
 ( 1.000000000000000000, 0.7352412587068134497, 1.000000000000000000),
 ( 1.000000000000000000, 0.7200556229443167977, 1.000000000000000000),
 ( 1.000000000000000000, 0.7140806601001210563, 1.000000000000000000),
 ( 1.000000000000000000, 0.7009386729189606147, 1.000000000000000000),
 ( 1.000000000000000000, 0.6938174132529958404, 1.000000000000000000),
 ( 1.000000000000000000, 0.6790697772413124556, 1.000000000000000000),
 ( 1.000000000000000000, 0.6714408432011916839, 1.000000000000000000),
 ( 1.000000000000000000, 0.6564065633759171847, 1.000000000000000000),
 ( 1.000000000000000000, 0.6489510379847600596, 1.000000000000000000),
 ( 1.000000000000000000, 0.6356113203842299608, 1.000000000000000000),
 ( 1.000000000000000000, 0.6296912164606264239, 1.000000000000000000),
 ( 1.000000000000000000, 0.6225417645797769461, 1.000000000000000000),
 ( 1.000000000000000000, 0.6204465321787280274, 1.000000000000000000),
 ( 1.000000000000000000, 0.6169216871892950760, 1.000000000000000000),
 ( 1.000000000000000000, 0.6155016171862526253, 1.000000000000000000),
 ( 1.000000000000000000, 0.6123816062328042431, 1.000000000000000000),
 ( 1.000000000000000000, 0.6117967163037434375, 1.000000000000000000),
 ( 1.000000000000000000, 0.6130028206688593606, 1.000000000000000000),
 ( 1.000000000000000000, 0.6137491082589734415, 1.000000000000000000),
 ( 1.000000000000000000, 0.6158696746842220460, 1.000000000000000000),
 ( 1.000000000000000000, 0.6172499807807707572, 1.000000000000000000),
 ( 1.000000000000000000, 0.6220975276951665744, 1.000000000000000000),
 ( 1.000000000000000000, 0.6262835279352212403, 1.000000000000000000),
 ( 1.000000000000000000, 0.6355396176620391469, 1.000000000000000000),
 ( 1.000000000000000000, 0.6406497905274252114, 1.000000000000000000),
 ( 1.000000000000000000, 0.6505234917001551098, 1.000000000000000000),
 ( 1.000000000000000000, 0.6552943981022679720, 1.000000000000000000),
 ( 1.000000000000000000, 0.6637656571438727005, 1.000000000000000000),
 ( 1.000000000000000000, 0.6674871567836762054, 1.000000000000000000),
 ( 1.000000000000000000, 0.6731590004692020734, 1.000000000000000000),
 ( 1.000000000000000000, 0.6751296496122961566, 1.000000000000000000),
 ( 1.000000000000000000, 0.6771305984922478816, 1.000000000000000000),
 ( 1.000000000000000000, 0.6771548257842952001, 1.000000000000000000),
 ( 1.000000000000000000, 0.6742147169802384932, 1.000000000000000000),
 ( 1.000000000000000000, 0.6682671589301644177, 1.000000000000000000),
 ( 1.000000000000000000, 0.6555315094090650163, 1.000000000000000000),
 ( 1.000000000000000000, 0.6507284898546285001, 1.000000000000000000),
 ( 1.000000000000000000, 0.6409367973921450412, 1.000000000000000000),
 ( 1.000000000000000000, 0.6359230196329027640, 1.000000000000000000),
 ( 1.000000000000000000, 0.6266085828807440583, 1.000000000000000000),
 ( 1.000000000000000000, 0.6223160178622464400, 1.000000000000000000),
 ( 1.000000000000000000, 0.6158161838050073555, 1.000000000000000000),
 ( 1.000000000000000000, 0.6135607247596366332, 1.000000000000000000),
 ( 1.000000000000000000, 0.6117889963409239851, 1.000000000000000000),
 ( 1.000000000000000000, 0.6123161496792929315, 1.000000000000000000),
 ( 1.000000000000000000, 0.6163584728649634803, 1.000000000000000000),
 ( 1.000000000000000000, 0.6198375735205692294, 1.000000000000000000),
 ( 1.000000000000000000, 0.6292699336656990550, 1.000000000000000000),
 ( 1.000000000000000000, 0.6352691617163160887, 1.000000000000000000),
 ( 1.000000000000000000, 0.6485718343924502527, 1.000000000000000000),
 ( 1.000000000000000000, 0.6558929686343136778, 1.000000000000000000),
 ( 1.000000000000000000, 0.6709892557901798726, 1.000000000000000000),
 ( 1.000000000000000000, 0.6787899122752630854, 1.000000000000000000),
 ( 1.000000000000000000, 0.6936905356355238528, 1.000000000000000000),
 ( 1.000000000000000000, 0.7008379245427935889, 1.000000000000000000),
 ( 1.000000000000000000, 0.7139594056183991011, 1.000000000000000000),
 ( 1.000000000000000000, 0.7199647099235089165, 1.000000000000000000),
 ( 1.000000000000000000, 0.7301796029319667092, 1.000000000000000000),
 ( 1.000000000000000000, 0.7343899733826660947, 1.000000000000000000),
 ( 1.000000000000000000, 0.7408103714601322887, 1.000000000000000000),
 ( 1.000000000000000000, 0.7430216292999781702, 1.000000000000000000),
 ( 1.000000000000000000, 0.7452812010865806913, 1.000000000000000000),
 ( 1.000000000000000000, 0.7453214615320080672, 1.000000000000000000),
 ( 1.000000000000000000, 0.7442417417348949904, 1.000000000000000000) ) ) 
 REPRESENTATION_ITEM ( '' )  SURFACE ( )  );
#38453=CARTESIAN_POINT ( 'NONE',  ( 23.12586401754871446, 1.482052930854636186, 5.229025453252686972 ) ) ;
#38457=CARTESIAN_POINT ( 'NONE',  ( 14.74962925723565021, 13.05063958597602713, -2.500338280337093710 ) ) ;
#38458=CARTESIAN_POINT ( 'NONE',  ( 85.51486067931016066, 2.303374301570278782, 3.104493111481445133 ) ) ;
#38463=CARTESIAN_POINT ( 'NONE',  ( 23.65021474120684175, 3.294044046464493114, -3.628962476493511335 ) ) ;
#38465=CARTESIAN_POINT ( 'NONE',  ( -71.92837670882109080, -0.6505656586640776728, 5.916079783099611689 ) ) ;
#38467=CARTESIAN_POINT ( 'NONE',  ( 21.85643539959777826, -3.517407513333692837, -12.34883488727242806 ) ) ;
#38468=AXIS2_PLACEMENT_3D ( 'NONE', #28343, #22390, #5915 ) ;
#38469=CARTESIAN_POINT ( 'NONE',  ( 17.09215160922207133, 14.51084972820098606, -1.912535534561643491 ) ) ;
#38472=CARTESIAN_POINT ( 'NONE',  ( 87.06807637922989329, 0.009568187950425697044, -5.830412620327568796 ) ) ;
#38479=CARTESIAN_POINT ( 'NONE',  ( 32.30199181244099549, -3.779839205847876027, 4.859909891667491877 ) ) ;
#38480=CARTESIAN_POINT ( 'NONE',  ( 36.63338369844979781, -3.080224374057493719, -5.923923526512606230 ) ) ;
#38482=CARTESIAN_POINT ( 'NONE',  ( 84.37976216279319885, 2.675842969773557734, -2.958831758778651455 ) ) ;
#38483=CARTESIAN_POINT ( 'NONE',  ( -73.12195409265169133, 0.3003155719458506789, 10.93237219782067093 ) ) ;
#38487=CARTESIAN_POINT ( 'NONE',  ( 33.45208957067621469, -3.251134754649326553, 5.427405637984302089 ) ) ;
#38488=EDGE_CURVE ( 'NONE', #38156, #9413, #9067, .T. ) ;
#38491=CARTESIAN_POINT ( 'NONE',  ( 36.68486169653590423, -1.915814949631118758, 5.803682713086825373 ) ) ;
#38494=CARTESIAN_POINT ( 'NONE',  ( 87.91312586971599785, -2.495764367860345612, 0.6122158967995121603 ) ) ;
#38496=AXIS2_PLACEMENT_3D ( 'NONE', #28787, #7156, #23015 ) ;
#38503=CARTESIAN_POINT ( 'NONE',  ( 22.25877217673135888, 4.971410982095481046, 3.249134972655711273 ) ) ;
#38517=CARTESIAN_POINT ( 'NONE',  ( 27.43879703630890887, 0.9604363013853572939, -4.488885905966782275 ) ) ;
#38520=CARTESIAN_POINT ( 'NONE',  ( 29.86640044794213011, -3.433240980530400499, 4.572246828724481738 ) ) ;
#38524=CARTESIAN_POINT ( 'NONE',  ( -70.66609929912286248, -21.75673952224967422, 9.997285688091769984 ) ) ;
#38525=EDGE_CURVE ( 'NONE', #17878, #35921, #9028, .T. ) ;
#38530=CARTESIAN_POINT ( 'NONE',  ( 34.51608426288976972, -1.013665949057833915, -5.504871762502034471 ) ) ;
#38537=CARTESIAN_POINT ( 'NONE',  ( 14.77315594796849574, 13.19392823276453441, -2.500000000000005773 ) ) ;
#38539=CARTESIAN_POINT ( 'NONE',  ( 31.86209868568754544, -0.1501604454850196113, 5.152680217172298960 ) ) ;
#38546=CARTESIAN_POINT ( 'NONE',  ( 23.25558064308254558, 3.168631396969136649, 3.922402285246370024 ) ) ;
#38551=CARTESIAN_POINT ( 'NONE',  ( 24.40511021066326336, 3.163327161787246933, 3.272226049981214135 ) ) ;
#38555=ORIENTED_EDGE ( 'NONE', *, *, #33408, .F. ) ;
#38557=CARTESIAN_POINT ( 'NONE',  ( 23.59267417321471427, 0.4265057547314817232, 5.522590887384096092 ) ) ;
#38570=CARTESIAN_POINT ( 'NONE',  ( 22.63837051618441620, -3.414681707391253429, 8.302592004085083133 ) ) ;
#38573=CARTESIAN_POINT ( 'NONE',  ( -72.46102572804289821, -1.248168175329565255, 9.882956611723583862 ) ) ;
#38574=CARTESIAN_POINT ( 'NONE',  ( 26.76858707236903712, 0.8094380621706002144, -4.384283432004588477 ) ) ;
#38577=CARTESIAN_POINT ( 'NONE',  ( 25.01091293555841233, 3.329590545877085805, 1.936828124349011526 ) ) ;
#38578=CARTESIAN_POINT ( 'NONE',  ( 36.68540230263305801, -1.915051275179609380, -5.803267592155077814 ) ) ;
#38580=CARTESIAN_POINT ( 'NONE',  ( 8.290806648384990041, -35.94265729135299381, -2.500000000000000444 ) ) ;
#38587=CARTESIAN_POINT ( 'NONE',  ( 21.89213072762610679, 0.4842128809993961336, -7.752462955432138259 ) ) ;
#38588=CARTESIAN_POINT ( 'NONE',  ( 30.52514172340196907, 0.8294708601856738417, -4.428110633612789115 ) ) ;
#38597=CARTESIAN_POINT ( 'NONE',  ( 84.80660115723814840, 2.320002077609508717, 4.142190259225312587 ) ) ;
#38600=CARTESIAN_POINT ( 'NONE',  ( -74.96765229735504477, 7.901165263090923929, -10.49888776350863040 ) ) ;
#38609=CARTESIAN_POINT ( 'NONE',  ( 33.77557131158557269, -4.800086674967288580, 3.580757159575843396 ) ) ;
#38611=CARTESIAN_POINT ( 'NONE',  ( -83.92837670882109080, 2.429809908903242999, -12.50000000000000000 ) ) ;
#38615=B_SPLINE_CURVE_WITH_KNOTS ( 'NONE', 3,
 ( #21814, #3109, #15629, #28178, #3, #12534, #25316, #9441, #6376, #18924, #3315, #37847, #9651, #22237, #639, #31929, #3736, #19566, #10281, #19356, #22664, #16259, #25740, #38281, #16460, #10078, #29033, #35229, #837, #13369, #39023, #3688, #6952, #4277, #23202, #38231, #10028, #16801, #22611, #35179, #32090, #3894, #16409, #28984, #787, #8133, #17205, #33696, #20704, #14117, #29976, #26696, #40055, #39231, #29771 ),
 .UNSPECIFIED., .F., .F.,
 ( 4, 1, 1, 1, 1, 2, 2, 1, 1, 1, 1, 1, 1, 2, 2, 1, 1, 1, 1, 2, 2, 1, 1, 1, 1, 1, 1, 1, 1, 2, 2, 1, 1, 1, 1, 1, 1, 2, 2, 1, 1, 1, 4 ),
 ( 0.000000000000000000, 0.08647898122975995749, 0.1080987265372002210, 0.1189085991909197421, 0.1243135355177801410, 0.1249891525586373786, 0.1251580568188523090, 0.1253269610790672672, 0.1256647695994971836, 0.1270160036812162940, 0.1297184718446550700, 0.1729579624596754572, 0.1837678351134310606, 0.1864703032768696978, 0.1891727714403083349, 0.1945777077671867750, 0.2161974530747031165, 0.2378171983822194580, 0.2486270710359776148, 0.2499783051176977522, 0.2503161136381279461, 0.2506539221585581401, 0.2513295391994198602, 0.2540320073628683506, 0.2594369436897639436, 0.3459159249200896569, 0.3675356702276709187, 0.3729406065545658455, 0.3742918406362890638, 0.3749674576771503398, 0.3753052661975809223, 0.3756430747180115048, 0.3783455428814596622, 0.3891554155352489608, 0.4323949061504016034, 0.4756343967655542460, 0.4972541420731305672, 0.4999566102365775588, 0.5013078443183011101, 0.5026590784000246614, 0.5080640147269191997, 0.5188738873807084984, 0.6918318498413339457 ),
 .UNSPECIFIED. ) ;
#38616=LINE ( 'NONE', #18076, #26553 ) ;
#38617=CARTESIAN_POINT ( 'NONE',  ( 21.85643539959778892, -12.39743456692229628, -10.22857181343751520 ) ) ;
#38620=CARTESIAN_POINT ( 'NONE',  ( 23.75175095104303225, 3.571146634990261415, -3.154077189411854665 ) ) ;
#38629=CARTESIAN_POINT ( 'NONE',  ( -72.05796840954714355, -0.01142228043888725460, -9.936409781712523426 ) ) ;
#38633=CARTESIAN_POINT ( 'NONE',  ( 87.90619863186083194, -2.144287391213948624, -2.780224877855328014 ) ) ;
#38634=LINE ( 'NONE', #28981, #28586 ) ;
#38642=CARTESIAN_POINT ( 'NONE',  ( 34.77309709234581447, -3.162889125028089055, 5.633580810428385099 ) ) ;
#38643=CARTESIAN_POINT ( 'NONE',  ( 85.93841924537714760, 1.827613216861550205, 4.619486236290579306 ) ) ;
#38656=CARTESIAN_POINT ( 'NONE',  ( 24.94969356037918828, 3.454325501316659608, -1.299993212727057479 ) ) ;
#38657=CARTESIAN_POINT ( 'NONE',  ( 25.02958830711385829, 2.171333288770124881, 4.140797983151394135 ) ) ;
#38663=CARTESIAN_POINT ( 'NONE',  ( 85.37176321662279577, 2.464108163476022018, 2.465283846017703340 ) ) ;
#38668=CARTESIAN_POINT ( 'NONE',  ( 23.01179671817061845, 3.457809282331678169, -3.829885419034514626 ) ) ;
#38670=CARTESIAN_POINT ( 'NONE',  ( -71.80167951437309171, -0.2784832644296509896, 5.936322957303396208 ) ) ;
#38671=ORIENTED_EDGE ( 'NONE', *, *, #30559, .T. ) ;
#38672=CARTESIAN_POINT ( 'NONE',  ( 21.85643539959776049, -12.91308397612913161, -3.835380774090566103 ) ) ;
#38673=CARTESIAN_POINT ( 'NONE',  ( 21.26333942293403467, 9.593021065652562740, 2.042309770454811435 ) ) ;
#38678=CARTESIAN_POINT ( 'NONE',  ( 85.76961320806377387, 1.955528254085527662, 4.811735575706960866 ) ) ;
#38680=CARTESIAN_POINT ( 'NONE',  ( -81.73423472054517447, -5.610403504835165478, 1.501100129317205489 ) ) ;
#38682=CARTESIAN_POINT ( 'NONE',  ( 23.84321753579541081, -2.715127441814079834, 3.927708765492790022 ) ) ;
#38684=CARTESIAN_POINT ( 'NONE',  ( 33.95462147649067930, -3.429569851476566011, -5.493391470225660989 ) ) ;
#38685=CARTESIAN_POINT ( 'NONE',  ( 36.78903429469688291, -3.040829720014896154, -5.948216566480869716 ) ) ;
#38687=CARTESIAN_POINT ( 'NONE',  ( 84.11150843037509617, 3.004017517549075311, -0.5155748138339447673 ) ) ;
#38690=CARTESIAN_POINT ( 'NONE',  ( 28.33744289130897442, -3.843786207261427723, 4.468846400079240055 ) ) ;
#38694=CARTESIAN_POINT ( 'NONE',  ( 36.87144894572305986, -2.086539832640053049, 5.863895186686348460 ) ) ;
#38699=CARTESIAN_POINT ( 'NONE',  ( 87.07401102672321258, -1.450421667693342798, 4.784145908967932570 ) ) ;
#38700=B_SPLINE_CURVE_WITH_KNOTS ( 'NONE', 5,
 ( #24985, #19207, #37519, #9119, #16113, #6856, #31569, #34470 ),
 .UNSPECIFIED., .F., .F.,
 ( 6, 2, 6 ),
 ( 0.000000000000000000, 0.5000000000000000000, 1.000000000000000000 ),
 .UNSPECIFIED. ) ;
#38708=CARTESIAN_POINT ( 'NONE',  ( 23.18984300410216903, 3.594347016654975135, 3.590839796171831910 ) ) ;
#38710=CIRCLE ( 'NONE', #24251, 15.73502530973474478 ) ;
#38721=CARTESIAN_POINT ( 'NONE',  ( 24.17959102519681736, 2.679401842515043430, -3.980207983737488409 ) ) ;
#38726=CARTESIAN_POINT ( 'NONE',  ( 85.94962389285764459, 1.815027625006768730, -4.252598035848374813 ) ) ;
#38727=CARTESIAN_POINT ( 'NONE',  ( 31.71671097226645131, -1.585248588153130855, -6.002663613118158992 ) ) ;
#38733=CARTESIAN_POINT ( 'NONE',  ( 35.97288949415787584, -1.842364254675447066, -5.810895595490718435 ) ) ;
#38738=FACE_OUTER_BOUND ( 'NONE', #2840, .T. ) ;
#38743=VERTEX_POINT ( 'NONE', #24115 ) ;
#38744=CARTESIAN_POINT ( 'NONE',  ( 37.14562426157099395, -2.766377302884501344, 6.000546555870065468 ) ) ;
#38745=B_SPLINE_CURVE_WITH_KNOTS ( 'NONE', 3,
 ( #7351, #19515, #20299, #35972, #4279, #994, #17005, #25894, #32685, #16602, #19908, #10631 ),
 .UNSPECIFIED., .F., .F.,
 ( 4, 2, 2, 2, 2, 4 ),
 ( 0.0002778957232965137826, 0.001623504286842941766, 0.002969112850389369479, 0.005660329977482225772, 0.008351547104575083799, 0.01104276423166794183 ),
 .UNSPECIFIED. ) ;
#38752=CARTESIAN_POINT ( 'NONE',  ( 30.80517229667822932, -3.346871776499003470, 4.960489240099761332 ) ) ;
#38753=CARTESIAN_POINT ( 'NONE',  ( 84.80999693743234502, 2.128580961947359462, -4.467585834308593462 ) ) ;
#38755=EDGE_CURVE ( 'NONE', #10538, #24333, #9433, .T. ) ;
#38758=DIRECTION ( 'NONE',  ( 1.000000000000000000, 0.000000000000000000, 0.000000000000000000 ) ) ;
#38760=EDGE_CURVE ( 'NONE', #3867, #833, #11342, .T. ) ;
#38761=CARTESIAN_POINT ( 'NONE',  ( 21.98982740266793456, 5.607487361672509607, 3.095612616452370514 ) ) ;
#38767=CARTESIAN_POINT ( 'NONE',  ( 25.38030252091800065, 0.7242675303424039868, 4.602055157131172969 ) ) ;
#38772=CARTESIAN_POINT ( 'NONE',  ( -81.90664279350785648, 11.45717611192839591, 0.6911394749367770762 ) ) ;
#38776=CARTESIAN_POINT ( 'NONE',  ( 22.76577552469399990, -5.388071312449273620, 6.143773694815460651 ) ) ;
#38779=CARTESIAN_POINT ( 'NONE',  ( -75.05072613888007993, -3.128072587506124602, 10.46819543870325475 ) ) ;
#38780=CARTESIAN_POINT ( 'NONE',  ( 21.73379047671751962, 0.2086737143224493274, -9.125075291706918890 ) ) ;
#38783=CARTESIAN_POINT ( 'NONE',  ( 23.03325835086280193, 4.443132776864800348, 2.273497529138607476 ) ) ;
#38786=CARTESIAN_POINT ( 'NONE',  ( 35.73088790136473136, -1.303468173786156870, -5.537281536383253489 ) ) ;
#38787=CARTESIAN_POINT ( 'NONE',  ( 30.58053394437551020, -3.206738070849787015, -4.963780911168087506 ) ) ;
#38797=CARTESIAN_POINT ( 'NONE',  ( 86.59537683758360060, -0.3992097724244685342, -5.811584838773467432 ) ) ;
#38798=EDGE_CURVE ( 'NONE', #32959, #29224, #19125, .T. ) ;
#38801=B_SPLINE_SURFACE_WITH_KNOTS ( 'NONE', 5, 3, ( 
 ( #40152, #36459, #21434, #24511, #30493, #4765, #2303, #14615, #30284, #4969, #36661, #8649, #21025, #14825, #17496, #29877, #26798, #27391 ),
 ( #5576, #14422, #21226, #5173, #39335, #1902, #36867, #33401, #30707, #24303, #26991, #33797, #20804, #2514, #17705, #11126, #2099, #432 ),
 ( #3533, #37267, #5783, #24718, #30912, #9062, #28004, #12359, #28201, #12972, #15656, #33, #37465, #9884, #15858, #28629, #37873, #22050 ),
 ( #9463, #34420, #6192, #15445, #27796, #3138, #9678, #28415, #6606, #21638, #40348, #18321, #34219, #21842, #5989, #34830, #25540, #18526 ),
 ( #12760, #25339, #15240, #6400, #38082, #31111, #19153, #31516, #12145, #25131, #18738, #18952, #34627, #31719, #37663, #2923, #12560, #34010 ),
 ( #31316, #3339, #2720, #40546, #222, #24931, #9262, #16058, #22263, #6803, #16258, #19758, #13368, #25739, #35822, #1042, #638, #19355 ),
 ( #16646, #32337, #35027, #10077, #13575, #38682, #39078, #4131, #26542, #22460, #13177, #31928, #22661, #38280, #32143, #10280, #4332, #19951 ),
 ( #3735, #7000, #22857, #28831, #7599, #20152, #29232, #26148, #17049, #13973, #35228, #19565, #32531, #13783, #7398, #3940, #38883, #16852 ) ),
 .UNSPECIFIED., .F., .F., .F.,
 ( 6, 2, 6 ),
 ( 4, 1, 1, 1, 1, 1, 1, 1, 1, 1, 1, 1, 1, 1, 1, 4 ),
 ( 0.000000000000000000, 0.5000000000000000000, 1.000000000000000000 ),
 ( 0.006359509864058362355, 0.008899940506546142119, 0.01165379832700513818, 0.01387926207582779702, 0.01684654707425800937, 0.01907201082308066648, 0.02092656394709954681, 0.02241020644631465386, 0.02352293832072598415, 0.02445021488273542778, 0.02519203613234298131, 0.02574840206954863778, 0.02630476800675430812, 0.02686113394395997153, 0.02741749988116563841, 0.02797386581837130182 ),
 .UNSPECIFIED. ) ;
#38804=LINE ( 'NONE', #6919, #10047 ) ;
#38805=EDGE_CURVE ( 'NONE', #7875, #19840, #22632, .T. ) ;
#38812=CARTESIAN_POINT ( 'NONE',  ( 33.89602703800589012, -5.455856628420105103, 0.7063779492982765751 ) ) ;
#38817=CARTESIAN_POINT ( 'NONE',  ( 25.33339624544385416, 2.111467966597739832, 4.160287193241738457 ) ) ;
#38820=CARTESIAN_POINT ( 'NONE',  ( 21.85643539959773207, -10.94848525941816675, -12.02078412262589602 ) ) ;
#38824=CARTESIAN_POINT ( 'NONE',  ( 0.000000000000000000, 13.37661300689600097, 6.000000000000000000 ) ) ;
#38825=CARTESIAN_POINT ( 'NONE',  ( -71.87765774115447925, 0.8657319589700837037, -9.955254003897318071 ) ) ;
#38841=CARTESIAN_POINT ( 'NONE',  ( 36.44708399685710987, -2.354165099489201385, 5.894846952403873352 ) ) ;
#38844=CARTESIAN_POINT ( 'NONE',  ( 85.23697547898807159, 2.562304445728192714, -3.499295437968926947 ) ) ;
#38850=ORIENTED_EDGE ( 'NONE', *, *, #40273, .T. ) ;
#38852=CARTESIAN_POINT ( 'NONE',  ( -76.67582790101022283, 10.73401294744294532, -8.185679464797956939 ) ) ;
#38853=CARTESIAN_POINT ( 'NONE',  ( -0.7996099067669091287, -29.56993018339339940, 6.000000000000000000 ) ) ;
#38856=CARTESIAN_POINT ( 'NONE',  ( 21.85643539959777115, -33.54387950140291963, -2.500000000000000000 ) ) ;
#38862=CARTESIAN_POINT ( 'NONE',  ( 23.62965689264861879, 0.6308181322251997791, 5.426430504554879519 ) ) ;
#38865=CARTESIAN_POINT ( 'NONE',  ( -8.400069747914319152, -0.9236158798217076749, -2.500000000000000000 ) ) ;
#38868=CARTESIAN_POINT ( 'NONE',  ( -70.92837670882107659, -65.19654454972992141, 6.000000000000002665 ) ) ;
#38870=ORIENTED_EDGE ( 'NONE', *, *, #29796, .T. ) ;
#38871=CARTESIAN_POINT ( 'NONE',  ( 22.08468009823165801, 5.143601559783003374, -3.328927790978220891 ) ) ;
#38874=CARTESIAN_POINT ( 'NONE',  ( 21.85643539959779957, 2.883972393613821072, 11.80804406839454046 ) ) ;
#38875=CARTESIAN_POINT ( 'NONE',  ( 21.69289330442630259, 6.888012688853828891, 2.083760414285012352 ) ) ;
#38876=CARTESIAN_POINT ( 'NONE',  ( 17.47038192185404171, 11.99840028321635010, 2.499999999999993339 ) ) ;
#38880=CARTESIAN_POINT ( 'NONE',  ( 86.11108918975101290, 0.7237488529220831301, -5.972109037703948076 ) ) ;
#38883=CARTESIAN_POINT ( 'NONE',  ( 14.75302088585650573, -5.978111498305209714, 2.508963731033090117 ) ) ;
#38884=CARTESIAN_POINT ( 'NONE',  ( 31.00341140003851947, -3.765336078302973899, 4.602883256886119767 ) ) ;
#38885=CARTESIAN_POINT ( 'NONE',  ( 26.27873381384168994, -2.762334174294334144, -4.307829983865710588 ) ) ;
#38886=CARTESIAN_POINT ( 'NONE',  ( 36.89680064675319926, -3.001266127369541792, -5.965036112058319517 ) ) ;
#38890=VERTEX_POINT ( 'NONE', #38856 ) ;
#38894=CARTESIAN_POINT ( 'NONE',  ( 32.98767453130994909, -3.051313967188787668, -5.354922439171034831 ) ) ;
#38897=CARTESIAN_POINT ( 'NONE',  ( 36.87099407197327139, -2.087246581719376604, 5.864208482129122046 ) ) ;
#38898=LINE ( 'NONE', #26365, #40253 ) ;
#38900=CARTESIAN_POINT ( 'NONE',  ( 86.32543542292076211, -0.3344508995418832842, 5.872725293628850096 ) ) ;
#38908=ORIENTED_EDGE ( 'NONE', *, *, #34628, .T. ) ;
#38909=CARTESIAN_POINT ( 'NONE',  ( 21.80921096923039215, 5.240870915421466769, 3.636790624354177215 ) ) ;
#38914=CARTESIAN_POINT ( 'NONE',  ( -8.400069747914319152, -0.9236158798217076749, 2.500000000000000000 ) ) ;
#38915=CARTESIAN_POINT ( 'NONE',  ( -70.92837670882107659, -65.19654454972992141, 0.000000000000000000 ) ) ;
#38917=CARTESIAN_POINT ( 'NONE',  ( 21.85265456426768083, 2.967629154170456474, -5.140454503935664832 ) ) ;
#38921=CARTESIAN_POINT ( 'NONE',  ( 24.21109618614866932, 2.662543315632417862, -3.985125126059221312 ) ) ;
#38926=CARTESIAN_POINT ( 'NONE',  ( 27.86875652909539980, 2.635651561731235493, 0.006556038081918813022 ) ) ;
#38932=CARTESIAN_POINT ( 'NONE',  ( 34.95695827223672580, -1.636488140955191017, -5.662276794249945233 ) ) ;
#38940=CARTESIAN_POINT ( 'NONE',  ( 36.78034191296258371, -2.229234730061248282, 5.922124464258623711 ) ) ;
#38948=CARTESIAN_POINT ( 'NONE',  ( 85.70685082919769116, 0.7924140212991883647, -5.893544677374721097 ) ) ;
#38951=VECTOR ( 'NONE', #31336, 1000.000000000000000 ) ;
#38956=CARTESIAN_POINT ( 'NONE',  ( 30.10909256169910364, -6.281120516155699995, -2.500000000000003997 ) ) ;
#38959=CARTESIAN_POINT ( 'NONE',  ( 26.74545741276980237, 0.9075178902881906318, 4.382577745642065814 ) ) ;
#38966=CARTESIAN_POINT ( 'NONE',  ( 26.66483005201559564, 2.460286195115170216, -3.284910328407702806 ) ) ;
#38970=CARTESIAN_POINT ( 'NONE',  ( -77.59921745286224848, -4.978234906976595653, 7.463450837162017848 ) ) ;
#38971=CARTESIAN_POINT ( 'NONE',  ( 21.73405303197773009, 0.2198190191631417822, -9.095604756692427628 ) ) ;
#38973=LINE ( 'NONE', #32635, #19042 ) ;
#38975=CARTESIAN_POINT ( 'NONE',  ( 33.11285781741161571, -0.1526090149532899065, -4.944069884480080113 ) ) ;
#38976=CARTESIAN_POINT ( 'NONE',  ( 30.19238557334687911, -2.952639005720375742, -4.918649992961978690 ) ) ;
#38991=CARTESIAN_POINT ( 'NONE',  ( 88.11323260317807637, -2.391772166421624490, 1.226420884133070599 ) ) ;
#38993=CARTESIAN_POINT ( 'NONE',  ( -81.15948786935145165, 10.50821952958543903, -3.991233431468591331 ) ) ;
#39002=CARTESIAN_POINT ( 'NONE',  ( 37.20094714327657215, -2.700959843830776919, 5.995701502916164216 ) ) ;
#39006=PLANE ( 'NONE',  #40301 ) ;
#39009=CARTESIAN_POINT ( 'NONE',  ( 21.85643539959777470, 7.942361823516107755, 9.319573164223585948 ) ) ;
#39014=CARTESIAN_POINT ( 'NONE',  ( -72.84104406220187400, 2.224784376281895071, -10.96219629948401675 ) ) ;
#39023=CARTESIAN_POINT ( 'NONE',  ( 35.89208955089092967, -2.095693868708802921, 5.808226646519337955 ) ) ;
#39034=CARTESIAN_POINT ( 'NONE',  ( 36.79789676325057712, -2.555714875043423095, 5.949599769038292685 ) ) ;
#39037=CARTESIAN_POINT ( 'NONE',  ( 85.38594790374143884, 2.393190016811436394, 3.957880923259903927 ) ) ;
#39040=CARTESIAN_POINT ( 'NONE',  ( 11.29080664838498649, 1.564594260697056104E-15, 6.000000000000000000 ) ) ;
#39042=VERTEX_POINT ( 'NONE', #27311 ) ;
#39043=CARTESIAN_POINT ( 'NONE',  ( -80.90861860399088812, 11.45717611192839591, 0.6283086135788885640 ) ) ;
#39044=CARTESIAN_POINT ( 'NONE',  ( 24.80856304665041634, -5.882444228827781174, -2.847423770020717892 ) ) ;
#39046=VECTOR ( 'NONE', #18137, 1000.000000000000000 ) ;
#39053=CARTESIAN_POINT ( 'NONE',  ( 22.80473035351651134, 0.6264772378953792353, 6.107320914785919541 ) ) ;
#39057=MANIFOLD_SOLID_BREP ( 'Cut-Extrude12', #13048 ) ;
#39060=CARTESIAN_POINT ( 'NONE',  ( 16.64247417493278292, 12.36459659649736409, 2.500000000000000888 ) ) ;
#39063=CARTESIAN_POINT ( 'NONE',  ( 24.29495741014220300, 3.123657746401501623, -3.464203466336227333 ) ) ;
#39065=CARTESIAN_POINT ( 'NONE',  ( -70.92837670882012446, 0.2170085631207802901, 6.000000000001379341 ) ) ;
#39067=CARTESIAN_POINT ( 'NONE',  ( 22.43090457150155004, 1.240285785788341810, -8.908344141805525140 ) ) ;
#39069=CARTESIAN_POINT ( 'NONE',  ( 18.14195397311778990, 13.68994309133309173, -3.806916816955884020 ) ) ;
#39070=CARTESIAN_POINT ( 'NONE',  ( 15.71701927994473813, 8.042377773714102673, 3.484701592660909508 ) ) ;
#39073=CARTESIAN_POINT ( 'NONE',  ( 87.19696342060086636, -0.1553247823698818142, -5.755373573531420206 ) ) ;
#39076=CARTESIAN_POINT ( 'NONE',  ( 24.12517570173129400, 0.5279882154166138930, -5.092426393238373983 ) ) ;
#39077=EDGE_CURVE ( 'NONE', #5343, #1678, #21973, .T. ) ;
#39078=CARTESIAN_POINT ( 'NONE',  ( 21.52094422564899290, -2.679845695244565729, 3.565261851052226483 ) ) ;
#39082=CARTESIAN_POINT ( 'NONE',  ( 16.01709162683344445, -3.387958631065356663, -2.706252541828943592 ) ) ;
#39083=CARTESIAN_POINT ( 'NONE',  ( 36.97911392267047148, -2.955988235745242498, -5.977883089519319348 ) ) ;
#39093=ORIENTED_EDGE ( 'NONE', *, *, #37075, .F. ) ;
#39094=CARTESIAN_POINT ( 'NONE',  ( 33.11343782431677596, -0.1514955757993836083, 4.942505121863887574 ) ) ;
#39097=CARTESIAN_POINT ( 'NONE',  ( 33.44054677433027933, -3.435571797939218186, 5.408185224205094954 ) ) ;
#39102=B_SPLINE_CURVE_WITH_KNOTS ( 'NONE', 3,
 ( #2704, #31094, #2905, #15424, #27984, #40531, #24912, #9245, #21822, #31701 ),
 .UNSPECIFIED., .F., .F.,
 ( 4, 2, 2, 2, 4 ),
 ( 0.001566336636202482393, 0.001957536639217858504, 0.002348736642233234181, 0.002739936645248610293, 0.003131136648263986404 ),
 .UNSPECIFIED. ) ;
#39105=CARTESIAN_POINT ( 'NONE',  ( -9.796229648729232409, -33.54387950140292673, -2.500000000000000000 ) ) ;
#39107=CARTESIAN_POINT ( 'NONE',  ( 23.93134969406609969, 3.254905450091994279, 3.508261123597265385 ) ) ;
#39115=CARTESIAN_POINT ( 'NONE',  ( 16.15910822604420716, -3.328347674494501973, -2.728417666820209586 ) ) ;
#39116=CARTESIAN_POINT ( 'NONE',  ( 22.37801635562015079, 5.219640035649274701, -3.555971675700331680 ) ) ;
#39118=CARTESIAN_POINT ( 'NONE',  ( 22.04692162351881279, 3.100284280110099377, -4.816771713714539160 ) ) ;
#39121=DIRECTION ( 'NONE',  ( -1.000000000000000000, -5.786005779812646808E-17, 0.000000000000000000 ) ) ;
#39122=CARTESIAN_POINT ( 'NONE',  ( 22.14407712215583501, 4.579442068576085489, -3.662516810078165097 ) ) ;
#39126=CARTESIAN_POINT ( 'NONE',  ( 86.56125476490799997, 1.128014799767447229, 4.962829853851403961 ) ) ;
#39127=CARTESIAN_POINT ( 'NONE',  ( 32.22946493318451644, -2.099509172777830557, 5.989391533279509794 ) ) ;
#39134=CARTESIAN_POINT ( 'NONE',  ( 21.48247305285511288, 3.876926268098481287, -3.508130033835277217 ) ) ;
#39140=AXIS2_PLACEMENT_3D ( 'NONE', #29696, #1508, #24742 ) ;
#39142=CARTESIAN_POINT ( 'NONE',  ( 35.10416124133201521, -1.272529116935883442, 5.608947908793178172 ) ) ;
#39149=CARTESIAN_POINT ( 'NONE',  ( 86.01040231118156498, 0.2354137643325349138, -5.999916684876917650 ) ) ;
#39155=CARTESIAN_POINT ( 'NONE',  ( 23.43424776407714916, 3.789913264566200368, 3.112445696235128345 ) ) ;
#39161=CARTESIAN_POINT ( 'NONE',  ( 24.12566071183585237, 0.5138664147065530319, 5.092652492612476323 ) ) ;
#39167=CIRCLE ( 'NONE', #14163, 2.500000000000000444 ) ;
#39172=CARTESIAN_POINT ( 'NONE',  ( 23.92067639343244778, 4.177307434159622801, 1.236145424036337426 ) ) ;
#39175=CARTESIAN_POINT ( 'NONE',  ( -80.93421692491173758, -5.699880070350716643, 0.2256805699841040458 ) ) ;
#39176=CARTESIAN_POINT ( 'NONE',  ( 25.39387711625591848, 0.7059127421703671468, -4.600211075182401466 ) ) ;
#39182=CARTESIAN_POINT ( 'NONE',  ( 34.78593673359796412, -3.774928924632479976, -5.430219759624750786 ) ) ;
#39183=CARTESIAN_POINT ( 'NONE',  ( -4.224659823956008253, -51.67615071827237472, 6.000000000000000000 ) ) ;
#39186=CARTESIAN_POINT ( 'NONE',  ( -71.02793705302472915, -48.61702805680359774, 6.000000000000004441 ) ) ;
#39192=ORIENTED_EDGE ( 'NONE', *, *, #28084, .F. ) ;
#39196=CARTESIAN_POINT ( 'NONE',  ( 86.38495421312710221, -0.4360953479145894263, -5.826368990767747391 ) ) ;
#39207=CARTESIAN_POINT ( 'NONE',  ( 23.63366851782300770, -3.140391636472827930, 3.778057570207932425 ) ) ;
#39210=CARTESIAN_POINT ( 'NONE',  ( 15.43177750874984433, 12.90197807773783367, -2.500000000000005773 ) ) ;
#39217=CARTESIAN_POINT ( 'NONE',  ( 21.85643539959774273, -10.14878426894149221, 9.991042268249278990 ) ) ;
#39221=CARTESIAN_POINT ( 'NONE',  ( 14.74185191083505231, -5.107022699585343162, 2.499999999999729106 ) ) ;
#39223=CARTESIAN_POINT ( 'NONE',  ( -79.25808045669066360, 11.47437878731752647, -5.548284614561191042 ) ) ;
#39226=CARTESIAN_POINT ( 'NONE',  ( 37.00891459296443031, -3.247065243002688284, -5.946827200946571246 ) ) ;
#39231=CARTESIAN_POINT ( 'NONE',  ( 28.38512348074436886, 0.6183906642395941011, 4.636583034612477228 ) ) ;
#39235=CARTESIAN_POINT ( 'NONE',  ( 87.35850478739605762, 0.2325057347401545127, 4.553521783490353414 ) ) ;
#39238=CARTESIAN_POINT ( 'NONE',  ( 34.77301380135100572, -3.165686779924592020, 5.633567810854094304 ) ) ;
#39241=CARTESIAN_POINT ( 'NONE',  ( 84.79809517660038409, 3.058972130929652256, -0.4747855469284483210 ) ) ;
#39247=CARTESIAN_POINT ( 'NONE',  ( -80.14709680133751135, 11.51107841541166010, -3.897538531476514745 ) ) ;
#39258=CARTESIAN_POINT ( 'NONE',  ( 24.77959113649616540, 1.432599100595700614, 4.541996434422298279 ) ) ;
#39265=CARTESIAN_POINT ( 'NONE',  ( 15.70794464946376223, 12.77956130056348272, 2.499999999999996003 ) ) ;
#39268=CARTESIAN_POINT ( 'NONE',  ( 23.70771619120949936, 3.501700497104693000, -3.333794200282627074 ) ) ;
#39272=CARTESIAN_POINT ( 'NONE',  ( 22.31814515643556263, 6.191369071892208531, -1.397765879422002033 ) ) ;
#39274=CARTESIAN_POINT ( 'NONE',  ( 21.89858680184175199, 3.819795205001112137, 2.126311674330342072 ) ) ;
#39275=CARTESIAN_POINT ( 'NONE',  ( 15.99304516048508340, 7.920163621858975489, 3.484773800358847318 ) ) ;
#39280=CARTESIAN_POINT ( 'NONE',  ( 84.36655727669636917, 3.025886916471207222, -1.294691096651311435 ) ) ;
#39286=CARTESIAN_POINT ( 'NONE',  ( 23.82868741420347192, -2.964576112339935232, -3.895336304183651510 ) ) ;
#39287=CARTESIAN_POINT ( 'NONE',  ( 37.04299532825181274, -2.892526904198844395, -5.987853327837934891 ) ) ;
#39288=DIRECTION ( 'NONE',  ( 0.1542073060391599970, 0.000000000000000000, 0.9880385148181951571 ) ) ;
#39289=CARTESIAN_POINT ( 'NONE',  ( 22.65759398342077091, 0.3095578120561012225, -6.438391604401149770 ) ) ;
#39293=CARTESIAN_POINT ( 'NONE',  ( 35.86761721751184240, -2.089954870031187628, 5.804407147029888137 ) ) ;
#39296=CARTESIAN_POINT ( 'NONE',  ( 30.71212904023629520, -2.930635124035476657, -4.999768531013319084 ) ) ;
#39299=CARTESIAN_POINT ( 'NONE',  ( 36.49335442002869456, -3.559127862921612984, 5.796824973035940687 ) ) ;
#39301=CARTESIAN_POINT ( 'NONE',  ( 33.45749450797183044, -3.829747548865578555, 5.093667367007288505 ) ) ;
#39303=CARTESIAN_POINT ( 'NONE',  ( 86.10475594078930328, 0.05610482897665627217, 5.990085204934172403 ) ) ;
#39305=EDGE_CURVE ( 'NONE', #22934, #36468, #1189, .T. ) ;
#39308=LINE ( 'NONE', #10899, #19446 ) ;
#39311=CARTESIAN_POINT ( 'NONE',  ( 23.41023413628745331, 3.546567081235476593, 3.496136802669740362 ) ) ;
#39318=CARTESIAN_POINT ( 'NONE',  ( 16.15328323628989082, -3.330670468083324565, -2.727508536291139762 ) ) ;
#39321=ORIENTED_EDGE ( 'NONE', *, *, #6084, .T. ) ;
#39322=CARTESIAN_POINT ( 'NONE',  ( 23.94801143228027840, 2.553151854112576835, -4.127014578414197388 ) ) ;
#39331=CARTESIAN_POINT ( 'NONE',  ( 87.79476240240137486, -0.2575195244695515639, -3.704994186184041194 ) ) ;
#39332=CARTESIAN_POINT ( 'NONE',  ( 29.60575365153160732, -0.8332953136462766253, 6.005451346670388268 ) ) ;
#39334=CARTESIAN_POINT ( 'NONE',  ( -75.69582718456990733, -3.730213777768353722, -10.20091118747310510 ) ) ;
#39335=CARTESIAN_POINT ( 'NONE',  ( 26.28311404583794086, -3.249458262315999768, 4.182437110436346472 ) ) ;
#39338=CARTESIAN_POINT ( 'NONE',  ( 34.38869957687920476, -1.330714714903810769, -5.573586281450729096 ) ) ;
#39341=EDGE_CURVE ( 'NONE', #10467, #29737, #22986, .T. ) ;
#39344=CARTESIAN_POINT ( 'NONE',  ( 27.67012909237472584, 1.632019845528506208, 4.348991244234835740 ) ) ;
#39349=VERTEX_POINT ( 'NONE', #19879 ) ;
#39357=ORIENTED_EDGE ( 'NONE', *, *, #24676, .T. ) ;
#39366=CARTESIAN_POINT ( 'NONE',  ( 25.40612371031801331, 0.6579664209402951158, 4.600295987165074152 ) ) ;
#39367=CARTESIAN_POINT ( 'NONE',  ( 14.73431651683273991, -4.754725209805407360, -2.504653360488686253 ) ) ;
#39373=CARTESIAN_POINT ( 'NONE',  ( 66.41194937274630661, -13.65448019739280028, 6.000000000000001776 ) ) ;
#39374=ORIENTED_EDGE ( 'NONE', *, *, #25078, .F. ) ;
#39375=CARTESIAN_POINT ( 'NONE',  ( 28.41236345070440805, -1.224654026667450157, -6.045523132457580218 ) ) ;
#39379=CARTESIAN_POINT ( 'NONE',  ( 26.75738543021116200, 0.8858420045314591151, -4.383008446193700003 ) ) ;
#39382=CARTESIAN_POINT ( 'NONE',  ( -71.67963774732312743, -48.41903106474732255, 9.972075897659857802 ) ) ;
#39383=CARTESIAN_POINT ( 'NONE',  ( 32.06786553091724556, 0.2506460099112566287, -4.730677192303592626 ) ) ;
#39392=CARTESIAN_POINT ( 'NONE',  ( 21.78485685878760947, 1.220823519683512437, -7.120777440962641869 ) ) ;
#39400=CARTESIAN_POINT ( 'NONE',  ( 87.87138265328074738, -2.102315541244656583, 2.954904511526853295 ) ) ;
#39410=ORIENTED_EDGE ( 'NONE', *, *, #25124, .F. ) ;
#39413=CARTESIAN_POINT ( 'NONE',  ( 17.53685894859813388, 11.96893683007039044, -2.499999999999995115 ) ) ;
#39420=CARTESIAN_POINT ( 'NONE',  ( 21.85643539959778892, 8.438975622634238505, -5.206363084432100052 ) ) ;
#39422=CARTESIAN_POINT ( 'NONE',  ( -76.45965604259320969, 10.62460191217738448, 8.333162867111299832 ) ) ;
#39423=CARTESIAN_POINT ( 'NONE',  ( 14.61823925964541004, -4.523600697705748352, 2.500000000000073275 ) ) ;
#39424=CARTESIAN_POINT ( 'NONE',  ( -78.52362145773746249, 11.36409002021383330, -6.517339437912577971 ) ) ;
#39426=CARTESIAN_POINT ( 'NONE',  ( 37.17733778849484594, -2.564252759210302823, -5.980908861731766279 ) ) ;
#39429=CARTESIAN_POINT ( 'NONE',  ( -62.92837670882106238, 10.37661300689600097, 6.000000000000000000 ) ) ;
#39431=DIRECTION ( 'NONE',  ( -0.000000000000000000, -0.000000000000000000, 1.000000000000000000 ) ) ;
#39434=CARTESIAN_POINT ( 'NONE',  ( 86.62098239308187431, 1.060925892958334060, 5.009353818272591852 ) ) ;
#39438=CARTESIAN_POINT ( 'NONE',  ( 35.89360613694101687, -2.027894626843364634, 5.808463346451208764 ) ) ;
#39442=CARTESIAN_POINT ( 'NONE',  ( 88.53816506398004549, -1.092544677973264378, 2.020403607635292254 ) ) ;
#39446=CARTESIAN_POINT ( 'NONE',  ( 4.588767459758324848E-15, -39.37473357531881391, -6.000000000000000000 ) ) ;
#39457=CARTESIAN_POINT ( 'NONE',  ( 23.94017511164331680, 1.184131663965027670, 4.939058140371498595 ) ) ;
#39465=FACE_OUTER_BOUND ( 'NONE', #27009, .T. ) ;
#39469=CARTESIAN_POINT ( 'NONE',  ( 23.69871966413117548, 3.485273507834210527, -3.367185970104320525 ) ) ;
#39473=CARTESIAN_POINT ( 'NONE',  ( 21.85643539959775694, 1.480681348264278219, 12.33944218828100325 ) ) ;
#39478=CARTESIAN_POINT ( 'NONE',  ( 86.19964454037233281, 1.163379821962233107, 5.771090254565081068 ) ) ;
#39483=CARTESIAN_POINT ( 'NONE',  ( 21.51740365705089530, -3.014515692509022404, -3.492477130908738570 ) ) ;
#39484=CARTESIAN_POINT ( 'NONE',  ( 25.29565861915397207, 1.734054340005127592, -4.154397323971344314 ) ) ;
#39486=CARTESIAN_POINT ( 'NONE',  ( 22.02701140547943837, 0.2674203034431413828, -7.573749491548535495 ) ) ;
#39488=CARTESIAN_POINT ( 'NONE',  ( 29.67411805608928077, -3.794755287726077064, -4.437710655330253218 ) ) ;
#39490=CARTESIAN_POINT ( 'NONE',  ( 34.13650501603236620, -3.129963852335855723, 5.534225220880571783 ) ) ;
#39497=CARTESIAN_POINT ( 'NONE',  ( 37.21233496738312851, -2.743626844932671727, 6.000895157570843352 ) ) ;
#39498=AXIS2_PLACEMENT_3D ( 'NONE', #32915, #35420, #29424 ) ;
#39500=CARTESIAN_POINT ( 'NONE',  ( 22.09538886637081134, -3.077477272664422614, -3.558916382092313757 ) ) ;
#39511=CARTESIAN_POINT ( 'NONE',  ( 14.73406068751933162, -4.758336531859351126, 2.504581428669218734 ) ) ;
#39516=CARTESIAN_POINT ( 'NONE',  ( 23.65346275343500437, 3.385680140419784934, 3.532840291856774062 ) ) ;
#39521=CARTESIAN_POINT ( 'NONE',  ( 22.14253154251144551, -2.652528785423459823, -3.662275584994673316 ) ) ;
#39524=CARTESIAN_POINT ( 'NONE',  ( 24.39390220926783570, 2.657251210456484269, -3.945702052070736432 ) ) ;
#39528=CARTESIAN_POINT ( 'NONE',  ( 20.26403867649277046, -7.228813795793931796, 2.500000000000000000 ) ) ;
#39534=CARTESIAN_POINT ( 'NONE',  ( 85.56690561042726983, 2.244914964738076613, -3.295588454431229497 ) ) ;
#39535=CARTESIAN_POINT ( 'NONE',  ( 33.89705139301766224, -5.463269898809035574, -0.9834710557593000502 ) ) ;
#39540=CARTESIAN_POINT ( 'NONE',  ( 35.78807231114511467, -3.222432190208943226, -5.791992240590498220 ) ) ;
#39544=DIRECTION ( 'NONE',  ( 1.000000000000000000, 1.385724075720358314E-16, -0.000000000000000000 ) ) ;
#39549=CARTESIAN_POINT ( 'NONE',  ( 25.69800855216902846, 2.595871837028679963, 3.649274041461021856 ) ) ;
#39552=CARTESIAN_POINT ( 'NONE',  ( -71.05894754566223526, 0.2170085631127749437, 10.00000000000003197 ) ) ;
#39554=ORIENTED_EDGE ( 'NONE', *, *, #29119, .T. ) ;
#39557=CARTESIAN_POINT ( 'NONE',  ( 85.39527935772777312, 1.303495358572782647, -5.575796090785288150 ) ) ;
#39564=CARTESIAN_POINT ( 'NONE',  ( 22.19187174190395240, 5.244396285582032746, 3.092647308070439305 ) ) ;
#39568=ORIENTED_EDGE ( 'NONE', *, *, #737, .T. ) ;
#39570=CARTESIAN_POINT ( 'NONE',  ( 22.59969544733755953, 0.2728855050143408900, 6.520465242868895395 ) ) ;
#39580=CARTESIAN_POINT ( 'NONE',  ( 87.04213330793392345, 0.5878691963682337596, 6.000000000000000000 ) ) ;
#39581=CARTESIAN_POINT ( 'NONE',  ( 29.75545004716739683, -3.157578436209982353, 4.923334784591472335 ) ) ;
#39585=CARTESIAN_POINT ( 'NONE',  ( -81.82390275669976631, -5.600668035901278152, 0.2449979024077967027 ) ) ;
#39586=CARTESIAN_POINT ( 'NONE',  ( 21.78199703343759452, 0.2105167186554868786, -8.406929788681917870 ) ) ;
#39587=EDGE_CURVE ( 'NONE', #29224, #23963, #14903, .T. ) ;
#39593=CARTESIAN_POINT ( 'NONE',  ( 36.71858516611970202, -3.456771977683057884, -5.861348970100675793 ) ) ;
#39596=CARTESIAN_POINT ( 'NONE',  ( -80.92837670882107659, 2.429809908903242555, -12.50000000000000000 ) ) ;
#39597=CARTESIAN_POINT ( 'NONE',  ( -71.31807670174137570, -48.56883691054113683, 5.988105119137681065 ) ) ;
#39601=CARTESIAN_POINT ( 'NONE',  ( 23.16133184106407583, 1.224392961250923229, -5.385929051048157667 ) ) ;
#39613=CARTESIAN_POINT ( 'NONE',  ( -4.890026461918809630, -25.50263309590217276, 2.500000000000000000 ) ) ;
#39617=CARTESIAN_POINT ( 'NONE',  ( 23.16657086568211099, -3.117828266824798966, 3.711575906808437075 ) ) ;
#39622=CARTESIAN_POINT ( 'NONE',  ( 16.55058197964011768, 7.675960740364504709, -3.484773916741207067 ) ) ;
#39627=DIRECTION ( 'NONE',  ( 0.000000000000000000, 0.000000000000000000, 1.000000000000000000 ) ) ;
#39628=CARTESIAN_POINT ( 'NONE',  ( 21.85643539959776760, -12.33099359671888884, 6.023794913588264244 ) ) ;
#39632=CARTESIAN_POINT ( 'NONE',  ( 14.78265019125518975, -5.167055302568825503, 2.499999999999999556 ) ) ;
#39634=CARTESIAN_POINT ( 'NONE',  ( -80.78529318222091149, 10.51041525961532663, -4.938515984036527584 ) ) ;
#39636=CARTESIAN_POINT ( 'NONE',  ( 30.67349724481533002, -3.593355625737403525, 4.777428303402127874 ) ) ;
#39649=CARTESIAN_POINT ( 'NONE',  ( 33.45622785515271147, -3.169918179184307849, 5.428051517361659251 ) ) ;
#39652=CARTESIAN_POINT ( 'NONE',  ( 88.61980888719223515, -1.376070350315937940, 2.940712392697649058 ) ) ;
#39665=CARTESIAN_POINT ( 'NONE',  ( 22.81843309643631201, 0.8035065468961524182, 5.971597756558487013 ) ) ;
#39677=CARTESIAN_POINT ( 'NONE',  ( 22.64349050896827009, 4.515835945530393580, -3.146491140164486833 ) ) ;
#39680=CARTESIAN_POINT ( 'NONE',  ( 21.85643539959777115, -1.513967970512005268, 12.69801924519992120 ) ) ;
#39685=CARTESIAN_POINT ( 'NONE',  ( 85.01740037914012760, 2.610285099004062470, -3.580537606963684283 ) ) ;
#39687=ORIENTED_EDGE ( 'NONE', *, *, #16571, .F. ) ;
#39690=CARTESIAN_POINT ( 'NONE',  ( 21.50588977098013999, -2.807818977413083950, -3.559126483975300292 ) ) ;
#39692=CARTESIAN_POINT ( 'NONE',  ( 22.91933720673384656, 2.648293172188526334, -3.783514896012181161 ) ) ;
#39694=CARTESIAN_POINT ( 'NONE',  ( 25.13440357308012807, 0.9923446184508544210, -4.613365629549119440 ) ) ;
#39697=CARTESIAN_POINT ( 'NONE',  ( 35.78603942060401977, -3.161145183569410211, 5.791674958855998590 ) ) ;
#39704=CARTESIAN_POINT ( 'NONE',  ( 36.87235869322262261, -2.085126334481405497, 5.863268595800801286 ) ) ;
#39708=ORIENTED_EDGE ( 'NONE', *, *, #39866, .T. ) ;
#39711=VERTEX_POINT ( 'NONE', #17323 ) ;
#39718=ORIENTED_EDGE ( 'NONE', *, *, #22009, .T. ) ;
#39723=CARTESIAN_POINT ( 'NONE',  ( 23.87861567317384015, 3.102426543664170033, 3.710302979149028957 ) ) ;
#39728=CARTESIAN_POINT ( 'NONE',  ( 21.85643539959776760, -15.11427361947482062, -2.500000000000000000 ) ) ;
#39732=CARTESIAN_POINT ( 'NONE',  ( 22.74486227573763841, 2.267316151577437822, -4.906501245702026281 ) ) ;
#39734=EDGE_CURVE ( 'NONE', #35457, #24696, #7074, .T. ) ;
#39743=CARTESIAN_POINT ( 'NONE',  ( 86.06238440510853138, 1.688369665709827272, 4.446988894268222303 ) ) ;
#39748=DIRECTION ( 'NONE',  ( 1.000000000000000000, 8.959828616340678715E-16, 0.000000000000000000 ) ) ;
#39749=LINE ( 'NONE', #6195, #14402 ) ;
#39751=CARTESIAN_POINT ( 'NONE',  ( 20.53310393597628192, 3.934805220908249801, -3.411085482841109240 ) ) ;
#39758=CARTESIAN_POINT ( 'NONE',  ( 34.14209189958793900, -3.845064354223240333, 5.237926034909554218 ) ) ;
#39762=ADVANCED_FACE ( 'NONE', ( #19835 ), #23131, .F. ) ;
#39763=DIRECTION ( 'NONE',  ( 1.000000000000000000, 0.000000000000000000, 0.000000000000000000 ) ) ;
#39768=CARTESIAN_POINT ( 'NONE',  ( 86.06519988977099445, 0.1302210779029090437, -5.995352467121073836 ) ) ;
#39775=CARTESIAN_POINT ( 'NONE',  ( 22.61643043036420053, 4.612325523533245430, 3.058534595953864343 ) ) ;
#39777=VECTOR ( 'NONE', #32258, 1000.000000000000000 ) ;
#39778=LINE ( 'NONE', #24331, #13010 ) ;
#39780=CARTESIAN_POINT ( 'NONE',  ( 24.75839165839662925, 3.019244830385916956, -3.350409272483306111 ) ) ;
#39784=CARTESIAN_POINT ( 'NONE',  ( 21.73396269091076860, 0.2160964541248809045, 9.105401517513902476 ) ) ;
#39785=CARTESIAN_POINT ( 'NONE',  ( 14.71768660209398583, -5.068519077135388073, -2.499999999999999556 ) ) ;
#39797=CARTESIAN_POINT ( 'NONE',  ( 29.86640044794213011, -3.433240980530400499, 4.572246828724481738 ) ) ;
#39798=DIRECTION ( 'NONE',  ( -1.000000000000000000, 0.000000000000000000, 0.000000000000000000 ) ) ;
#39800=EDGE_LOOP ( 'NONE', ( #28445, #21566, #7010, #27424 ) ) ;
#39802=CARTESIAN_POINT ( 'NONE',  ( 21.97057884596240740, 0.2201703367346467544, -7.735646635481312927 ) ) ;
#39808=DIRECTION ( 'NONE',  ( 0.000000000000000000, 0.000000000000000000, -1.000000000000000000 ) ) ;
#39809=CARTESIAN_POINT ( 'NONE',  ( 32.06722284780977361, 0.2495805760236646520, -4.732413161253986367 ) ) ;
#39814=CARTESIAN_POINT ( 'NONE',  ( -71.41359911753804113, -48.53977970579884982, 5.981042891625516056 ) ) ;
#39815=DIRECTION ( 'NONE',  ( -0.000000000000000000, -1.000000000000000000, -0.000000000000000000 ) ) ;
#39820=CARTESIAN_POINT ( 'NONE',  ( 23.04890016929587659, 1.973574480669345155, -4.925800778672301483 ) ) ;
#39821=CARTESIAN_POINT ( 'NONE',  ( -70.44203116010082510, -48.53935907511377934, 5.980943839742335122 ) ) ;
#39834=AXIS2_PLACEMENT_3D ( 'NONE', #14769, #30438, #11071 ) ;
#39844=DIRECTION ( 'NONE',  ( -0.000000000000000000, -0.000000000000000000, -1.000000000000000000 ) ) ;
#39846=CARTESIAN_POINT ( 'NONE',  ( 21.85643539959777115, 4.792808800112425160, -12.41435969090265523 ) ) ;
#39848=CARTESIAN_POINT ( 'NONE',  ( -81.24663647081587214, 10.50463385007281936, 3.730473497536808125 ) ) ;
#39849=CARTESIAN_POINT ( 'NONE',  ( 14.75140948485206316, -5.119342064155394390, 2.500052128446318189 ) ) ;
#39850=CARTESIAN_POINT ( 'NONE',  ( -74.31397190940765540, 7.087263004850651527, -10.69992065686621352 ) ) ;
#39854=CARTESIAN_POINT ( 'NONE',  ( 14.68017742504109613, 12.65464173479535859, 2.497594747247088520 ) ) ;
#39855=CARTESIAN_POINT ( 'NONE',  ( 14.61802081865033820, 0.000000000000000000, 3.500000000000000000 ) ) ;
#39858=CARTESIAN_POINT ( 'NONE',  ( 16.11725891507163766, 15.27317977277692052, -2.500000000000000000 ) ) ;
#39864=CARTESIAN_POINT ( 'NONE',  ( 20.42703419276611498, 3.672991389036573739, 3.394530734106728787 ) ) ;
#39866=EDGE_CURVE ( 'NONE', #12570, #28242, #4927, .T. ) ;
#39867=CARTESIAN_POINT ( 'NONE',  ( 87.00363285854439255, 0.09201467311058098009, -5.867932143725643535 ) ) ;
#39869=CARTESIAN_POINT ( 'NONE',  ( 86.37929632089314680, 1.332399160353644696, 5.153246707575002361 ) ) ;
#39877=CARTESIAN_POINT ( 'NONE',  ( 25.25995482075194332, 0.8517947254116883249, 4.614222942109635461 ) ) ;
#39880=EDGE_CURVE ( 'NONE', #18532, #561, #16618, .T. ) ;
#39891=CARTESIAN_POINT ( 'NONE',  ( 21.85746124272390034, 5.806209280568897846, -3.202049940849499343 ) ) ;
#39894=CARTESIAN_POINT ( 'NONE',  ( 25.50488203239457974, -4.522972804344248310, -2.044314315604920829 ) ) ;
#39898=CARTESIAN_POINT ( 'NONE',  ( 85.83023444425720072, 0.8841707150779518631, 5.891289308415252890 ) ) ;
#39899=CARTESIAN_POINT ( 'NONE',  ( 14.83041318099878048, 12.75128460074939163, 2.505930628224293244 ) ) ;
#39900=ORIENTED_EDGE ( 'NONE', *, *, #23741, .F. ) ;
#39903=CARTESIAN_POINT ( 'NONE',  ( 14.70827183493699231, -5.600023334934355113, -2.501374264973752926 ) ) ;
#39906=B_SPLINE_CURVE_WITH_KNOTS ( 'NONE', 3,
 ( #12977, #38086, #9888, #4722, #7605, #26357, #10883, #29441, #17659, #7803, #30241, #26156, #17256, #7995, #14375, #4534, #17057, #39488, #20759, #36026, #20355, #10682 ),
 .UNSPECIFIED., .F., .F.,
 ( 4, 2, 1, 1, 2, 2, 2, 1, 1, 1, 1, 2, 2, 4 ),
 ( 0.000000000000000000, 0.1249999999999835132, 0.1874999999999753253, 0.2187499999999711897, 0.2343749999999692191, 0.2499999999999672484, 0.3749999999999468758, 0.4374999999999369393, 0.4687499999999320544, 0.4843749999999263367, 0.4921874999999268918, 0.4960937499999268363, 0.4999999999999268363, 1.000000000000000000 ),
 .UNSPECIFIED. ) ;
#39908=ORIENTED_EDGE ( 'NONE', *, *, #2019, .T. ) ;
#39911=CARTESIAN_POINT ( 'NONE',  ( 87.00441857019603731, 0.6302321798448609069, -4.918210918608230564 ) ) ;
#39912=EDGE_LOOP ( 'NONE', ( #15230, #1644, #15610, #2606, #17868, #33418 ) ) ;
#39913=ORIENTED_EDGE ( 'NONE', *, *, #17819, .F. ) ;
#39915=CARTESIAN_POINT ( 'NONE',  ( 34.79255493759018947, -3.835798378834245348, 5.376544616508660113 ) ) ;
#39916=CARTESIAN_POINT ( 'NONE',  ( 22.13668169188128942, -2.652521926670949437, 3.661362574324665609 ) ) ;
#39917=CARTESIAN_POINT ( 'NONE',  ( 14.68065631944763716, 12.91438177319697012, -2.499999999999999556 ) ) ;
#39929=EDGE_LOOP ( 'NONE', ( #11606, #724, #3271, #31613 ) ) ;
#39930=CARTESIAN_POINT ( 'NONE',  ( 22.04812685758551183, 2.736502322861370740, 5.115368073871701782 ) ) ;
#39934=EDGE_CURVE ( 'NONE', #10017, #34818, #14143, .T. ) ;
#39942=CARTESIAN_POINT ( 'NONE',  ( 23.95477519611412376, 2.905619892612372190, -3.859501322721603511 ) ) ;
#39945=ORIENTED_EDGE ( 'NONE', *, *, #11883, .T. ) ;
#39948=CARTESIAN_POINT ( 'NONE',  ( 85.18642856628412119, 2.672284839249654542, -1.189885989438959069 ) ) ;
#39952=AXIS2_PLACEMENT_3D ( 'NONE', #28545, #28955, #38402 ) ;
#39957=CARTESIAN_POINT ( 'NONE',  ( 36.99319814093074399, -2.718620650874782108, -5.980081272406960302 ) ) ;
#39961=EDGE_CURVE ( 'NONE', #33153, #2897, #38212, .T. ) ;
#39965=CARTESIAN_POINT ( 'NONE',  ( 34.78606437710333665, -3.774923618171289519, 5.430246727453117650 ) ) ;
#39969=CARTESIAN_POINT ( 'NONE',  ( -70.92837670882107659, 13.87661300689600097, 0.000000000000000000 ) ) ;
#39973=CARTESIAN_POINT ( 'NONE',  ( -71.75720568778372410, 2.602768977313620002, -9.965624305424430673 ) ) ;
#39974=CARTESIAN_POINT ( 'NONE',  ( 15.58057500401926809, 10.76795092870248283, 2.638123565644369783 ) ) ;
#39976=ORIENTED_EDGE ( 'NONE', *, *, #9324, .T. ) ;
#39980=CARTESIAN_POINT ( 'NONE',  ( 23.42804606522540212, 3.768913320211875195, 3.161532174550911289 ) ) ;
#39983=LINE ( 'NONE', #24125, #262 ) ;
#39987=CARTESIAN_POINT ( 'NONE',  ( 26.75722929591961474, 0.8862554030004115013, 4.383001231454183966 ) ) ;
#39993=ORIENTED_EDGE ( 'NONE', *, *, #38755, .T. ) ;
#39995=DIRECTION ( 'NONE',  ( 0.7468947394616094471, 0.6649422893489137509, 0.000000000000000000 ) ) ;
#39998=CARTESIAN_POINT ( 'NONE',  ( 31.96905077431594933, -4.633974458378385286, -3.035954366531696369 ) ) ;
#39999=CARTESIAN_POINT ( 'NONE',  ( 14.61802081865033642, -4.461995682952384357, -2.500000000000000000 ) ) ;
#40001=CARTESIAN_POINT ( 'NONE',  ( -80.93496385967344509, -5.699872886623274404, -0.1912487157657831449 ) ) ;
#40002=CARTESIAN_POINT ( 'NONE',  ( 22.30956144702520660, 0.2684327122098100760, -7.077481357559062047 ) ) ;
#40007=CARTESIAN_POINT ( 'NONE',  ( 36.96506824942532177, -2.310990836009445548, -5.934258570784053610 ) ) ;
#40014=AXIS2_PLACEMENT_3D ( 'NONE', #130, #28727, #28932 ) ;
#40016=CARTESIAN_POINT ( 'NONE',  ( 22.26933136229914822, 1.666440873335421013, -5.843949089993668800 ) ) ;
#40019=CARTESIAN_POINT ( 'NONE',  ( 0.000000000000000000, 0.000000000000000000, 6.000000000000000000 ) ) ;
#40023=CARTESIAN_POINT ( 'NONE',  ( 85.08782340246310127, 1.754895396694989840, 5.093632142551737907 ) ) ;
#40031=ORIENTED_EDGE ( 'NONE', *, *, #13562, .F. ) ;
#40032=CARTESIAN_POINT ( 'NONE',  ( 22.18571586291277598, 5.278230443170779829, 3.067113879996727022 ) ) ;
#40033=EDGE_CURVE ( 'NONE', #29737, #12570, #27426, .T. ) ;
#40036=CARTESIAN_POINT ( 'NONE',  ( 16.10543327323123108, 10.11511941432178219, -2.500000000000563993 ) ) ;
#40040=CARTESIAN_POINT ( 'NONE',  ( 22.81955182245838643, 3.687635531278536050, 3.767940973477740485 ) ) ;
#40042=CARTESIAN_POINT ( 'NONE',  ( 22.45979449916501736, 0.3571986981647585768, -9.138524188866155029 ) ) ;
#40044=CARTESIAN_POINT ( 'NONE',  ( -79.86115014363866749, 11.51025212515079943, 4.513412623698347836 ) ) ;
#40045=LINE ( 'NONE', #2405, #20061 ) ;
#40046=EDGE_CURVE ( 'NONE', #13553, #36097, #22813, .T. ) ;
#40048=CARTESIAN_POINT ( 'NONE',  ( -73.50452121051399956, 5.643715073541963889, -9.720672664084132109 ) ) ;
#40053=CARTESIAN_POINT ( 'NONE',  ( 14.96508221674406336, 11.84948168787969180, 2.542061030440761815 ) ) ;
#40055=CARTESIAN_POINT ( 'NONE',  ( 29.58369257489212956, 0.1927579767638456509, 4.823648729257316248 ) ) ;
#40058=CARTESIAN_POINT ( 'NONE',  ( 87.34473703301738112, 0.2479703299153093454, 4.572837505533756897 ) ) ;
#40059=CARTESIAN_POINT ( 'NONE',  ( 26.66739313631886432, 1.596111124545895210, -4.344095840588632740 ) ) ;
#40062=CARTESIAN_POINT ( 'NONE',  ( 21.25554478757682730, 3.326128526321320500, 3.523839850031435628 ) ) ;
#40067=CARTESIAN_POINT ( 'NONE',  ( 87.79537149936930973, -0.4305974645707495441, -5.064761461465907999 ) ) ;
#40068=CARTESIAN_POINT ( 'NONE',  ( 33.87650332550894916, -5.319205609767368337, 2.014658837789633949 ) ) ;
#40089=CARTESIAN_POINT ( 'NONE',  ( 22.24686819720471931, 5.023333803137271403, -3.219619871319814752 ) ) ;
#40097=CARTESIAN_POINT ( 'NONE',  ( 84.80660115723814840, 2.320002077609508717, 4.142190259225312587 ) ) ;
#40098=CARTESIAN_POINT ( 'NONE',  ( 21.71182896267971074, 6.328908860361642574, -3.192117583127509928 ) ) ;
#40103=CARTESIAN_POINT ( 'NONE',  ( 86.00134810727946899, 0.2530519298808260320, -5.999722280616810899 ) ) ;
#40106=CARTESIAN_POINT ( 'NONE',  ( 28.88853511041031652, -3.138669953830422354, -4.706520689280823788 ) ) ;
#40111=CARTESIAN_POINT ( 'NONE',  ( 36.97894744516257504, -2.955629259446093116, 5.977857106677936905 ) ) ;
#40112=EDGE_CURVE ( 'NONE', #22420, #40359, #10958, .T. ) ;
#40114=CARTESIAN_POINT ( 'NONE',  ( 88.32659454254844889, -0.8548986265586405731, 1.105665148257566566 ) ) ;
#40118=CARTESIAN_POINT ( 'NONE',  ( 33.45699141876632865, -3.835191985160780526, 5.087378379710845167 ) ) ;
#40119=CARTESIAN_POINT ( 'NONE',  ( 24.40347370081251199, -3.150362192350396828, -3.888145324086332177 ) ) ;
#40129=CARTESIAN_POINT ( 'NONE',  ( 23.22046785484262799, 2.436457413438301689, 4.499336473899634647 ) ) ;
#40130=CARTESIAN_POINT ( 'NONE',  ( 21.24912046457389891, 8.714595741889111125, -2.623796381800369115 ) ) ;
#40131=ORIENTED_EDGE ( 'NONE', *, *, #33518, .F. ) ;
#40137=CARTESIAN_POINT ( 'NONE',  ( 85.20403636288057214, 2.652506926396006381, -1.368233707929553011 ) ) ;
#40140=CARTESIAN_POINT ( 'NONE',  ( 24.37218514414048798, 2.867522109304287525, -3.798528098029286593 ) ) ;
#40142=CARTESIAN_POINT ( 'NONE',  ( 21.85643539959780313, -10.31987362501297056, 12.61309593674697993 ) ) ;
#40144=ORIENTED_EDGE ( 'NONE', *, *, #26497, .T. ) ;
#40148=CARTESIAN_POINT ( 'NONE',  ( 87.78348876263190448, -0.2448564372010923473, 4.525229423219702340 ) ) ;
#40152=CARTESIAN_POINT ( 'NONE',  ( 33.96310664646391331, -3.802643679816640532, 5.242972732703274019 ) ) ;
#40155=CARTESIAN_POINT ( 'NONE',  ( 35.78609575529035425, -3.165688131210327771, -5.791683751246249123 ) ) ;
#40158=PLANE ( 'NONE',  #12513 ) ;
#40165=CARTESIAN_POINT ( 'NONE',  ( 37.13782911524162955, -2.596434994875571167, 5.986181626017550883 ) ) ;
#40169=CARTESIAN_POINT ( 'NONE',  ( -89.00859394718983708, 2.429809908903242555, 12.50000000000000000 ) ) ;
#40172=CARTESIAN_POINT ( 'NONE',  ( -74.40237796511935642, -4.238142967041890863, -9.381656193524049669 ) ) ;
#40174=PLANE ( 'NONE',  #29320 ) ;
#40175=CARTESIAN_POINT ( 'NONE',  ( 4.938390203311415748E-15, -42.37473357531882101, 2.500000000000000000 ) ) ;
#40177=CARTESIAN_POINT ( 'NONE',  ( 22.41328823501740786, 4.823693133274301381, 3.136477976532023870 ) ) ;
#40185=CARTESIAN_POINT ( 'NONE',  ( 14.72845434633629935, -4.936288270239374221, -2.501305200057243106 ) ) ;
#40189=ORIENTED_EDGE ( 'NONE', *, *, #32111, .F. ) ;
#40197=CARTESIAN_POINT ( 'NONE',  ( 33.19459970134796123, -3.309813850278316760, -5.543304389637502716 ) ) ;
#40205=CARTESIAN_POINT ( 'NONE',  ( 35.35501206519987960, -3.679878928346165701, -5.594686265449704266 ) ) ;
#40207=CARTESIAN_POINT ( 'NONE',  ( 86.00134810727946899, 0.2530519298808260320, -5.999722280616810899 ) ) ;
#40212=DIRECTION ( 'NONE',  ( 0.000000000000000000, -1.000000000000000000, 0.000000000000000000 ) ) ;
#40214=CARTESIAN_POINT ( 'NONE',  ( 21.82665949262245064, 2.023054712012288370, -6.063193687149706079 ) ) ;
#40217=ORIENTED_EDGE ( 'NONE', *, *, #27413, .F. ) ;
#40225=DIRECTION ( 'NONE',  ( 0.000000000000000000, 0.000000000000000000, 1.000000000000000000 ) ) ;
#40229=CARTESIAN_POINT ( 'NONE',  ( 22.87997942668749118, 4.340340381634286260, 3.050530276400981400 ) ) ;
#40234=CARTESIAN_POINT ( 'NONE',  ( 20.41154503683626942, 10.73873491509298006, -2.500000000000005773 ) ) ;
#40238=PLANE ( 'NONE',  #26739 ) ;
#40240=CARTESIAN_POINT ( 'NONE',  ( 21.85643539959776760, -10.46150609831112455, 5.349806725441734301 ) ) ;
#40242=CARTESIAN_POINT ( 'NONE',  ( -80.34441969748445445, 11.50396638009181238, 3.391339543253393707 ) ) ;
#40244=EDGE_CURVE ( 'NONE', #6636, #13553, #26761, .T. ) ;
#40245=CARTESIAN_POINT ( 'NONE',  ( -81.84931294303031279, 10.45753422446598790, -0.2086162088654086033 ) ) ;
#40246=CARTESIAN_POINT ( 'NONE',  ( 28.70188943284334471, -3.562248915020447715, -4.654001059522564709 ) ) ;
#40247=CARTESIAN_POINT ( 'NONE',  ( 36.71914689311213920, -3.458944023387923838, -5.860523124445346177 ) ) ;
#40249=CARTESIAN_POINT ( 'NONE',  ( 14.67067001192470066, 13.26205651873949520, 2.496110885492619502 ) ) ;
#40253=VECTOR ( 'NONE', #23074, 1000.000000000000000 ) ;
#40254=CARTESIAN_POINT ( 'NONE',  ( 17.30847559132336144, 14.31944607823880844, -2.500000000000000444 ) ) ;
#40255=CARTESIAN_POINT ( 'NONE',  ( 36.98394962418372245, -2.224080708393568973, -5.905313656129409061 ) ) ;
#40256=CARTESIAN_POINT ( 'NONE',  ( 25.71016244533634065, 2.120338955733263031, -4.148448561564090475 ) ) ;
#40261=CARTESIAN_POINT ( 'NONE',  ( 30.58586944111105055, 0.06670329603780118799, 4.980062666969890195 ) ) ;
#40264=CARTESIAN_POINT ( 'NONE',  ( 85.76120202873109122, 1.723374722402979620, 5.285180586055219898 ) ) ;
#40265=CARTESIAN_POINT ( 'NONE',  ( 33.51852797086635150, -3.949141208872448683, 4.993608438669980387 ) ) ;
#40266=CARTESIAN_POINT ( 'NONE',  ( 37.03125091814749936, -2.782549409756239545, -5.986020328601505902 ) ) ;
#40269=DIRECTION ( 'NONE',  ( 0.000000000000000000, -0.000000000000000000, -1.000000000000000000 ) ) ;
#40271=ORIENTED_EDGE ( 'NONE', *, *, #36241, .T. ) ;
#40273=EDGE_CURVE ( 'NONE', #1813, #5958, #11035, .T. ) ;
#40287=EDGE_CURVE ( 'NONE', #36231, #11923, #5084, .T. ) ;
#40288=PLANE ( 'NONE',  #20880 ) ;
#40289=CARTESIAN_POINT ( 'NONE',  ( 23.71667221069719744, 3.517694658488856430, -3.297412223443493495 ) ) ;
#40296=CARTESIAN_POINT ( 'NONE',  ( 88.11323260317807637, -2.391772166421624490, 1.226420884133070599 ) ) ;
#40301=AXIS2_PLACEMENT_3D ( 'NONE', #19495, #4066, #10417 ) ;
#40304=CARTESIAN_POINT ( 'NONE',  ( 21.25143292528058225, 3.315796426267975328, -3.523198094474456532 ) ) ;
#40305=CARTESIAN_POINT ( 'NONE',  ( -70.92837670882107659, -23.80776546975053165, 6.000000000000002665 ) ) ;
#40307=CARTESIAN_POINT ( 'NONE',  ( 31.71768278297239263, -0.5622167780584130803, 5.156709511976435678 ) ) ;
#40313=CARTESIAN_POINT ( 'NONE',  ( 37.10477226148266539, -3.126860894810321145, 5.976159207400391971 ) ) ;
#40314=CARTESIAN_POINT ( 'NONE',  ( 26.94740486763593523, -2.794811601311201876, 4.412192273680850541 ) ) ;
#40315=CARTESIAN_POINT ( 'NONE',  ( 22.11758564014485628, -3.078173236878668284, -3.562082636516995304 ) ) ;
#40316=B_SPLINE_CURVE_WITH_KNOTS ( 'NONE', 3,
 ( #36170, #27908, #27705, #5277, #8756, #33247, #1966, #30358, #27057, #39821, #33661, #5438, #23497, #14417 ),
 .UNSPECIFIED., .F., .F.,
 ( 4, 2, 2, 2, 2, 2, 4 ),
 ( 0.007062463343506314266, 0.007356602418556547340, 0.007650741493606780415, 0.008239019643707230084, 0.008827297793807680620, 0.009121436868857905889, 0.009415575943908131157 ),
 .UNSPECIFIED. ) ;
#40320=ORIENTED_EDGE ( 'NONE', *, *, #24928, .F. ) ;
#40322=CARTESIAN_POINT ( 'NONE',  ( 14.76639648210999667, -4.521389705567960604, 2.511021882340067179 ) ) ;
#40323=CARTESIAN_POINT ( 'NONE',  ( 23.31153495202840631, 2.940644873606350185, 4.073321330939048579 ) ) ;
#40324=CARTESIAN_POINT ( 'NONE',  ( 29.33427167545534431, 1.276824085243427165, 4.194055504906347487 ) ) ;
#40325=ORIENTED_EDGE ( 'NONE', *, *, #11768, .T. ) ;
#40329=EDGE_CURVE ( 'NONE', #17714, #12496, #33926, .T. ) ;
#40334=DIRECTION ( 'NONE',  ( -0.000000000000000000, -0.000000000000000000, -1.000000000000000000 ) ) ;
#40337=CARTESIAN_POINT ( 'NONE',  ( 23.04763360661103988, 3.226630789359916651, -3.993616397825694442 ) ) ;
#40338=ORIENTED_EDGE ( 'NONE', *, *, #6414, .F. ) ;
#40341=CARTESIAN_POINT ( 'NONE',  ( 21.85643539959773207, -10.94848525941816675, -12.02078412262589602 ) ) ;
#40345=CARTESIAN_POINT ( 'NONE',  ( 88.57583237253618336, -1.134854386742023546, -1.768762308819206375 ) ) ;
#40346=CARTESIAN_POINT ( 'NONE',  ( 30.30396332325029718, -0.06004591992995000210, 5.542382567169830132 ) ) ;
#40348=CARTESIAN_POINT ( 'NONE',  ( 16.24913492685886851, -3.406803814618201365, 2.736837790127818248 ) ) ;
#40350=CARTESIAN_POINT ( 'NONE',  ( 27.44843548912706765, 1.080599773242067574, -4.490390219635936653 ) ) ;
#40357=VECTOR ( 'NONE', #559, 1000.000000000000000 ) ;
#40359=VERTEX_POINT ( 'NONE', #33710 ) ;
#40360=CARTESIAN_POINT ( 'NONE',  ( 33.08016986529464276, -0.2095144213782778597, 5.024908790581100959 ) ) ;
#40364=CARTESIAN_POINT ( 'NONE',  ( -71.81436415662651029, 1.349290789225021436, -9.960713035918328018 ) ) ;
#40370=CARTESIAN_POINT ( 'NONE',  ( 23.14177627322540687, 4.014150865615426333, 3.136148348386343709 ) ) ;
#40374=CARTESIAN_POINT ( 'NONE',  ( 21.71182896267971074, 6.328908860361642574, -3.192117583127509928 ) ) ;
#40375=ORIENTED_EDGE ( 'NONE', *, *, #27284, .T. ) ;
#40393=CARTESIAN_POINT ( 'NONE',  ( 28.89923929355584065, 0.07307017450661948410, 5.719397691353443669 ) ) ;
#40397=CARTESIAN_POINT ( 'NONE',  ( 22.62891770203226471, 0.3003589381232597000, -6.476356472173973700 ) ) ;
#40402=CARTESIAN_POINT ( 'NONE',  ( 36.48442795868031396, -3.515690391850441632, -5.817181155477498145 ) ) ;
#40403=DIRECTION ( 'NONE',  ( 1.000000000000000000, 0.000000000000000000, -0.000000000000000000 ) ) ;
#40410=CARTESIAN_POINT ( 'NONE',  ( 22.02569479573740452, 1.683627192489213442, -6.127589934087004586 ) ) ;
#40421=CARTESIAN_POINT ( 'NONE',  ( 22.88100581559600144, 4.343313832157520871, 3.044019733130736594 ) ) ;
#40428=ORIENTED_EDGE ( 'NONE', *, *, #11831, .T. ) ;
#40432=LINE ( 'NONE', #19044, #36043 ) ;
#40433=CARTESIAN_POINT ( 'NONE',  ( 22.77977322753350720, -5.661609348961630594, -5.678499401198807917 ) ) ;
#40435=CARTESIAN_POINT ( 'NONE',  ( -74.80457647086952022, 7.715846600713136105, 10.55247600905316574 ) ) ;
#40436=CARTESIAN_POINT ( 'NONE',  ( 37.05408364730916304, -3.185536086795005328, 5.961296328585691029 ) ) ;
#40441=CARTESIAN_POINT ( 'NONE',  ( 34.63837955954176095, -0.7796828013290140191, -5.272681140724467141 ) ) ;
#40443=CARTESIAN_POINT ( 'NONE',  ( 14.92554660196259775, 12.09598766256684499, 2.535890541581709456 ) ) ;
#40445=CARTESIAN_POINT ( 'NONE',  ( 29.66023932424631226, -3.797131443868001721, 4.433517098046177551 ) ) ;
#40448=CARTESIAN_POINT ( 'NONE',  ( 23.62484588740604607, 0.5005666067537509756, -5.479226438200067051 ) ) ;
#40449=CARTESIAN_POINT ( 'NONE',  ( 36.83628562539227858, -2.061009687061731377, -5.854267444441933144 ) ) ;
#40450=CARTESIAN_POINT ( 'NONE',  ( 24.72034790271620963, 2.638369506531949682, -3.924384734724444712 ) ) ;
#40453=CARTESIAN_POINT ( 'NONE',  ( 36.94807309570725096, -2.593677492714873800, 5.973038417746441731 ) ) ;
#40454=EDGE_CURVE ( 'NONE', #15393, #16288, #24515, .T. ) ;
#40458=AXIS2_PLACEMENT_3D ( 'NONE', #802, #10845, #7766 ) ;
#40459=CARTESIAN_POINT ( 'NONE',  ( 87.33013056844055200, 0.1115698105147486796, -5.569409363020906056 ) ) ;
#40460=CARTESIAN_POINT ( 'NONE',  ( 29.43591252028664584, 1.494051637964393553, 3.776330930280134002 ) ) ;
#40461=CARTESIAN_POINT ( 'NONE',  ( 35.96180494042192066, -3.155136263811515018, -5.819107419128717318 ) ) ;
#40463=CARTESIAN_POINT ( 'NONE',  ( 24.34570196473333681, 2.899197553801855065, 3.775102329553754021 ) ) ;
#40466=ORIENTED_EDGE ( 'NONE', *, *, #18053, .F. ) ;
#40468=EDGE_CURVE ( 'NONE', #32120, #16957, #474, .T. ) ;
#40477=B_SPLINE_CURVE_WITH_KNOTS ( 'NONE', 3,
 ( #27208, #27011, #39149, #14240, #23322, #39768, #26814, #20220, #36092, #17121, #17931, #7668 ),
 .UNSPECIFIED., .F., .F.,
 ( 4, 2, 1, 1, 2, 2, 4 ),
 ( 0.9809184011985524476, 0.9815147011610976246, 0.9821110011236428017, 0.9833036010487331557, 0.9856888008989141969, 0.9904592005992760573, 1.000000000000000000 ),
 .UNSPECIFIED. ) ;
#40479=FACE_OUTER_BOUND ( 'NONE', #32762, .T. ) ;
#40482=CARTESIAN_POINT ( 'NONE',  ( 22.90896498715502005, 4.192648223596282975, -3.220349011596035815 ) ) ;
#40484=CARTESIAN_POINT ( 'NONE',  ( 25.50874925706157725, -4.568791516319697266, 1.869930813790659618 ) ) ;
#40486=CARTESIAN_POINT ( 'NONE',  ( -77.50117670466831044, -4.927849438259591430, -7.545501454821059717 ) ) ;
#40489=CARTESIAN_POINT ( 'NONE',  ( 86.75210013534866960, -0.2795847087395720298, -5.842668109216860195 ) ) ;
#40490=( BOUNDED_CURVE ( )  B_SPLINE_CURVE ( 3, ( #11580, #30554, #24570, #40207 ),
 .UNSPECIFIED., .F., .T. ) 
 B_SPLINE_CURVE_WITH_KNOTS ( ( 4, 4 ),
 ( 0.3200567940537017431, 0.9849192321825703811 ),
 .UNSPECIFIED. ) 
 CURVE ( )  GEOMETRIC_REPRESENTATION_ITEM ( )  RATIONAL_B_SPLINE_CURVE ( ( 0.9715283094173854384, 0.9610933789717652775, 0.9699361791336866823, 0.9980567099031494305 ) ) 
 REPRESENTATION_ITEM ( '' )  );
#40491=CARTESIAN_POINT ( 'NONE',  ( 18.96867664023077893, 7.708620133838740784, 3.077328312083026152 ) ) ;
#40494=CARTESIAN_POINT ( 'NONE',  ( -72.22997424438122493, -46.36506344532806168, 9.915082283677739028 ) ) ;
#40495=VECTOR ( 'NONE', #29120, 1000.000000000000000 ) ;
#40496=EDGE_CURVE ( 'NONE', #5343, #8047, #7718, .T. ) ;
#40502=CARTESIAN_POINT ( 'NONE',  ( 36.89707210798169257, -3.001693912205876114, 5.965078480148344298 ) ) ;
#40503=B_SPLINE_CURVE_WITH_KNOTS ( 'NONE', 3,
 ( #31696, #26474, #1179, #23179, #23378, #23582, #35946, #38609, #32662, #10413, #36146, #26279, #7728, #22989, #33057, #32860, #4844, #7324, #26674, #35555, #19883, #38812, #10606 ),
 .UNSPECIFIED., .F., .F.,
 ( 4, 2, 2, 2, 1, 2, 2, 2, 2, 2, 2, 4 ),
 ( 0.06733963574726689605, 0.1651538230393540529, 0.2140609166853975620, 0.2385144635084192888, 0.2446278502141747135, 0.2476845435670523843, 0.2507412369199301105, 0.2629680103314415152, 0.3607821976235333628, 0.3852357444465562830, 0.4096892912695793143, 0.4585963849156251548 ),
 .UNSPECIFIED. ) ;
#40505=CARTESIAN_POINT ( 'NONE',  ( 86.69860591627480062, 0.9737354674733970095, 5.003702464200671329 ) ) ;
#40518=ORIENTED_EDGE ( 'NONE', *, *, #40329, .F. ) ;
#40523=ORIENTED_EDGE ( 'NONE', *, *, #25014, .T. ) ;
#40524=CARTESIAN_POINT ( 'NONE',  ( 23.34681557898295168, 2.817057717204138445, 4.150130206757231655 ) ) ;
#40525=CARTESIAN_POINT ( 'NONE',  ( 32.56727300831884264, 0.05559756199407518001, 4.835980446979140090 ) ) ;
#40526=ORIENTED_EDGE ( 'NONE', *, *, #27284, .F. ) ;
#40531=CARTESIAN_POINT ( 'NONE',  ( -70.12833371007830863, -0.1687847323711494374, 5.947160319466099132 ) ) ;
#40532=CARTESIAN_POINT ( 'NONE',  ( 86.14290222033510247, 1.597928234041334106, -4.557262599208225851 ) ) ;
#40536=CARTESIAN_POINT ( 'NONE',  ( 24.15427200232377913, 2.904266593399515983, -3.806858982482544729 ) ) ;
#40538=CARTESIAN_POINT ( 'NONE',  ( 21.85643539959776760, 7.606201961588627825, -9.696886732879795190 ) ) ;
#40539=CARTESIAN_POINT ( 'NONE',  ( 16.14595902796557425, 15.25073734555082794, 3.865347545245052701E-13 ) ) ;
#40543=CARTESIAN_POINT ( 'NONE',  ( 87.10491796770416784, 0.5173464865745804886, -5.275911943831619766 ) ) ;
#40544=EDGE_LOOP ( 'NONE', ( #178, #17345, #22800, #34360 ) ) ;
#40546=CARTESIAN_POINT ( 'NONE',  ( 28.89384288918207844, -3.006948380915847263, 4.715981001724134813 ) ) ;
#40549=CARTESIAN_POINT ( 'NONE',  ( 36.99353526044117046, -2.718331692064833494, -5.980133888059827818 ) ) ;
#40560=EDGE_LOOP ( 'NONE', ( #22241, #7310, #9497, #2486, #25837 ) ) ;
#40561=CARTESIAN_POINT ( 'NONE',  ( 37.21137251006081215, -2.743940103560390753, 6.000897398658226578 ) ) ;
#40569=CARTESIAN_POINT ( 'NONE',  ( -74.69374601795452406, -4.520613029625567769, -9.269913512513538123 ) ) ;
#40576=CARTESIAN_POINT ( 'NONE',  ( 22.89285562436331745, 4.257133708064684718, 3.156151907905176746 ) ) ;
#40582=CARTESIAN_POINT ( 'NONE',  ( 14.81709837128977014, 12.80649608571206599, -2.504134368729534543 ) ) ;
#40583=B_SPLINE_CURVE_WITH_KNOTS ( 'NONE', 3,
 ( #2002, #33078, #14717, #17396, #7748, #24203, #26890, #30394, #20297, #5475 ),
 .UNSPECIFIED., .F., .F.,
 ( 4, 2, 2, 2, 4 ),
 ( 0.001564566806966613197, 0.001955354412007498290, 0.002346142017048383384, 0.002736929622089268477, 0.003127717227130153571 ),
 .UNSPECIFIED. ) ;
#40586=CARTESIAN_POINT ( 'NONE',  ( 17.61407464359234609, 8.411925271401869963, -2.955500364774379385 ) ) ;
#40589=CARTESIAN_POINT ( 'NONE',  ( -4.224659823956008253, -51.67615071827237472, 2.500000000000000000 ) ) ;
#40593=VECTOR ( 'NONE', #11640, 1000.000000000000000 ) ;
#40594=CARTESIAN_POINT ( 'NONE',  ( 0.6783104270758654186, -48.60743831809499227, -6.000000000000000000 ) ) ;
#40599=CARTESIAN_POINT ( 'NONE',  ( 31.86155337613836380, -4.142523116122148963, 4.178567150506776962 ) ) ;
#40603=CARTESIAN_POINT ( 'NONE',  ( 22.32588140555700917, 0.2761883842276166012, -7.044564668695222132 ) ) ;
#40606=LINE ( 'NONE', #12412, #36232 ) ;
#40608=CYLINDRICAL_SURFACE ( 'NONE', #8492, 2.500000000000000444 ) ;
#40610=CARTESIAN_POINT ( 'NONE',  ( 34.13092259911290682, -3.728237912347327043, -5.351359701968583238 ) ) ;
#40612=CARTESIAN_POINT ( 'NONE',  ( 32.73787262251559582, -3.800317724956558063, 4.944879674104074141 ) ) ;
#40618=CARTESIAN_POINT ( 'NONE',  ( 87.09859342968812257, 0.5244505078549105415, -5.068689133590885909 ) ) ;
#40620=CARTESIAN_POINT ( 'NONE',  ( 14.77222177532591196, -4.492696128702778680, -2.511960494210057959 ) ) ;
#40623=VERTEX_POINT ( 'NONE', #36139 ) ;
#40629=EDGE_CURVE ( 'NONE', #21561, #40359, #22280, .T. ) ;
#40634=ORIENTED_EDGE ( 'NONE', *, *, #12178, .F. ) ;
#40635=CARTESIAN_POINT ( 'NONE',  ( 24.77632181662465172, 3.027756120316424049, 3.312394854541005795 ) ) ;
#40640=CARTESIAN_POINT ( 'NONE',  ( 22.02793885145894492, 0.2684150387854475905, 7.571002712326798445 ) ) ;
#40647=B_SPLINE_CURVE_WITH_KNOTS ( 'NONE', 3,
 ( #19185, #5816, #34658, #6225, #34043, #21671, #255, #12591, #31751, #31344, #28447, #3563, #16093, #18770, #62, #25158 ),
 .UNSPECIFIED., .F., .F.,
 ( 4, 2, 2, 2, 2, 2, 2, 4 ),
 ( 0.002354838921902799483, 0.002649036855363638438, 0.002943234788824477394, 0.003531630655746170917, 0.003825828589206996862, 0.004120026522667821940, 0.004414224456128647452, 0.004708422389589472963 ),
 .UNSPECIFIED. ) ;
#40649=CARTESIAN_POINT ( 'NONE',  ( 21.85643539959778181, 1.552649203755968488, -12.31912549844641447 ) ) ;
#40651=VERTEX_POINT ( 'NONE', #34850 ) ;
#40652=CARTESIAN_POINT ( 'NONE',  ( -72.84122331582933896, 2.640701540777562251, 10.96218028030935443 ) ) ;
#40653=CARTESIAN_POINT ( 'NONE',  ( 37.09188196241630209, -3.135874510096115841, 5.972645679324628532 ) ) ;
#40659=CARTESIAN_POINT ( 'NONE',  ( 36.68588390344509520, -1.914239285580463745, -5.802834115057662778 ) ) ;
#40661=CARTESIAN_POINT ( 'NONE',  ( 14.77291369034715096, 13.25847280940105932, 2.500173083280071040 ) ) ;
#40662=CARTESIAN_POINT ( 'NONE',  ( -17.27251170661583402, -8.656638842136340273, -2.500000000000000000 ) ) ;
#40666=CARTESIAN_POINT ( 'NONE',  ( 24.10540974869017461, 0.6288044972621918971, -5.083578459613002032 ) ) ;
#40669=CARTESIAN_POINT ( 'NONE',  ( 24.36315553053532312, 2.932691449427110353, -3.734387699189308130 ) ) ;
#40670=VERTEX_POINT ( 'NONE', #6419 ) ;
#40672=CARTESIAN_POINT ( 'NONE',  ( 36.83721040901404820, -2.495908143111605249, 5.955735614263799604 ) ) ;
#40677=ADVANCED_FACE ( 'NONE', ( #13195, #16480 ), #3361, .T. ) ;
#40678=CARTESIAN_POINT ( 'NONE',  ( 36.08735695191136017, -2.181264466747378616, -5.838702847008515384 ) ) ;
#40682=PLANE ( 'NONE',  #31079 ) ;
#40686=VERTEX_POINT ( 'NONE', #38300 ) ;
#40696=CARTESIAN_POINT ( 'NONE',  ( 23.71023650492422163, -7.011372125143266132, 2.558830977042959365 ) ) ;
#40699=CARTESIAN_POINT ( 'NONE',  ( 21.83674782184219509, 5.925148072649942144, -3.152431264756139662 ) ) ;
#40702=CARTESIAN_POINT ( 'NONE',  ( 24.19350110911862828, 1.223952504169800948, -6.554579921768042716 ) ) ;
#40703=CARTESIAN_POINT ( 'NONE',  ( -76.47802091883025355, -4.341682083958475324, -8.338848444810246008 ) ) ;
#40706=CARTESIAN_POINT ( 'NONE',  ( 84.61114100273776728, 2.563204847888557403, 3.486439758113726306 ) ) ;
#40707=CARTESIAN_POINT ( 'NONE',  ( 15.61612061779542060, 11.17844057676542846, 2.610974633258779765 ) ) ;
#40710=DIRECTION ( 'NONE',  ( -0.000000000000000000, -0.000000000000000000, -1.000000000000000000 ) ) ;
#40711=VECTOR ( 'NONE', #11728, 1000.000000000000000 ) ;
#40717=CARTESIAN_POINT ( 'NONE',  ( 85.57827979132923701, 1.010891326585220629, 5.785350395857181915 ) ) ;
#40718=CARTESIAN_POINT ( 'NONE',  ( 36.97917538118862524, -2.955947328860137002, 5.977892681607455572 ) ) ;
#40732=COLOUR_RGB('Dark Blue',0.08,0.2,0.34);
#40733=FILL_AREA_STYLE_COLOUR('',#40732);
#40734=FILL_AREA_STYLE('',(#40733));
#40735=SURFACE_STYLE_FILL_AREA(#40734);
#40736=SURFACE_SIDE_STYLE('',(#40735));
#40737=SURFACE_STYLE_USAGE(.BOTH.,#40736);
#40738=PRESENTATION_STYLE_ASSIGNMENT((#40737));
ENDSEC;
END-ISO-10303-21;
